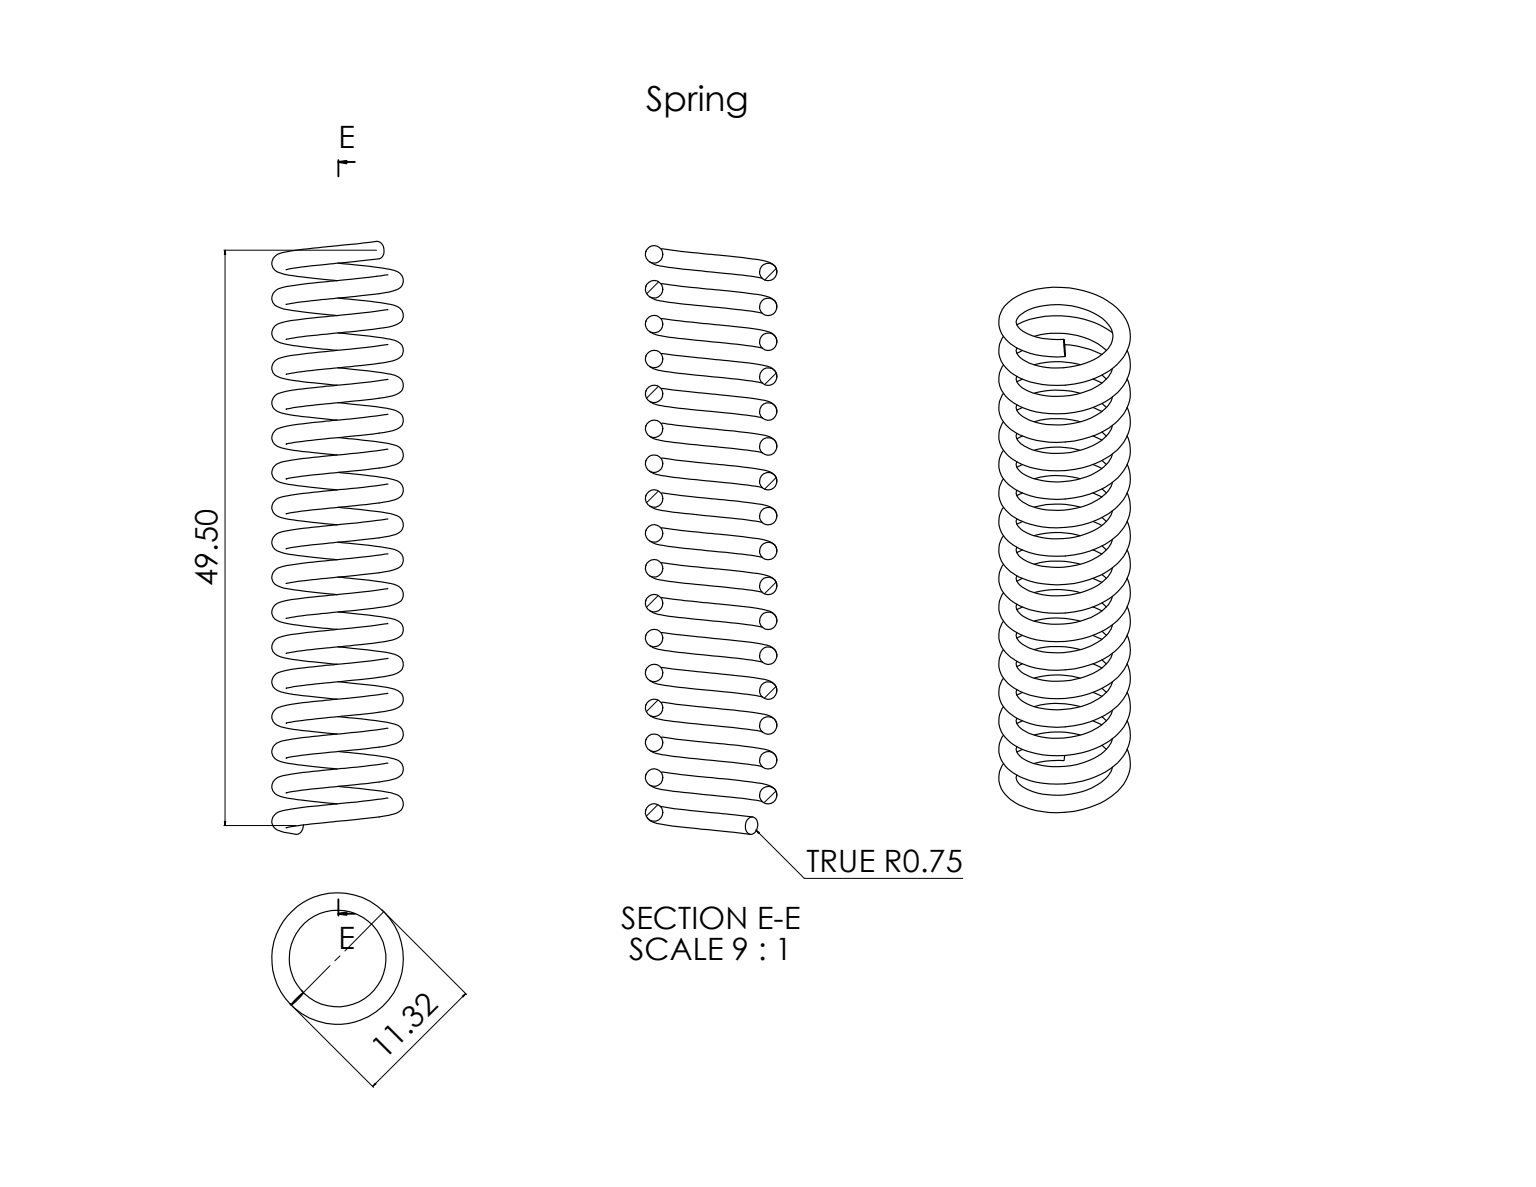
ISO-10303-21;
HEADER;
FILE_DESCRIPTION (('STEP AP214'),
    '1' );
FILE_NAME ('Spring.step',
    '2026-10-25T21:42:00',
    ( '' ),
    ( '' ),
    'SwSTEP 2.0',
    'SolidWorks 2025',
    '' );
FILE_SCHEMA (( 'AUTOMOTIVE_DESIGN' ));
ENDSEC;

DATA;
#8=CARTESIAN_POINT ( 'NONE',  ( 2.564989113914249330, 22.87042866830903876, -37.34295307432606137 ) ) ;
#27=CARTESIAN_POINT ( 'NONE',  ( -3.895814058185739448, 15.51498359085620571, -28.64999999999995950 ) ) ;
#28=CARTESIAN_POINT ( 'NONE',  ( 0.6839900399647733664, 13.18145684914961357, -55.04999999999995453 ) ) ;
#40=CARTESIAN_POINT ( 'NONE',  ( -4.099003336600151925, 21.81495595370741469, -69.75704692567386189 ) ) ;
#41=CARTESIAN_POINT ( 'NONE',  ( -0.8851648821498765418, 11.91128888458923285, -58.19999999999996732 ) ) ;
#52=CARTESIAN_POINT ( 'NONE',  ( 5.852430833189966819, 16.41846101382252243, -49.95704692567387184 ) ) ;
#56=CARTESIAN_POINT ( 'NONE',  ( 3.898383833589191383, 21.60376697729997275, -70.49295307432603863 ) ) ;
#72=CARTESIAN_POINT ( 'NONE',  ( 5.041649132594343996, 14.93115145952162415, -45.59999999999996589 ) ) ;
#75=CARTESIAN_POINT ( 'NONE',  ( 4.129897239856814117, 18.00707336630801336, -58.80704692567387326 ) ) ;
#76=CARTESIAN_POINT ( 'NONE',  ( 1.985016409143818272, 21.39581405818570659, -50.84999999999996589 ) ) ;
#85=CARTESIAN_POINT ( 'NONE',  ( 4.107178604518054499, 18.15051318458946383, -60.29999999999996163 ) ) ;
#87=CARTESIAN_POINT ( 'NONE',  ( 3.043106805520193525, 20.33772366180932067, -46.50704692567387610 ) ) ;
#91=CARTESIAN_POINT ( 'NONE',  ( -4.342430937695320736, 18.03316848959025620, -36.44295307432606279 ) ) ;
#106=CARTESIAN_POINT ( 'NONE',  ( -0.8851648821498765418, 11.91128888458923285, -49.19999999999996732 ) ) ;
#122=CARTESIAN_POINT ( 'NONE',  ( -5.876318620034919782, 18.43071743580290089, -67.94999999999994600 ) ) ;
#127=CARTESIAN_POINT ( 'NONE',  ( 4.107178604518054499, 18.15051318458946383, -42.29999999999996874 ) ) ;
#138=CARTESIAN_POINT ( 'NONE',  ( -3.826489000663265472, 15.37892550466785480, -51.14295307432606563 ) ) ;
#154=CARTESIAN_POINT ( 'NONE',  ( 4.107178604518054499, 18.15051318458946383, -33.29999999999996874 ) ) ;
#181=CARTESIAN_POINT ( 'NONE',  ( 3.965139115708213868, 19.34895832295540430, -37.65704692567386758 ) ) ;
#186=CARTESIAN_POINT ( 'NONE',  ( 4.314955953707388936, 13.40099666339979123, -38.24295307432604574 ) ) ;
#187=CARTESIAN_POINT ( 'NONE',  ( -3.705139346311794313, 19.38786279086902198, -26.09999999999996234 ) ) ;
#193=CARTESIAN_POINT ( 'NONE',  ( -1.887862790868997553, 21.20513934631180319, -44.39999999999997016 ) ) ;
#196=CARTESIAN_POINT ( 'NONE',  ( -1.028604700431329233, 11.93400751992799513, -41.70704692567387184 ) ) ;
#198=CARTESIAN_POINT ( 'NONE',  ( 3.705139346311793869, 15.61213720913094960, -63.59999999999995879 ) ) ;
#211=CARTESIAN_POINT ( 'NONE',  ( -0.7417250638684240727, 11.88857024925047057, -35.69295307432606279 ) ) ;
#233=CARTESIAN_POINT ( 'NONE',  ( 3.091735541773220852, 14.40826445822673563, -57.74999999999995737 ) ) ;
#243=CARTESIAN_POINT ( 'NONE',  ( -1.028604700431329233, 11.93400751992799513, -68.70704692567387895 ) ) ;
#244=CARTESIAN_POINT ( 'NONE',  ( 5.301103610786608300, 20.20104720010254340, -60.14999999999996305 ) ) ;
#258=CARTESIAN_POINT ( 'NONE',  ( -4.099003336600151925, 21.81495595370741469, -48.75704692567386189 ) ) ;
#264=CARTESIAN_POINT ( 'NONE',  ( -2.698247469942396837, 22.47571708489507358, -63.89295307432605853 ) ) ;
#279=CARTESIAN_POINT ( 'NONE',  ( -5.588711115410763597, 16.61483511785016987, -43.79999999999996163 ) ) ;
#282=CARTESIAN_POINT ( 'NONE',  ( -4.129897239856814117, 16.99292663369196177, -48.30704692567388037 ) ) ;
#284=CARTESIAN_POINT ( 'NONE',  ( -1.985016409143819605, 13.60418594181426855, -52.34999999999995879 ) ) ;
#294=CARTESIAN_POINT ( 'NONE',  ( 2.940415233664778416, 20.44041523366473712, -59.99999999999997158 ) ) ;
#297=CARTESIAN_POINT ( 'NONE',  ( -0.7939530028709754772, 13.41554003082070246, -47.70704692567387184 ) ) ;
#301=CARTESIAN_POINT ( 'NONE',  ( 2.017261720333081598, 13.86079270138745834, -35.39295307432605142 ) ) ;
#307=CARTESIAN_POINT ( 'NONE',  ( 3.965139115708213868, 19.34895832295540430, -28.65704692567387468 ) ) ;
#316=CARTESIAN_POINT ( 'NONE',  ( 2.701047200102605572, 22.80110361078655856, -44.84999999999996589 ) ) ;
#332=CARTESIAN_POINT ( 'NONE',  ( -2.701047200102606016, 12.19889638921340413, -70.34999999999993747 ) ) ;
#337=CARTESIAN_POINT ( 'NONE',  ( 3.895814058185739448, 19.48501640914375344, -45.14999999999994884 ) ) ;
#351=CARTESIAN_POINT ( 'NONE',  ( -0.5070733663080690956, 13.37010276014318144, -41.69295307432606279 ) ) ;
#356=CARTESIAN_POINT ( 'NONE',  ( 2.017261720333081598, 13.86079270138745834, -65.39295307432605853 ) ) ;
#368=CARTESIAN_POINT ( 'NONE',  ( -4.318543150850367773, 18.18399003996480801, -25.94999999999996732 ) ) ;
#377=CARTESIAN_POINT ( 'NONE',  ( -1.028604700431329233, 11.93400751992799513, -29.70704692567387184 ) ) ;
#395=CARTESIAN_POINT ( 'NONE',  ( 2.983759233219601459, 14.30028814967311668, -35.25704692567386900 ) ) ;
#400=CARTESIAN_POINT ( 'NONE',  ( 1.081538986177402295, 11.64756916681001186, -29.54295307432605355 ) ) ;
#401=CARTESIAN_POINT ( 'NONE',  ( -0.7939530028709754772, 13.41554003082070246, -68.70704692567387895 ) ) ;
#408=CARTESIAN_POINT ( 'NONE',  ( 0.6505131845895220088, 21.60717860451803674, -44.69999999999996021 ) ) ;
#411=CARTESIAN_POINT ( 'NONE',  ( 2.439449611014226971, 12.39241881970633230, -26.40704692567387823 ) ) ;
#413=CARTESIAN_POINT ( 'NONE',  ( 3.705139346311793869, 15.61213720913094960, -60.59999999999996589 ) ) ;
#424=CARTESIAN_POINT ( 'NONE',  ( 3.898383833589191383, 21.60376697729997275, -34.49295307432605995 ) ) ;
#445=CARTESIAN_POINT ( 'NONE',  ( 4.107178604518054499, 18.15051318458946383, -45.29999999999996874 ) ) ;
#453=CARTESIAN_POINT ( 'NONE',  ( -2.837723661809363751, 14.45689319447982335, -29.99295307432605640 ) ) ;
#455=CARTESIAN_POINT ( 'NONE',  ( -4.975717084895059372, 20.19824746994243370, -66.60704692567387042 ) ) ;
#456=CARTESIAN_POINT ( 'NONE',  ( -4.001075405444606936, 13.49892459455542060, -46.49999999999997158 ) ) ;
#469=CARTESIAN_POINT ( 'NONE',  ( -5.370428668309080500, 14.93501088608579153, -42.15704692567387468 ) ) ;
#475=CARTESIAN_POINT ( 'NONE',  ( -5.107581180293630396, 19.93944961101426827, -63.59295307432605426 ) ) ;
#491=CARTESIAN_POINT ( 'NONE',  ( -0.8851648821498765418, 11.91128888458923285, -34.19999999999996732 ) ) ;
#494=CARTESIAN_POINT ( 'NONE',  ( 3.043106805520193525, 20.33772366180932067, -49.50704692567387610 ) ) ;
#495=CARTESIAN_POINT ( 'NONE',  ( 3.091735541773220852, 14.40826445822673740, -45.74999999999995737 ) ) ;
#503=CARTESIAN_POINT ( 'NONE',  ( 4.107178604518054499, 18.15051318458946383, -57.29999999999996874 ) ) ;
#505=CARTESIAN_POINT ( 'NONE',  ( -3.639207298612509689, 19.51726172033310647, -48.60704692567386331 ) ) ;
#509=CARTESIAN_POINT ( 'NONE',  ( 0.8348115903393232839, 13.20534463599456387, -35.54295307432605711 ) ) ;
#516=CARTESIAN_POINT ( 'NONE',  ( 4.129897239856814117, 18.00707336630801336, -28.80704692567387326 ) ) ;
#523=CARTESIAN_POINT ( 'NONE',  ( 5.588711115410763597, 18.38516488214980882, -36.29999999999996163 ) ) ;
#543=CARTESIAN_POINT ( 'NONE',  ( -5.588711115410763597, 16.61483511785016987, -67.79999999999996874 ) ) ;
#548=CARTESIAN_POINT ( 'NONE',  ( -1.887862790868997553, 21.20513934631180319, -35.39999999999996305 ) ) ;
#549=CARTESIAN_POINT ( 'NONE',  ( -2.940415233664778860, 14.55958476633523802, -73.49999999999997158 ) ) ;
#560=CARTESIAN_POINT ( 'NONE',  ( 3.199711850326839357, 14.51624076678035635, -44.24295307432605995 ) ) ;
#565=CARTESIAN_POINT ( 'NONE',  ( -2.017261720333081598, 21.13920729861251857, -66.89295307432607274 ) ) ;
#575=CARTESIAN_POINT ( 'NONE',  ( -0.6839900399647736995, 21.81854315085035623, -26.54999999999996163 ) ) ;
#584=CARTESIAN_POINT ( 'NONE',  ( 5.301103610786608300, 20.20104720010253985, -63.14999999999997016 ) ) ;
#598=CARTESIAN_POINT ( 'NONE',  ( 4.314955953707388936, 13.40099666339979123, -62.24295307432607416 ) ) ;
#603=CARTESIAN_POINT ( 'NONE',  ( 4.129897239856814117, 18.00707336630801336, -31.80704692567387326 ) ) ;
#607=CARTESIAN_POINT ( 'NONE',  ( -2.837723661809363751, 14.45689319447982335, -74.99295307432603863 ) ) ;
#608=CARTESIAN_POINT ( 'NONE',  ( 4.294655364005415699, 16.66518840966061887, -64.95704692567387895 ) ) ;
#615=CARTESIAN_POINT ( 'NONE',  ( 0.6839900399647733664, 13.18145684914961357, -40.04999999999994742 ) ) ;
#618=CARTESIAN_POINT ( 'NONE',  ( -5.852430833189966819, 18.58153898617744915, -27.45704692567386829 ) ) ;
#620=CARTESIAN_POINT ( 'NONE',  ( 4.107178604518054499, 18.15051318458946383, -57.29999999999996874 ) ) ;
#633=( GEOMETRIC_REPRESENTATION_CONTEXT ( 3 ) GLOBAL_UNCERTAINTY_ASSIGNED_CONTEXT ( ( #768 ) ) GLOBAL_UNIT_ASSIGNED_CONTEXT ( ( #32119, #6174, #22541 ) ) REPRESENTATION_CONTEXT ( 'NONE', 'WORKASPACE' ) );
#635=CARTESIAN_POINT ( 'NONE',  ( -0.7417250638684240727, 11.88857024925047057, -29.69295307432606279 ) ) ;
#655=CARTESIAN_POINT ( 'NONE',  ( -4.318543150850367773, 18.18399003996480801, -43.94999999999995310 ) ) ;
#665=CARTESIAN_POINT ( 'NONE',  ( 0.6839900399647733664, 13.18145684914961357, -73.04999999999998295 ) ) ;
#667=CARTESIAN_POINT ( 'NONE',  ( -0.7798958854283041253, 23.40020640687986386, -58.05704692567386616 ) ) ;
#668=CARTESIAN_POINT ( 'NONE',  ( -5.041649132594344884, 20.06884854047834921, -44.09999999999996589 ) ) ;
#682=CARTESIAN_POINT ( 'NONE',  ( -1.028604700431329233, 11.93400751992799513, -41.70704692567387184 ) ) ;
#690=CARTESIAN_POINT ( 'NONE',  ( 5.565992480072003978, 18.52860470043125574, -58.79295307432606421 ) ) ;
#705=CARTESIAN_POINT ( 'NONE',  ( 4.206979645153767322, 13.29302035484617051, -30.74999999999995737 ) ) ;
#708=CARTESIAN_POINT ( 'NONE',  ( -3.639207298612509689, 19.51726172033310647, -54.60704692567387752 ) ) ;
#709=CARTESIAN_POINT ( 'NONE',  ( 3.705139346311793869, 15.61213720913094960, -36.59999999999996589 ) ) ;
#718=CARTESIAN_POINT ( 'NONE',  ( -1.985016409143819605, 13.60418594181426855, -52.34999999999994458 ) ) ;
#721=CARTESIAN_POINT ( 'NONE',  ( 0.5331684895902240040, 13.15756906230466328, -32.55704692567387326 ) ) ;
#725=CARTESIAN_POINT ( 'NONE',  ( -2.017261720333081598, 21.13920729861251857, -39.89295307432605853 ) ) ;
#733=CARTESIAN_POINT ( 'NONE',  ( 0.5331684895902240040, 13.15756906230466328, -26.55704692567386971 ) ) ;
#741=CARTESIAN_POINT ( 'NONE',  ( -5.301103610786608300, 14.79895279989743706, -40.64999999999994174 ) ) ;
#759=CARTESIAN_POINT ( 'NONE',  ( -5.301103610786608300, 14.79895279989743706, -58.64999999999997016 ) ) ;
#764=CARTESIAN_POINT ( 'NONE',  ( 4.318543150850367773, 16.81600996003516357, -33.44999999999994600 ) ) ;
#765=CARTESIAN_POINT ( 'NONE',  ( -1.985016409143819605, 13.60418594181426855, -64.34999999999996589 ) ) ;
#768=UNCERTAINTY_MEASURE_WITH_UNIT (LENGTH_MEASURE( 1.000000000000000082E-05 ), #32119, 'distance_accuracy_value', 'NONE');
#778=CARTESIAN_POINT ( 'NONE',  ( -0.8348115903393239501, 21.79465536400541126, -43.04295307432605711 ) ) ;
#784=CARTESIAN_POINT ( 'NONE',  ( -2.837723661809363751, 14.45689319447982335, -62.99295307432606705 ) ) ;
#796=CARTESIAN_POINT ( 'NONE',  ( 2.940415233664778416, 20.44041523366473712, -29.99999999999996447 ) ) ;
#804=CARTESIAN_POINT ( 'NONE',  ( 2.568848540478311460, 12.45835086740561692, -63.89999999999997016 ) ) ;
#821=CARTESIAN_POINT ( 'NONE',  ( -0.7417250638684240727, 11.88857024925047057, -68.69295307432605568 ) ) ;
#829=CARTESIAN_POINT ( 'NONE',  ( 1.848958322955461808, 21.46513911570817612, -76.34295307432604716 ) ) ;
#830=CARTESIAN_POINT ( 'NONE',  ( -0.7939530028709754772, 13.41554003082070246, -62.70704692567387184 ) ) ;
#842=CARTESIAN_POINT ( 'NONE',  ( -2.837105286290963146, 12.26822144673588255, -26.85704692567387397 ) ) ;
#844=CARTESIAN_POINT ( 'NONE',  ( -3.895814058185739448, 15.51498359085620571, -58.64999999999997016 ) ) ;
#857=CARTESIAN_POINT ( 'NONE',  ( -3.898383833589191827, 13.39623302270000771, -29.99295307432605640 ) ) ;
#876=CARTESIAN_POINT ( 'NONE',  ( -0.6839900399647736995, 21.81854315085035623, -44.54999999999994742 ) ) ;
#885=CARTESIAN_POINT ( 'NONE',  ( 4.107178604518054499, 18.15051318458946383, -66.29999999999996874 ) ) ;
#887=CARTESIAN_POINT ( 'NONE',  ( 1.028604700431328567, 23.06599248007198355, -61.20704692567387184 ) ) ;
#888=CARTESIAN_POINT ( 'NONE',  ( -4.206979645153769098, 21.70697964515380107, -41.24999999999995737 ) ) ;
#901=CARTESIAN_POINT ( 'NONE',  ( -0.7798958854283041253, 23.40020640687986386, -43.05704692567387326 ) ) ;
#906=CARTESIAN_POINT ( 'NONE',  ( 2.698247469942395949, 12.52428291510489977, -56.39295307432605853 ) ) ;
#924=CARTESIAN_POINT ( 'NONE',  ( 5.301103610786608300, 20.20104720010253985, -33.14999999999996305 ) ) ;
#927=CARTESIAN_POINT ( 'NONE',  ( 3.639207298612508801, 15.48273827966686866, -53.10704692567387752 ) ) ;
#938=CARTESIAN_POINT ( 'NONE',  ( 3.705139346311793869, 15.61213720913094960, -57.59999999999997300 ) ) ;
#940=CARTESIAN_POINT ( 'NONE',  ( -2.983759233219601903, 20.69971185032686023, -36.75704692567386900 ) ) ;
#941=CARTESIAN_POINT ( 'NONE',  ( -2.568848540478311904, 22.54164913259435465, -74.39999999999996305 ) ) ;
#944=CARTESIAN_POINT ( 'NONE',  ( -1.848958322955462474, 13.53486088429179546, -32.84295307432606137 ) ) ;
#952=CARTESIAN_POINT ( 'NONE',  ( 3.043106805520193525, 20.33772366180932067, -25.50704692567387610 ) ) ;
#958=CARTESIAN_POINT ( 'NONE',  ( 4.001075405444606048, 21.50107540544455276, -38.99999999999996447 ) ) ;
#976=CARTESIAN_POINT ( 'NONE',  ( -4.001075405444606936, 13.49892459455542060, -61.49999999999997158 ) ) ;
#981=CARTESIAN_POINT ( 'NONE',  ( 0.6505131845895220088, 21.60717860451803674, -35.69999999999996732 ) ) ;
#982=CARTESIAN_POINT ( 'NONE',  ( -2.940415233664778860, 14.55958476633523802, -64.49999999999997158 ) ) ;
#995=CARTESIAN_POINT ( 'NONE',  ( 3.199711850326839357, 14.51624076678035635, -41.24295307432605284 ) ) ;
#1000=CARTESIAN_POINT ( 'NONE',  ( -3.771071394011080269, 19.25846386140493394, -60.59295307432606847 ) ) ;
#1011=CARTESIAN_POINT ( 'NONE',  ( 1.887862790868997109, 13.79486065368817194, -30.89999999999996305 ) ) ;
#1020=CARTESIAN_POINT ( 'NONE',  ( 4.206979645153767322, 13.29302035484617051, -66.74999999999997158 ) ) ;
#1038=CARTESIAN_POINT ( 'NONE',  ( 4.314955953707388936, 13.40099666339979123, -59.24295307432605995 ) ) ;
#1047=CARTESIAN_POINT ( 'NONE',  ( -3.771071394011080269, 19.25846386140493394, -72.59295307432606137 ) ) ;
#1049=CARTESIAN_POINT ( 'NONE',  ( -2.983759233219601903, 20.69971185032686023, -60.75704692567388321 ) ) ;
#1059=CARTESIAN_POINT ( 'NONE',  ( -2.439449611014227859, 22.60758118029364283, -27.90704692567387823 ) ) ;
#1061=CARTESIAN_POINT ( 'NONE',  ( 3.091735541773220852, 14.40826445822673563, -54.74999999999997158 ) ) ;
#1076=CARTESIAN_POINT ( 'NONE',  ( -5.900206406879871857, 18.27989588542834554, -30.44295307432605213 ) ) ;
#1095=CARTESIAN_POINT ( 'NONE',  ( 3.091735541773220852, 14.40826445822673563, -45.74999999999995737 ) ) ;
#1103=CARTESIAN_POINT ( 'NONE',  ( 3.895814058185739448, 19.48501640914375344, -63.14999999999997016 ) ) ;
#1105=CARTESIAN_POINT ( 'NONE',  ( -1.028604700431329233, 11.93400751992799513, -53.70704692567388605 ) ) ;
#1106=CARTESIAN_POINT ( 'NONE',  ( 5.876318620034919782, 16.56928256419707068, -45.44999999999996021 ) ) ;
#1118=CARTESIAN_POINT ( 'NONE',  ( -1.028604700431329233, 11.93400751992799513, -35.70704692567387184 ) ) ;
#1122=CARTESIAN_POINT ( 'NONE',  ( 2.564989113914249330, 22.87042866830903876, -58.34295307432606137 ) ) ;
#1137=CARTESIAN_POINT ( 'NONE',  ( -4.001075405444606936, 13.49892459455542060, -28.49999999999996447 ) ) ;
#1140=CARTESIAN_POINT ( 'NONE',  ( -1.758463861404912842, 21.27107139401109137, -54.90704692567386758 ) ) ;
#1142=CARTESIAN_POINT ( 'NONE',  ( 1.887862790868997109, 13.79486065368817194, -72.89999999999996305 ) ) ;
#1150=CARTESIAN_POINT ( 'NONE',  ( -4.318543150850367773, 18.18399003996480801, -58.94999999999995310 ) ) ;
#1152=CARTESIAN_POINT ( 'NONE',  ( -4.294655364005415699, 18.33481159033935626, -39.45704692567387184 ) ) ;
#1162=CARTESIAN_POINT ( 'NONE',  ( -4.099003336600151925, 21.81495595370741469, -69.75704692567386189 ) ) ;
#1167=CARTESIAN_POINT ( 'NONE',  ( -5.588711115410763597, 16.61483511785016987, -37.79999999999996874 ) ) ;
#1182=CARTESIAN_POINT ( 'NONE',  ( -2.701047200102606016, 12.19889638921340413, -61.34999999999996589 ) ) ;
#1187=CARTESIAN_POINT ( 'NONE',  ( -0.6505131845895224529, 13.39282139548194195, -31.19999999999996376 ) ) ;
#1188=CARTESIAN_POINT ( 'NONE',  ( -3.895814058185739892, 15.51498359085620748, -67.64999999999997726 ) ) ;
#1202=CARTESIAN_POINT ( 'NONE',  ( -0.8348115903393239501, 21.79465536400541126, -46.04295307432605711 ) ) ;
#1207=CARTESIAN_POINT ( 'NONE',  ( -3.199711850326840246, 20.48375923321962233, -63.74295307432605995 ) ) ;
#1225=CARTESIAN_POINT ( 'NONE',  ( 5.876318620034919782, 16.56928256419707068, -66.44999999999997442 ) ) ;
#1245=CARTESIAN_POINT ( 'NONE',  ( 1.081538986177402295, 11.64756916681001186, -59.54295307432605711 ) ) ;
#1253=CARTESIAN_POINT ( 'NONE',  ( 2.837723661809363307, 20.54310680552015356, -70.49295307432603863 ) ) ;
#1255=CARTESIAN_POINT ( 'NONE',  ( -4.129897239856814117, 16.99292663369196177, -63.30704692567387326 ) ) ;
#1270=CARTESIAN_POINT ( 'NONE',  ( 4.975717084895059372, 14.80175253005754143, -32.10704692567387042 ) ) ;
#1271=CARTESIAN_POINT ( 'NONE',  ( 3.091735541773220852, 14.40826445822673563, -57.74999999999995737 ) ) ;
#1282=CARTESIAN_POINT ( 'NONE',  ( 0.8348115903393232839, 13.20534463599456387, -71.54295307432605000 ) ) ;
#1299=CARTESIAN_POINT ( 'NONE',  ( -0.6839900399647736995, 21.81854315085035623, -47.54999999999997584 ) ) ;
#1308=CARTESIAN_POINT ( 'NONE',  ( 1.887862790868997109, 13.79486065368817194, -69.89999999999996305 ) ) ;
#1310=CARTESIAN_POINT ( 'NONE',  ( 4.103766977300021601, 21.39838383358913987, -58.50704692567387610 ) ) ;
#1311=CARTESIAN_POINT ( 'NONE',  ( 5.041649132594343996, 14.93115145952162415, -48.59999999999996589 ) ) ;
#1326=CARTESIAN_POINT ( 'NONE',  ( -5.611429750749524992, 16.75827493613162034, -36.30704692567387326 ) ) ;
#1330=CARTESIAN_POINT ( 'NONE',  ( 4.314955953707388936, 13.40099666339979123, -47.24295307432605995 ) ) ;
#1345=CARTESIAN_POINT ( 'NONE',  ( 0.9307174358028528216, 11.62368137996505801, -31.04999999999995808 ) ) ;
#1348=CARTESIAN_POINT ( 'NONE',  ( 3.043106805520193525, 20.33772366180932067, -46.50704692567387610 ) ) ;
#1349=CARTESIAN_POINT ( 'NONE',  ( 0.6839900399647733664, 13.18145684914961357, -73.04999999999998295 ) ) ;
#1356=CARTESIAN_POINT ( 'NONE',  ( -1.887862790868997553, 21.20513934631180319, -53.39999999999997016 ) ) ;
#1358=CARTESIAN_POINT ( 'NONE',  ( -1.758463861404912842, 21.27107139401109137, -36.90704692567386758 ) ) ;
#1369=CARTESIAN_POINT ( 'NONE',  ( 4.099003336600150149, 13.18504404629255689, -68.25704692567387610 ) ) ;
#1373=CARTESIAN_POINT ( 'NONE',  ( -5.301103610786608300, 14.79895279989743706, -37.64999999999996305 ) ) ;
#1391=CARTESIAN_POINT ( 'NONE',  ( 5.301103610786608300, 20.20104720010253985, -60.14999999999995595 ) ) ;
#1396=CARTESIAN_POINT ( 'NONE',  ( -3.705139346311794313, 19.38786279086902198, -29.09999999999996589 ) ) ;
#1397=CARTESIAN_POINT ( 'NONE',  ( -1.887862790868997553, 21.20513934631180319, -71.39999999999996305 ) ) ;
#1408=CARTESIAN_POINT ( 'NONE',  ( 2.017261720333081598, 13.86079270138745834, -32.39295307432605142 ) ) ;
#1413=CARTESIAN_POINT ( 'NONE',  ( -4.342430937695320736, 18.03316848959025620, -51.44295307432605568 ) ) ;
#1430=CARTESIAN_POINT ( 'NONE',  ( 4.001075405444606048, 21.50107540544455276, -65.99999999999997158 ) ) ;
#1453=CARTESIAN_POINT ( 'NONE',  ( 5.231778553264135212, 20.33710528629089254, -58.64295307432606563 ) ) ;
#1461=CARTESIAN_POINT ( 'NONE',  ( 2.837723661809363307, 20.54310680552015356, -61.49295307432606705 ) ) ;
#1463=CARTESIAN_POINT ( 'NONE',  ( -3.043106805520194413, 14.66227633819065623, -54.00704692567387610 ) ) ;
#1475=CARTESIAN_POINT ( 'NONE',  ( 1.985016409143818272, 21.39581405818570303, -53.84999999999995879 ) ) ;
#1485=CARTESIAN_POINT ( 'NONE',  ( 0.5070733663080689846, 21.62989723985679902, -70.19295307432605568 ) ) ;
#1499=CARTESIAN_POINT ( 'NONE',  ( -1.985016409143819605, 13.60418594181426855, -40.34999999999996589 ) ) ;
#1505=CARTESIAN_POINT ( 'NONE',  ( -4.107178604518053611, 16.84948681541050775, -31.79999999999996874 ) ) ;
#1515=CARTESIAN_POINT ( 'NONE',  ( 2.940415233664778416, 20.44041523366473712, -62.99999999999997158 ) ) ;
#1518=CARTESIAN_POINT ( 'NONE',  ( -4.975717084895059372, 20.19824746994243370, -54.60704692567387752 ) ) ;
#1519=CARTESIAN_POINT ( 'NONE',  ( -4.206979645153769098, 21.70697964515380107, -35.24999999999997158 ) ) ;
#1532=CARTESIAN_POINT ( 'NONE',  ( -4.099003336600151925, 21.81495595370741469, -39.75704692567386900 ) ) ;
#1535=CARTESIAN_POINT ( 'NONE',  ( -4.314955953707389824, 21.59900333660018390, -54.74295307432605995 ) ) ;
#1553=CARTESIAN_POINT ( 'NONE',  ( 0.8851648821498760977, 23.08871111541074228, -26.69999999999996732 ) ) ;
#1557=CARTESIAN_POINT ( 'NONE',  ( 3.965139115708213868, 19.34895832295540430, -43.65704692567387468 ) ) ;
#1567=CARTESIAN_POINT ( 'NONE',  ( 0.6839900399647733664, 13.18145684914961357, -49.04999999999994742 ) ) ;
#1570=CARTESIAN_POINT ( 'NONE',  ( -4.129897239856814117, 16.99292663369196177, -36.30704692567387326 ) ) ;
#1571=CARTESIAN_POINT ( 'NONE',  ( 5.041649132594343996, 14.93115145952162415, -72.59999999999996589 ) ) ;
#1581=CARTESIAN_POINT ( 'NONE',  ( 4.099003336600150149, 13.18504404629255689, -62.25704692567386900 ) ) ;
#1585=CARTESIAN_POINT ( 'NONE',  ( -5.876318620034919782, 18.43071743580290089, -31.94999999999994955 ) ) ;
#1600=CARTESIAN_POINT ( 'NONE',  ( -5.588711115410763597, 16.61483511785016987, -58.79999999999996163 ) ) ;
#1605=CARTESIAN_POINT ( 'NONE',  ( 3.043106805520193525, 20.33772366180932067, -73.50704692567386189 ) ) ;
#1606=CARTESIAN_POINT ( 'NONE',  ( 0.6839900399647732554, 13.18145684914961357, -64.04999999999995453 ) ) ;
#1613=CARTESIAN_POINT ( 'NONE',  ( 3.705139346311793869, 15.61213720913094960, -69.59999999999996589 ) ) ;
#1617=CARTESIAN_POINT ( 'NONE',  ( -2.017261720333081598, 21.13920729861251857, -39.89295307432605853 ) ) ;
#1620=CARTESIAN_POINT ( 'NONE',  ( 0.5070733663080689846, 21.62989723985679902, -52.19295307432606279 ) ) ;
#1634=CARTESIAN_POINT ( 'NONE',  ( -4.206979645153768210, 21.70697964515380107, -53.24999999999996447 ) ) ;
#1654=CARTESIAN_POINT ( 'NONE',  ( 5.565992480072003978, 18.52860470043125574, -58.79295307432606421 ) ) ;
#1663=CARTESIAN_POINT ( 'NONE',  ( 2.837723661809363307, 20.54310680552015356, -64.49295307432606705 ) ) ;
#1666=CARTESIAN_POINT ( 'NONE',  ( 2.983759233219601459, 14.30028814967311668, -59.25704692567388321 ) ) ;
#1680=CARTESIAN_POINT ( 'NONE',  ( -0.6839900399647736995, 21.81854315085035623, -50.54999999999996163 ) ) ;
#1691=CARTESIAN_POINT ( 'NONE',  ( -1.848958322955462474, 13.53486088429179546, -74.84295307432606137 ) ) ;
#1707=CARTESIAN_POINT ( 'NONE',  ( 2.940415233664778416, 20.44041523366473712, -38.99999999999996447 ) ) ;
#1711=CARTESIAN_POINT ( 'NONE',  ( -0.6839900399647736995, 21.81854315085035623, -32.54999999999996163 ) ) ;
#1722=CARTESIAN_POINT ( 'NONE',  ( -1.985016409143819605, 13.60418594181426855, -52.34999999999994458 ) ) ;
#1724=CARTESIAN_POINT ( 'NONE',  ( -5.611429750749524992, 16.75827493613162034, -51.30704692567388037 ) ) ;
#1725=CARTESIAN_POINT ( 'NONE',  ( -5.301103610786608300, 14.79895279989743528, -34.64999999999997016 ) ) ;
#1728=CARTESIAN_POINT ( 'NONE',  ( 3.091735541773220852, 14.40826445822673563, -72.74999999999995737 ) ) ;
#1740=CARTESIAN_POINT ( 'NONE',  ( -2.837105286290963146, 12.26822144673588255, -35.85704692567387752 ) ) ;
#1743=CARTESIAN_POINT ( 'NONE',  ( 2.698247469942395949, 12.52428291510489977, -53.39295307432605853 ) ) ;
#1761=CARTESIAN_POINT ( 'NONE',  ( 3.898383833589191383, 21.60376697729997275, -76.49295307432603863 ) ) ;
#1764=CARTESIAN_POINT ( 'NONE',  ( -4.129897239856814117, 16.99292663369196177, -45.30704692567388037 ) ) ;
#1765=CARTESIAN_POINT ( 'NONE',  ( 4.318543150850367773, 16.81600996003516357, -39.44999999999994600 ) ) ;
#1766=CARTESIAN_POINT ( 'NONE',  ( 1.985016409143818272, 21.39581405818570303, -68.84999999999996589 ) ) ;
#1775=CARTESIAN_POINT ( 'NONE',  ( -4.129897239856814117, 16.99292663369196177, -30.30704692567387326 ) ) ;
#1776=CARTESIAN_POINT ( 'NONE',  ( -4.001075405444606936, 13.49892459455542060, -64.49999999999997158 ) ) ;
#1786=CARTESIAN_POINT ( 'NONE',  ( 5.370428668309080500, 20.06498911391418360, -61.65704692567387468 ) ) ;
#1790=CARTESIAN_POINT ( 'NONE',  ( -2.701047200102606016, 12.19889638921340413, -28.34999999999995524 ) ) ;
#1806=CARTESIAN_POINT ( 'NONE',  ( 5.588711115410763597, 18.38516488214980882, -54.29999999999996874 ) ) ;
#1810=CARTESIAN_POINT ( 'NONE',  ( -0.5331684895902242260, 21.84243093769531185, -73.05704692567387326 ) ) ;
#1811=CARTESIAN_POINT ( 'NONE',  ( -4.318543150850366885, 18.18399003996480801, -55.94999999999997442 ) ) ;
#1823=CARTESIAN_POINT ( 'NONE',  ( -0.8348115903393239501, 21.79465536400541126, -37.04295307432605711 ) ) ;
#1826=CARTESIAN_POINT ( 'NONE',  ( -3.771071394011080269, 19.25846386140493394, -51.59295307432605426 ) ) ;
#1840=CARTESIAN_POINT ( 'NONE',  ( -0.8851648821498765418, 11.91128888458923285, -55.19999999999997442 ) ) ;
#1860=CARTESIAN_POINT ( 'NONE',  ( 5.900206406879871857, 16.72010411457162604, -52.94295307432605568 ) ) ;
#1868=CARTESIAN_POINT ( 'NONE',  ( -4.342430937695320736, 18.03316848959025620, -63.44295307432605568 ) ) ;
#1881=CARTESIAN_POINT ( 'NONE',  ( -4.107178604518053611, 16.84948681541050775, -46.79999999999996874 ) ) ;
#1892=CARTESIAN_POINT ( 'NONE',  ( 0.5070733663080689846, 21.62989723985679902, -76.19295307432606990 ) ) ;
#1903=CARTESIAN_POINT ( 'NONE',  ( -1.887862790868997553, 21.20513934631180319, -35.39999999999996305 ) ) ;
#1908=CARTESIAN_POINT ( 'NONE',  ( -1.985016409143819605, 13.60418594181426855, -31.34999999999996945 ) ) ;
#1913=SHAPE_REPRESENTATION ( 'Spring', ( #40442 ), #33653 ) ;
#1917=CARTESIAN_POINT ( 'NONE',  ( 3.705139346311793869, 15.61213720913094960, -51.59999999999996589 ) ) ;
#1919=CARTESIAN_POINT ( 'NONE',  ( 4.975717084895059372, 14.80175253005754143, -50.10704692567387752 ) ) ;
#1920=CARTESIAN_POINT ( 'NONE',  ( 2.701047200102605128, 22.80110361078656211, -32.84999999999996589 ) ) ;
#1924=CARTESIAN_POINT ( 'NONE',  ( -3.771071394011080269, 19.25846386140493394, -27.59295307432605782 ) ) ;
#1935=CARTESIAN_POINT ( 'NONE',  ( 5.370428668309080500, 20.06498911391418360, -31.65704692567386402 ) ) ;
#1940=CARTESIAN_POINT ( 'NONE',  ( -5.231778553264134324, 14.66289471370907727, -54.14295307432606563 ) ) ;
#1957=CARTESIAN_POINT ( 'NONE',  ( -5.231778553264134324, 14.66289471370907727, -75.14295307432605853 ) ) ;
#1960=CARTESIAN_POINT ( 'NONE',  ( 0.7939530028709752552, 21.58445996917927445, -46.20704692567387184 ) ) ;
#1961=CARTESIAN_POINT ( 'NONE',  ( -3.895814058185739448, 15.51498359085620571, -31.64999999999995950 ) ) ;
#1962=CARTESIAN_POINT ( 'NONE',  ( -4.107178604518053611, 16.84948681541050775, -64.79999999999996874 ) ) ;
#1971=CARTESIAN_POINT ( 'NONE',  ( 4.294655364005415699, 16.66518840966061887, -28.95704692567387184 ) ) ;
#1972=CARTESIAN_POINT ( 'NONE',  ( -4.001075405444606936, 13.49892459455542060, -61.49999999999997158 ) ) ;
#1987=CARTESIAN_POINT ( 'NONE',  ( -1.028604700431329233, 11.93400751992799513, -68.70704692567387895 ) ) ;
#1991=CARTESIAN_POINT ( 'NONE',  ( -1.081538986177402961, 23.35243083318996327, -76.04295307432605000 ) ) ;
#2008=CARTESIAN_POINT ( 'NONE',  ( -0.9307174358028533767, 23.37631862003491889, -50.54999999999996163 ) ) ;
#2013=CARTESIAN_POINT ( 'NONE',  ( -2.940415233664778860, 14.55958476633523802, -25.49999999999996803 ) ) ;
#2014=CARTESIAN_POINT ( 'NONE',  ( -2.940415233664778860, 14.55958476633523802, -55.49999999999996447 ) ) ;
#2020=CARTESIAN_POINT ( 'NONE',  ( 2.940415233664778416, 20.44041523366473712, -74.99999999999997158 ) ) ;
#2025=CARTESIAN_POINT ( 'NONE',  ( -4.084459969179292216, 16.70604699712905372, -39.29295307432605711 ) ) ;
#2029=CARTESIAN_POINT ( 'NONE',  ( 0.5070733663080689846, 21.62989723985679902, -55.19295307432606279 ) ) ;
#2044=CARTESIAN_POINT ( 'NONE',  ( 2.568848540478311460, 12.45835086740561692, -60.89999999999997016 ) ) ;
#2065=CARTESIAN_POINT ( 'NONE',  ( 5.900206406879871857, 16.72010411457162604, -46.94295307432605568 ) ) ;
#2075=CARTESIAN_POINT ( 'NONE',  ( -1.848958322955462474, 13.53486088429179546, -68.84295307432606137 ) ) ;
#2089=CARTESIAN_POINT ( 'NONE',  ( -0.6839900399647736995, 21.81854315085035623, -44.54999999999994742 ) ) ;
#2115=CARTESIAN_POINT ( 'NONE',  ( -1.887862790868997553, 21.20513934631180319, -41.39999999999996305 ) ) ;
#2120=CARTESIAN_POINT ( 'NONE',  ( -0.6505131845895224529, 13.39282139548194195, -34.19999999999996732 ) ) ;
#2129=CARTESIAN_POINT ( 'NONE',  ( 4.318543150850367773, 16.81600996003516357, -54.44999999999996021 ) ) ;
#2131=CARTESIAN_POINT ( 'NONE',  ( 4.099003336600150149, 13.18504404629255689, -44.25704692567387610 ) ) ;
#2132=CARTESIAN_POINT ( 'NONE',  ( -5.588711115410763597, 16.61483511785016987, -34.79999999999996163 ) ) ;
#2135=CARTESIAN_POINT ( 'NONE',  ( -1.887862790868997553, 21.20513934631180319, -71.39999999999996305 ) ) ;
#2143=CARTESIAN_POINT ( 'NONE',  ( 4.099003336600150149, 13.18504404629255689, -29.25704692567387255 ) ) ;
#2147=CARTESIAN_POINT ( 'NONE',  ( -5.231778553264134324, 14.66289471370907727, -51.14295307432606563 ) ) ;
#2166=CARTESIAN_POINT ( 'NONE',  ( -2.568848540478311904, 22.54164913259435465, -26.39999999999996660 ) ) ;
#2171=CARTESIAN_POINT ( 'NONE',  ( -3.965139115708213868, 15.65104167704456906, -39.15704692567386758 ) ) ;
#2172=CARTESIAN_POINT ( 'NONE',  ( 3.895814058185739448, 19.48501640914375344, -30.14999999999997016 ) ) ;
#2174=CARTESIAN_POINT ( 'NONE',  ( 1.985016409143818272, 21.39581405818570303, -62.84999999999995879 ) ) ;
#2185=CARTESIAN_POINT ( 'NONE',  ( 0.5331684895902240040, 13.15756906230466328, -29.55704692567387681 ) ) ;
#2186=CARTESIAN_POINT ( 'NONE',  ( 0.8851648821498760977, 23.08871111541074228, -68.69999999999997442 ) ) ;
#2199=CARTESIAN_POINT ( 'NONE',  ( 0.7798958854283032371, 11.59979359312010772, -62.55704692567387326 ) ) ;
#2203=CARTESIAN_POINT ( 'NONE',  ( 4.206979645153767322, 13.29302035484617051, -27.74999999999995381 ) ) ;
#2223=CARTESIAN_POINT ( 'NONE',  ( -2.568848540478311904, 22.54164913259435465, -47.39999999999997016 ) ) ;
#2227=CARTESIAN_POINT ( 'NONE',  ( 4.107178604518054499, 18.15051318458946383, -27.29999999999996163 ) ) ;
#2228=CARTESIAN_POINT ( 'NONE',  ( 0.6839900399647732554, 13.18145684914961357, -58.04999999999996163 ) ) ;
#2239=CARTESIAN_POINT ( 'NONE',  ( -3.199711850326840246, 20.48375923321962233, -36.74295307432605995 ) ) ;
#2243=CARTESIAN_POINT ( 'NONE',  ( 4.342430937695320736, 16.96683151040971538, -58.94295307432605568 ) ) ;
#2259=CARTESIAN_POINT ( 'NONE',  ( -0.9307174358028533767, 23.37631862003491889, -56.54999999999996874 ) ) ;
#2282=CARTESIAN_POINT ( 'NONE',  ( 4.314955953707388936, 13.40099666339979123, -44.24295307432605995 ) ) ;
#2289=CARTESIAN_POINT ( 'NONE',  ( -2.837723661809363751, 14.45689319447982335, -68.99295307432605284 ) ) ;
#2303=CARTESIAN_POINT ( 'NONE',  ( 3.895814058185739448, 19.48501640914375344, -42.14999999999996305 ) ) ;
#2330=CARTESIAN_POINT ( 'NONE',  ( 3.705139346311793869, 15.61213720913094960, -30.59999999999996589 ) ) ;
#2335=CARTESIAN_POINT ( 'NONE',  ( 0.6839900399647733664, 13.18145684914961357, -37.04999999999996163 ) ) ;
#2342=EDGE_CURVE ( 'NONE', #21597, #2773, #38326, .T. ) ;
#2344=CARTESIAN_POINT ( 'NONE',  ( -3.895814058185739448, 15.51498359085620571, -55.64999999999994174 ) ) ;
#2346=CARTESIAN_POINT ( 'NONE',  ( -4.099003336600151925, 21.81495595370741469, -42.75704692567387610 ) ) ;
#2347=CARTESIAN_POINT ( 'NONE',  ( 2.568848540478311460, 12.45835086740561692, -39.89999999999996305 ) ) ;
#2349=CARTESIAN_POINT ( 'NONE',  ( 1.887862790868997109, 13.79486065368817194, -69.89999999999996305 ) ) ;
#2360=CARTESIAN_POINT ( 'NONE',  ( -2.439449611014227859, 22.60758118029364283, -27.90704692567387823 ) ) ;
#2366=CARTESIAN_POINT ( 'NONE',  ( -0.7417250638684240727, 11.88857024925047057, -38.69295307432606279 ) ) ;
#2385=CARTESIAN_POINT ( 'NONE',  ( -2.698247469942396837, 22.47571708489507358, -72.89295307432605853 ) ) ;
#2390=CARTESIAN_POINT ( 'NONE',  ( -3.091735541773221296, 20.59173554177323950, -35.24999999999997158 ) ) ;
#2391=CARTESIAN_POINT ( 'NONE',  ( -4.107178604518053611, 16.84948681541050775, -67.79999999999996874 ) ) ;
#2401=CARTESIAN_POINT ( 'NONE',  ( 3.043106805520193525, 20.33772366180932067, -28.50704692567387610 ) ) ;
#2402=CARTESIAN_POINT ( 'NONE',  ( -2.568848540478311904, 22.54164913259435465, -68.39999999999997726 ) ) ;
#2413=CARTESIAN_POINT ( 'NONE',  ( 0.7798958854283032371, 11.59979359312010772, -56.55704692567387326 ) ) ;
#2416=CARTESIAN_POINT ( 'NONE',  ( -2.698247469942396837, 22.47571708489507358, -66.89295307432607274 ) ) ;
#2435=CARTESIAN_POINT ( 'NONE',  ( -2.568848540478311904, 22.54164913259435465, -50.39999999999996305 ) ) ;
#2439=CARTESIAN_POINT ( 'NONE',  ( 3.639207298612508801, 15.48273827966686866, -71.10704692567387042 ) ) ;
#2440=CARTESIAN_POINT ( 'NONE',  ( -4.318543150850366885, 18.18399003996480801, -58.94999999999996021 ) ) ;
#2446=CARTESIAN_POINT ( 'NONE',  ( -0.6839900399647736995, 21.81854315085035623, -74.54999999999994031 ) ) ;
#2448=CARTESIAN_POINT ( 'NONE',  ( -3.965139115708213868, 15.65104167704456906, -54.15704692567387468 ) ) ;
#2451=CARTESIAN_POINT ( 'NONE',  ( -4.342430937695320736, 18.03316848959025620, -30.44295307432605213 ) ) ;
#2453=CARTESIAN_POINT ( 'NONE',  ( 3.199711850326839357, 14.51624076678035635, -44.24295307432605995 ) ) ;
#2469=CARTESIAN_POINT ( 'NONE',  ( -2.568848540478311904, 22.54164913259435465, -62.39999999999997016 ) ) ;
#2490=CARTESIAN_POINT ( 'NONE',  ( 4.314955953707388936, 13.40099666339979123, -50.24295307432605284 ) ) ;
#2498=CARTESIAN_POINT ( 'NONE',  ( -1.848958322955462474, 13.53486088429179546, -59.84295307432606137 ) ) ;
#2511=CARTESIAN_POINT ( 'NONE',  ( 3.895814058185739448, 19.48501640914375344, -45.14999999999994884 ) ) ;
#2537=CARTESIAN_POINT ( 'NONE',  ( 0.6505131845895220088, 21.60717860451803674, -26.69999999999996732 ) ) ;
#2542=CARTESIAN_POINT ( 'NONE',  ( 0.5331684895902240040, 13.15756906230466328, -71.55704692567385905 ) ) ;
#2551=CARTESIAN_POINT ( 'NONE',  ( -3.895814058185739448, 15.51498359085620571, -58.64999999999997016 ) ) ;
#2555=CARTESIAN_POINT ( 'NONE',  ( 2.837105286290961370, 22.73177855326409613, -46.35704692567385621 ) ) ;
#2557=CARTESIAN_POINT ( 'NONE',  ( -4.084459969179292216, 16.70604699712905372, -30.29295307432605355 ) ) ;
#2568=CARTESIAN_POINT ( 'NONE',  ( -0.7798958854283041253, 23.40020640687986386, -28.05704692567386971 ) ) ;
#2572=CARTESIAN_POINT ( 'NONE',  ( 5.565992480072003978, 18.52860470043125574, -43.79295307432606421 ) ) ;
#2588=CARTESIAN_POINT ( 'NONE',  ( -0.7417250638684240727, 11.88857024925047057, -59.69295307432605568 ) ) ;
#2592=CARTESIAN_POINT ( 'NONE',  ( 0.6505131845895220088, 21.60717860451803674, -38.69999999999996021 ) ) ;
#2593=CARTESIAN_POINT ( 'NONE',  ( -2.940415233664778860, 14.55958476633523802, -64.49999999999997158 ) ) ;
#2605=CARTESIAN_POINT ( 'NONE',  ( 3.639207298612508801, 15.48273827966686866, -29.10704692567387752 ) ) ;
#2606=CARTESIAN_POINT ( 'NONE',  ( 5.876318620034919782, 16.56928256419707068, -63.44999999999996732 ) ) ;
#2619=CARTESIAN_POINT ( 'NONE',  ( 4.099003336600150149, 13.18504404629255689, -53.25704692567386900 ) ) ;
#2622=CARTESIAN_POINT ( 'NONE',  ( 0.7417250638684235176, 23.11142975074950101, -73.19295307432605568 ) ) ;
#2639=CARTESIAN_POINT ( 'NONE',  ( -5.588711115410763597, 16.61483511785016987, -37.79999999999996874 ) ) ;
#2643=CARTESIAN_POINT ( 'NONE',  ( -1.758463861404912842, 21.27107139401109137, -63.90704692567388179 ) ) ;
#2644=CARTESIAN_POINT ( 'NONE',  ( -3.705139346311794313, 19.38786279086902198, -56.09999999999996589 ) ) ;
#2651=CARTESIAN_POINT ( 'NONE',  ( -0.6505131845895224529, 13.39282139548194195, -64.19999999999996021 ) ) ;
#2654=CARTESIAN_POINT ( 'NONE',  ( 3.639207298612508801, 15.48273827966686866, -59.10704692567387752 ) ) ;
#2657=CARTESIAN_POINT ( 'NONE',  ( -2.940415233664778860, 14.55958476633523802, -70.49999999999997158 ) ) ;
#2660=CARTESIAN_POINT ( 'NONE',  ( -3.199711850326840246, 20.48375923321962233, -42.74295307432605284 ) ) ;
#2677=CARTESIAN_POINT ( 'NONE',  ( -4.001075405444606936, 13.49892459455542060, -52.49999999999996447 ) ) ;
#2695=CARTESIAN_POINT ( 'NONE',  ( 0.6505131845895220088, 21.60717860451803674, -38.69999999999996021 ) ) ;
#2697=CARTESIAN_POINT ( 'NONE',  ( 2.698247469942395949, 12.52428291510489977, -47.39295307432605853 ) ) ;
#2707=CARTESIAN_POINT ( 'NONE',  ( -0.5070733663080690956, 13.37010276014318144, -56.69295307432606279 ) ) ;
#2722=CARTESIAN_POINT ( 'NONE',  ( 1.985016409143818272, 21.39581405818570303, -38.84999999999996589 ) ) ;
#2748=CARTESIAN_POINT ( 'NONE',  ( 2.940415233664778416, 20.44041523366473712, -26.99999999999996803 ) ) ;
#2751=CARTESIAN_POINT ( 'NONE',  ( -4.314955953707389824, 21.59900333660018390, -33.74295307432605995 ) ) ;
#2752=CARTESIAN_POINT ( 'NONE',  ( 3.895814058185739448, 19.48501640914375344, -30.14999999999997016 ) ) ;
#2760=CARTESIAN_POINT ( 'NONE',  ( 0.6505131845895220088, 21.60717860451803674, -50.69999999999996732 ) ) ;
#2763=CARTESIAN_POINT ( 'NONE',  ( -2.837105286290963146, 12.26822144673588255, -35.85704692567387752 ) ) ;
#2765=CARTESIAN_POINT ( 'NONE',  ( -2.940415233664778860, 14.55958476633523802, -67.49999999999995737 ) ) ;
#2773=VERTEX_POINT ( 'NONE', #34406 ) ;
#2777=CARTESIAN_POINT ( 'NONE',  ( -5.041649132594344884, 20.06884854047834921, -74.09999999999996589 ) ) ;
#2783=CARTESIAN_POINT ( 'NONE',  ( -5.565992480072003978, 16.47139529956871229, -42.29295307432605711 ) ) ;
#2803=CARTESIAN_POINT ( 'NONE',  ( 1.081538986177402295, 11.64756916681001186, -65.54295307432606421 ) ) ;
#2808=CARTESIAN_POINT ( 'NONE',  ( 3.895814058185739448, 19.48501640914375344, -27.14999999999995595 ) ) ;
#2809=CARTESIAN_POINT ( 'NONE',  ( -3.091735541773221296, 20.59173554177323950, -56.24999999999995026 ) ) ;
#2819=CARTESIAN_POINT ( 'NONE',  ( 4.975717084895059372, 14.80175253005754143, -62.10704692567388463 ) ) ;
#2820=CARTESIAN_POINT ( 'NONE',  ( 4.206979645153768210, 13.29302035484617406, -54.74999999999996447 ) ) ;
#2831=CARTESIAN_POINT ( 'NONE',  ( 4.103766977300021601, 21.39838383358913987, -58.50704692567387610 ) ) ;
#2835=CARTESIAN_POINT ( 'NONE',  ( 4.314955953707388936, 13.40099666339979123, -74.24295307432606705 ) ) ;
#2851=CARTESIAN_POINT ( 'NONE',  ( 5.301103610786608300, 20.20104720010253985, -39.14999999999997016 ) ) ;
#2855=CARTESIAN_POINT ( 'NONE',  ( 4.129897239856814117, 18.00707336630801336, -64.80704692567387326 ) ) ;
#2856=CARTESIAN_POINT ( 'NONE',  ( 3.705139346311793869, 15.61213720913094960, -51.59999999999996589 ) ) ;
#2865=CARTESIAN_POINT ( 'NONE',  ( 1.887862790868997109, 13.79486065368817194, -63.89999999999997016 ) ) ;
#2867=CARTESIAN_POINT ( 'NONE',  ( -1.758463861404912842, 21.27107139401109137, -51.90704692567388179 ) ) ;
#2870=CARTESIAN_POINT ( 'NONE',  ( 1.887862790868997109, 13.79486065368817194, -72.89999999999996305 ) ) ;
#2873=CARTESIAN_POINT ( 'NONE',  ( -2.017261720333081598, 21.13920729861251857, -48.89295307432605853 ) ) ;
#2888=CARTESIAN_POINT ( 'NONE',  ( 4.206979645153767322, 13.29302035484617051, -48.74999999999997158 ) ) ;
#2904=CARTESIAN_POINT ( 'NONE',  ( 5.041649132594343996, 14.93115145952162415, -66.59999999999996589 ) ) ;
#2910=CARTESIAN_POINT ( 'NONE',  ( -0.6839900399647736995, 21.81854315085035623, -38.54999999999996874 ) ) ;
#2911=CARTESIAN_POINT ( 'NONE',  ( -5.900206406879871857, 18.27989588542834554, -45.44295307432605568 ) ) ;
#2920=CARTESIAN_POINT ( 'NONE',  ( -4.084459969179292216, 16.70604699712905372, -57.29295307432606421 ) ) ;
#2936=CARTESIAN_POINT ( 'NONE',  ( -3.091735541773221296, 20.59173554177323950, -35.24999999999997158 ) ) ;
#2938=DIRECTION ( 'NONE',  ( -0.7037848285661852943, 0.7037848285661921777, -0.09681854243955982653 ) ) ;
#2961=CARTESIAN_POINT ( 'NONE',  ( -3.639207298612509689, 19.51726172033310647, -33.60704692567387042 ) ) ;
#2962=CARTESIAN_POINT ( 'NONE',  ( -0.6839900399647738105, 21.81854315085035623, -29.54999999999996518 ) ) ;
#2964=CARTESIAN_POINT ( 'NONE',  ( 0.7417250638684235176, 23.11142975074950101, -31.19295307432605568 ) ) ;
#2965=CARTESIAN_POINT ( 'NONE',  ( -4.107178604518053611, 16.84948681541050775, -25.79999999999996163 ) ) ;
#2973=CARTESIAN_POINT ( 'NONE',  ( -3.705139346311794313, 19.38786279086902198, -50.09999999999996589 ) ) ;
#2976=CARTESIAN_POINT ( 'NONE',  ( 0.7798958854283032371, 11.59979359312010772, -35.55704692567386616 ) ) ;
#2977=CARTESIAN_POINT ( 'NONE',  ( 4.001075405444606048, 21.50107540544455276, -29.99999999999996447 ) ) ;
#2978=CARTESIAN_POINT ( 'NONE',  ( -3.705139346311794313, 19.38786279086902198, -62.09999999999996589 ) ) ;
#2987=CARTESIAN_POINT ( 'NONE',  ( 2.837105286290961370, 22.73177855326409613, -25.35704692567387042 ) ) ;
#2993=CARTESIAN_POINT ( 'NONE',  ( 3.898383833589191383, 21.60376697729997275, -40.49295307432605995 ) ) ;
#3011=CARTESIAN_POINT ( 'NONE',  ( -4.314955953707389824, 21.59900333660018390, -63.74295307432605995 ) ) ;
#3017=CARTESIAN_POINT ( 'NONE',  ( -0.6839900399647736995, 21.81854315085035623, -53.54999999999996163 ) ) ;
#3027=CARTESIAN_POINT ( 'NONE',  ( 2.837105286290961370, 22.73177855326409613, -61.35704692567387752 ) ) ;
#3028=CARTESIAN_POINT ( 'NONE',  ( 5.876318620034919782, 16.56928256419707068, -54.44999999999996021 ) ) ;
#3041=CARTESIAN_POINT ( 'NONE',  ( -0.7798958854283041253, 23.40020640687986386, -52.05704692567388747 ) ) ;
#3046=CARTESIAN_POINT ( 'NONE',  ( 5.107581180293630396, 15.06055038898570686, -74.09295307432606137 ) ) ;
#3063=CARTESIAN_POINT ( 'NONE',  ( 0.9307174358028528216, 11.62368137996505801, -43.04999999999996163 ) ) ;
#3067=CARTESIAN_POINT ( 'NONE',  ( -3.639207298612509689, 19.51726172033310647, -63.60704692567387752 ) ) ;
#3068=CARTESIAN_POINT ( 'NONE',  ( 3.091735541773220852, 14.40826445822673740, -51.74999999999995026 ) ) ;
#3078=CARTESIAN_POINT ( 'NONE',  ( 4.107178604518054499, 18.15051318458946383, -63.29999999999996874 ) ) ;
#3081=CARTESIAN_POINT ( 'NONE',  ( 3.965139115708213868, 19.34895832295540430, -43.65704692567387468 ) ) ;
#3086=CARTESIAN_POINT ( 'NONE',  ( 3.826489000663266360, 19.62107449533211678, -43.64295307432605853 ) ) ;
#3103=CARTESIAN_POINT ( 'NONE',  ( 2.701047200102605572, 22.80110361078655856, -47.84999999999994458 ) ) ;
#3113=EDGE_LOOP ( 'NONE', ( #6953, #20798, #19476, #12977 ) ) ;
#3116=CARTESIAN_POINT ( 'NONE',  ( -5.876318620034919782, 18.43071743580290089, -73.94999999999997442 ) ) ;
#3122=CARTESIAN_POINT ( 'NONE',  ( 3.895814058185739448, 19.48501640914375344, -42.14999999999996305 ) ) ;
#3134=CARTESIAN_POINT ( 'NONE',  ( 3.199711850326839357, 14.51624076678035635, -56.24295307432605995 ) ) ;
#3151=CARTESIAN_POINT ( 'NONE',  ( 0.6839900399647733664, 13.18145684914961357, -40.04999999999994742 ) ) ;
#3175=CARTESIAN_POINT ( 'NONE',  ( 4.294655364005415699, 16.66518840966061887, -31.95704692567387184 ) ) ;
#3176=CARTESIAN_POINT ( 'NONE',  ( -1.887862790868997553, 21.20513934631180319, -32.39999999999996305 ) ) ;
#3179=CARTESIAN_POINT ( 'NONE',  ( -5.900206406879871857, 18.27989588542834554, -36.44295307432606279 ) ) ;
#3180=CARTESIAN_POINT ( 'NONE',  ( -2.940415233664778860, 14.55958476633523802, -25.49999999999996803 ) ) ;
#3188=CARTESIAN_POINT ( 'NONE',  ( -4.107178604518053611, 16.84948681541050775, -49.79999999999996874 ) ) ;
#3191=CARTESIAN_POINT ( 'NONE',  ( 0.7798958854283032371, 11.59979359312010772, -41.55704692567387326 ) ) ;
#3192=CARTESIAN_POINT ( 'NONE',  ( -2.701047200102606460, 12.19889638921340591, -31.34999999999996945 ) ) ;
#3193=CARTESIAN_POINT ( 'NONE',  ( -3.895814058185739448, 15.51498359085620571, -61.64999999999995595 ) ) ;
#3206=CARTESIAN_POINT ( 'NONE',  ( 5.231778553264135212, 20.33710528629089254, -37.64295307432604432 ) ) ;
#3223=CARTESIAN_POINT ( 'NONE',  ( -4.107178604518053611, 16.84948681541050775, -25.79999999999996163 ) ) ;
#3224=CARTESIAN_POINT ( 'NONE',  ( 1.985016409143818272, 21.39581405818570303, -50.84999999999997300 ) ) ;
#3235=CARTESIAN_POINT ( 'NONE',  ( -1.028604700431329233, 11.93400751992799513, -62.70704692567387184 ) ) ;
#3236=CARTESIAN_POINT ( 'NONE',  ( -5.588711115410763597, 16.61483511785016987, -52.79999999999996874 ) ) ;
#3247=CARTESIAN_POINT ( 'NONE',  ( 2.439449611014226971, 12.39241881970633230, -50.40704692567388179 ) ) ;
#3254=CARTESIAN_POINT ( 'NONE',  ( -2.698247469942396837, 22.47571708489507358, -69.89295307432607274 ) ) ;
#3268=CARTESIAN_POINT ( 'NONE',  ( -4.206979645153768210, 21.70697964515380107, -44.24999999999997868 ) ) ;
#3271=CARTESIAN_POINT ( 'NONE',  ( -1.758463861404912842, 21.27107139401109137, -66.90704692567388179 ) ) ;
#3272=CARTESIAN_POINT ( 'NONE',  ( -3.705139346311794313, 19.38786279086902198, -47.09999999999996589 ) ) ;
#3283=CARTESIAN_POINT ( 'NONE',  ( 3.091735541773220852, 14.40826445822673563, -60.74999999999995737 ) ) ;
#3285=CARTESIAN_POINT ( 'NONE',  ( 0.7939530028709752552, 21.58445996917927445, -46.20704692567387184 ) ) ;
#3289=CARTESIAN_POINT ( 'NONE',  ( 4.084459969179292216, 18.29395300287091430, -40.79295307432605711 ) ) ;
#3302=CARTESIAN_POINT ( 'NONE',  ( -5.876318620034919782, 18.43071743580290089, -52.94999999999994600 ) ) ;
#3319=CARTESIAN_POINT ( 'NONE',  ( 2.568848540478311460, 12.45835086740561692, -72.89999999999996305 ) ) ;
#3325=CARTESIAN_POINT ( 'NONE',  ( -3.895814058185739448, 15.51498359085620571, -43.64999999999996305 ) ) ;
#3336=CARTESIAN_POINT ( 'NONE',  ( -1.848958322955462474, 13.53486088429179546, -56.84295307432604716 ) ) ;
#3353=CARTESIAN_POINT ( 'NONE',  ( 3.091735541773220852, 14.40826445822673563, -33.74999999999996447 ) ) ;
#3381=CARTESIAN_POINT ( 'NONE',  ( -4.294655364005415699, 18.33481159033935626, -36.45704692567386473 ) ) ;
#3384=CARTESIAN_POINT ( 'NONE',  ( -0.7417250638684240727, 11.88857024925047057, -32.69295307432605568 ) ) ;
#3385=CARTESIAN_POINT ( 'NONE',  ( 3.965139115708213868, 19.34895832295540430, -70.65704692567386758 ) ) ;
#3392=CARTESIAN_POINT ( 'NONE',  ( -1.985016409143819605, 13.60418594181426855, -49.34999999999996589 ) ) ;
#3394=CARTESIAN_POINT ( 'NONE',  ( 2.439449611014226971, 12.39241881970633230, -35.40704692567386758 ) ) ;
#3395=CARTESIAN_POINT ( 'NONE',  ( -5.301103610786608300, 14.79895279989743528, -25.64999999999996305 ) ) ;
#3396=CARTESIAN_POINT ( 'NONE',  ( -0.6505131845895224529, 13.39282139548194195, -67.19999999999997442 ) ) ;
#3407=CARTESIAN_POINT ( 'NONE',  ( -5.107581180293630396, 19.93944961101426827, -27.59295307432605782 ) ) ;
#3424=CARTESIAN_POINT ( 'NONE',  ( 4.318543150850367773, 16.81600996003516357, -27.44999999999996021 ) ) ;
#3425=CARTESIAN_POINT ( 'NONE',  ( 0.6505131845895220088, 21.60717860451803674, -56.69999999999997442 ) ) ;
#3435=CARTESIAN_POINT ( 'NONE',  ( 0.7798958854283032371, 11.59979359312010772, -65.55704692567385905 ) ) ;
#3436=CARTESIAN_POINT ( 'NONE',  ( -2.568848540478311904, 22.54164913259435465, -56.39999999999996305 ) ) ;
#3449=CARTESIAN_POINT ( 'NONE',  ( -4.103766977300021601, 13.60161616641083704, -45.00704692567388321 ) ) ;
#3454=CARTESIAN_POINT ( 'NONE',  ( 5.565992480072003978, 18.52860470043125574, -61.79295307432605000 ) ) ;
#3469=CARTESIAN_POINT ( 'NONE',  ( 5.301103610786608300, 20.20104720010253985, -45.14999999999994884 ) ) ;
#3472=CARTESIAN_POINT ( 'NONE',  ( -2.983759233219601903, 20.69971185032686023, -60.75704692567388321 ) ) ;
#3473=CARTESIAN_POINT ( 'NONE',  ( 0.6505131845895220088, 21.60717860451803674, -47.69999999999996732 ) ) ;
#3484=CARTESIAN_POINT ( 'NONE',  ( 0.6505131845895220088, 21.60717860451803674, -68.69999999999997442 ) ) ;
#3486=CARTESIAN_POINT ( 'NONE',  ( 2.121074495332174958, 21.32648900066323350, -43.35704692567387752 ) ) ;
#3490=CARTESIAN_POINT ( 'NONE',  ( -3.199711850326840246, 20.48375923321962233, -39.74295307432605995 ) ) ;
#3497=CARTESIAN_POINT ( 'NONE',  ( -3.639207298612509689, 19.51726172033310647, -27.60704692567387397 ) ) ;
#3503=CARTESIAN_POINT ( 'NONE',  ( 0.9307174358028528216, 11.62368137996505801, -49.04999999999994742 ) ) ;
#3520=CARTESIAN_POINT ( 'NONE',  ( 5.588711115410763597, 18.38516488214980882, -69.29999999999996874 ) ) ;
#3525=CARTESIAN_POINT ( 'NONE',  ( 1.887862790868997109, 13.79486065368817194, -42.89999999999996305 ) ) ;
#3526=CARTESIAN_POINT ( 'NONE',  ( -0.6839900399647738105, 21.81854315085035623, -74.54999999999995453 ) ) ;
#3536=CARTESIAN_POINT ( 'NONE',  ( -2.837723661809363751, 14.45689319447982335, -47.99295307432606705 ) ) ;
#3542=CARTESIAN_POINT ( 'NONE',  ( -2.837723661809363751, 14.45689319447982335, -65.99295307432606705 ) ) ;
#3553=CARTESIAN_POINT ( 'NONE',  ( 0.6505131845895220088, 21.60717860451803674, -35.69999999999996732 ) ) ;
#3579=CARTESIAN_POINT ( 'NONE',  ( -3.043106805520194413, 14.66227633819065623, -30.00704692567387610 ) ) ;
#3584=CARTESIAN_POINT ( 'NONE',  ( 3.898383833589191383, 21.60376697729997275, -37.49295307432604574 ) ) ;
#3585=CARTESIAN_POINT ( 'NONE',  ( -0.5331684895902242260, 21.84243093769531185, -64.05704692567387326 ) ) ;
#3594=CARTESIAN_POINT ( 'NONE',  ( 3.091735541773220852, 14.40826445822673563, -48.74999999999997158 ) ) ;
#3598=CARTESIAN_POINT ( 'NONE',  ( -2.837105286290963146, 12.26822144673588255, -41.85704692567387752 ) ) ;
#3600=CARTESIAN_POINT ( 'NONE',  ( -1.985016409143819605, 13.60418594181426855, -67.34999999999996589 ) ) ;
#3614=CARTESIAN_POINT ( 'NONE',  ( 2.698247469942395949, 12.52428291510489977, -35.39295307432605142 ) ) ;
#3634=CARTESIAN_POINT ( 'NONE',  ( 3.091735541773220852, 14.40826445822673563, -54.74999999999997158 ) ) ;
#3641=CARTESIAN_POINT ( 'NONE',  ( -0.6505131845895224529, 13.39282139548194195, -73.19999999999997442 ) ) ;
#3643=CARTESIAN_POINT ( 'NONE',  ( 4.975717084895059372, 14.80175253005754143, -65.10704692567387042 ) ) ;
#3644=CARTESIAN_POINT ( 'NONE',  ( -5.301103610786608300, 14.79895279989743528, -52.64999999999997016 ) ) ;
#3659=CARTESIAN_POINT ( 'NONE',  ( -4.099003336600151925, 21.81495595370741469, -42.75704692567387610 ) ) ;
#3665=CARTESIAN_POINT ( 'NONE',  ( -1.081538986177402961, 23.35243083318996327, -61.04295307432605711 ) ) ;
#3681=CARTESIAN_POINT ( 'NONE',  ( -5.588711115410763597, 16.61483511785016987, -28.79999999999996518 ) ) ;
#3684=CARTESIAN_POINT ( 'NONE',  ( 4.129897239856814117, 18.00707336630801336, -55.80704692567388037 ) ) ;
#3685=CARTESIAN_POINT ( 'NONE',  ( -3.705139346311794313, 19.38786279086902198, -44.09999999999996589 ) ) ;
#3694=CARTESIAN_POINT ( 'NONE',  ( 1.887862790868997109, 13.79486065368817194, -57.89999999999996305 ) ) ;
#3696=CARTESIAN_POINT ( 'NONE',  ( 3.965139115708213868, 19.34895832295540430, -46.65704692567388179 ) ) ;
#3700=CARTESIAN_POINT ( 'NONE',  ( 1.848958322955461808, 21.46513911570817612, -37.34295307432606137 ) ) ;
#3706=CARTESIAN_POINT ( 'NONE',  ( -4.129897239856814117, 16.99292663369196177, -24.30704692567386971 ) ) ;
#3712=CARTESIAN_POINT ( 'NONE',  ( -4.206979645153768210, 21.70697964515380107, -38.24999999999996447 ) ) ;
#3731=CARTESIAN_POINT ( 'NONE',  ( 5.041649132594343996, 14.93115145952162415, -72.59999999999996589 ) ) ;
#3736=CARTESIAN_POINT ( 'NONE',  ( -2.940415233664778860, 14.55958476633523802, -31.49999999999996447 ) ) ;
#3749=CARTESIAN_POINT ( 'NONE',  ( -3.199711850326840246, 20.48375923321962233, -48.74295307432605284 ) ) ;
#3754=CARTESIAN_POINT ( 'NONE',  ( 2.017261720333081598, 13.86079270138745834, -59.39295307432605853 ) ) ;
#3766=CARTESIAN_POINT ( 'NONE',  ( 4.107178604518054499, 18.15051318458946383, -27.29999999999996163 ) ) ;
#3774=CARTESIAN_POINT ( 'NONE',  ( 4.206979645153767322, 13.29302035484617051, -69.74999999999997158 ) ) ;
#3792=CARTESIAN_POINT ( 'NONE',  ( 0.7417250638684235176, 23.11142975074950101, -67.19295307432605568 ) ) ;
#3796=CARTESIAN_POINT ( 'NONE',  ( -3.965139115708213868, 15.65104167704456906, -36.15704692567386758 ) ) ;
#3801=CARTESIAN_POINT ( 'NONE',  ( -0.7417250638684240727, 11.88857024925047057, -29.69295307432606279 ) ) ;
#3803=CARTESIAN_POINT ( 'NONE',  ( -0.7939530028709754772, 13.41554003082070246, -59.70704692567387184 ) ) ;
#3812=CARTESIAN_POINT ( 'NONE',  ( -1.887862790868997553, 21.20513934631180319, -41.39999999999996305 ) ) ;
#3815=CARTESIAN_POINT ( 'NONE',  ( -4.099003336600151925, 21.81495595370741469, -27.75704692567387255 ) ) ;
#3817=CARTESIAN_POINT ( 'NONE',  ( -1.887862790868997553, 21.20513934631180319, -53.39999999999997016 ) ) ;
#3830=CARTESIAN_POINT ( 'NONE',  ( 1.081538986177402295, 11.64756916681001186, -32.54295307432605711 ) ) ;
#3849=CARTESIAN_POINT ( 'NONE',  ( -4.107178604518053611, 16.84948681541050775, -46.79999999999996874 ) ) ;
#3859=CARTESIAN_POINT ( 'NONE',  ( -3.091735541773221296, 20.59173554177323950, -74.24999999999997158 ) ) ;
#3861=CARTESIAN_POINT ( 'NONE',  ( -5.370428668309080500, 14.93501088608579153, -54.15704692567387468 ) ) ;
#3862=CARTESIAN_POINT ( 'NONE',  ( -2.568848540478311904, 22.54164913259435465, -50.39999999999996305 ) ) ;
#3876=CARTESIAN_POINT ( 'NONE',  ( 2.837105286290961370, 22.73177855326409613, -49.35704692567387042 ) ) ;
#3880=CARTESIAN_POINT ( 'NONE',  ( 2.564989113914249330, 22.87042866830903876, -64.34295307432606137 ) ) ;
#3887=CARTESIAN_POINT ( 'NONE',  ( 2.940415233664778416, 20.44041523366473712, -74.99999999999997158 ) ) ;
#3892=CARTESIAN_POINT ( 'NONE',  ( 0.9307174358028528216, 11.62368137996505801, -34.04999999999995453 ) ) ;
#3896=CARTESIAN_POINT ( 'NONE',  ( 2.983759233219601459, 14.30028814967311668, -50.25704692567386900 ) ) ;
#3897=CARTESIAN_POINT ( 'NONE',  ( -3.895814058185739892, 15.51498359085620748, -34.64999999999997016 ) ) ;
#3898=CARTESIAN_POINT ( 'NONE',  ( -3.091735541773221296, 20.59173554177323950, -74.24999999999997158 ) ) ;
#3906=CARTESIAN_POINT ( 'NONE',  ( -1.887862790868997553, 21.20513934631180319, -50.39999999999996305 ) ) ;
#3908=CARTESIAN_POINT ( 'NONE',  ( 4.129897239856814117, 18.00707336630801336, -40.80704692567388037 ) ) ;
#3909=CARTESIAN_POINT ( 'NONE',  ( -5.876318620034919782, 18.43071743580290089, -70.94999999999997442 ) ) ;
#3912=CARTESIAN_POINT ( 'NONE',  ( -2.017261720333081598, 21.13920729861251857, -33.89295307432605142 ) ) ;
#3919=CARTESIAN_POINT ( 'NONE',  ( -5.852430833189966819, 18.58153898617744915, -72.45704692567387895 ) ) ;
#3925=CARTESIAN_POINT ( 'NONE',  ( 4.206979645153767322, 13.29302035484617051, -39.74999999999996447 ) ) ;
#3942=CARTESIAN_POINT ( 'NONE',  ( -5.876318620034919782, 18.43071743580290089, -64.94999999999996021 ) ) ;
#3948=CARTESIAN_POINT ( 'NONE',  ( -3.091735541773221296, 20.59173554177323950, -32.24999999999996447 ) ) ;
#3949=CARTESIAN_POINT ( 'NONE',  ( 1.887862790868997109, 13.79486065368817194, -72.89999999999996305 ) ) ;
#3960=CARTESIAN_POINT ( 'NONE',  ( 2.837723661809363307, 20.54310680552015356, -46.49295307432606705 ) ) ;
#3965=CARTESIAN_POINT ( 'NONE',  ( 3.826489000663266360, 19.62107449533211678, -64.64295307432604432 ) ) ;
#3975=CARTESIAN_POINT ( 'NONE',  ( -4.107178604518053611, 16.84948681541050775, -25.79999999999996163 ) ) ;
#3983=VERTEX_POINT ( 'NONE', #8918 ) ;
#3984=CARTESIAN_POINT ( 'NONE',  ( -2.568848540478311904, 22.54164913259435465, -71.39999999999996305 ) ) ;
#3999=CARTESIAN_POINT ( 'NONE',  ( -3.898383833589191827, 13.39623302270000771, -62.99295307432606705 ) ) ;
#4008=CARTESIAN_POINT ( 'NONE',  ( 2.837723661809363307, 20.54310680552015356, -76.49295307432603863 ) ) ;
#4010=CARTESIAN_POINT ( 'NONE',  ( 4.294655364005415699, 16.66518840966061887, -67.95704692567387895 ) ) ;
#4022=CARTESIAN_POINT ( 'NONE',  ( 5.611429750749524992, 18.24172506386835479, -25.80704692567386971 ) ) ;
#4024=CARTESIAN_POINT ( 'NONE',  ( 1.887862790868997109, 13.79486065368817194, -54.89999999999996305 ) ) ;
#4031=CARTESIAN_POINT ( 'NONE',  ( -5.565992480072003978, 16.47139529956871229, -39.29295307432605711 ) ) ;
#4038=CARTESIAN_POINT ( 'NONE',  ( 5.565992480072003978, 18.52860470043125574, -34.79295307432605711 ) ) ;
#4055=CARTESIAN_POINT ( 'NONE',  ( 0.6839900399647733664, 13.18145684914961357, -43.04999999999996163 ) ) ;
#4064=CARTESIAN_POINT ( 'NONE',  ( -0.6839900399647736995, 21.81854315085035623, -68.54999999999998295 ) ) ;
#4066=CARTESIAN_POINT ( 'NONE',  ( -4.103766977300021601, 13.60161616641083704, -54.00704692567387610 ) ) ;
#4067=CARTESIAN_POINT ( 'NONE',  ( -5.588711115410763597, 16.61483511785016987, -49.79999999999996874 ) ) ;
#4076=PRODUCT ( 'Spring', 'Spring', '', ( #9700 ) ) ;
#4082=CARTESIAN_POINT ( 'NONE',  ( 4.103766977300021601, 21.39838383358913987, -49.50704692567387610 ) ) ;
#4086=CARTESIAN_POINT ( 'NONE',  ( -3.898383833589191827, 13.39623302270000771, -59.99295307432606705 ) ) ;
#4102=CARTESIAN_POINT ( 'NONE',  ( 4.001075405444606048, 21.50107540544455276, -35.99999999999996447 ) ) ;
#4105=CARTESIAN_POINT ( 'NONE',  ( 1.758463861404912620, 13.72892860598888731, -53.40704692567386758 ) ) ;
#4115=CARTESIAN_POINT ( 'NONE',  ( -1.887862790868997553, 21.20513934631180319, -56.39999999999996305 ) ) ;
#4117=CARTESIAN_POINT ( 'NONE',  ( -3.965139115708213868, 15.65104167704456906, -36.15704692567386758 ) ) ;
#4118=CARTESIAN_POINT ( 'NONE',  ( -5.301103610786608300, 14.79895279989743528, -73.64999999999994884 ) ) ;
#4122=CARTESIAN_POINT ( 'NONE',  ( 2.837723661809363307, 20.54310680552015356, -31.49295307432605995 ) ) ;
#4129=CARTESIAN_POINT ( 'NONE',  ( 3.965139115708213868, 19.34895832295540430, -25.65704692567387823 ) ) ;
#4136=CARTESIAN_POINT ( 'NONE',  ( -4.001075405444606936, 13.49892459455542060, -37.49999999999996447 ) ) ;
#4154=CARTESIAN_POINT ( 'NONE',  ( -5.041649132594344884, 20.06884854047834921, -62.09999999999996589 ) ) ;
#4159=CARTESIAN_POINT ( 'NONE',  ( -2.940415233664778860, 14.55958476633523802, -34.49999999999997158 ) ) ;
#4160=CARTESIAN_POINT ( 'NONE',  ( -3.091735541773221296, 20.59173554177323950, -68.24999999999995737 ) ) ;
#4172=CARTESIAN_POINT ( 'NONE',  ( 2.017261720333081598, 13.86079270138745834, -47.39295307432605853 ) ) ;
#4179=CARTESIAN_POINT ( 'NONE',  ( -1.848958322955462474, 13.53486088429179546, -68.84295307432606137 ) ) ;
#4190=CARTESIAN_POINT ( 'NONE',  ( 0.6505131845895220088, 21.60717860451803674, -29.69999999999996376 ) ) ;
#4198=CARTESIAN_POINT ( 'NONE',  ( 0.9307174358028528216, 11.62368137996505801, -67.04999999999994031 ) ) ;
#4218=CARTESIAN_POINT ( 'NONE',  ( 2.698247469942395949, 12.52428291510489977, -50.39295307432605853 ) ) ;
#4226=CARTESIAN_POINT ( 'NONE',  ( -4.084459969179292216, 16.70604699712905372, -72.29295307432605000 ) ) ;
#4228=CARTESIAN_POINT ( 'NONE',  ( 3.965139115708213868, 19.34895832295540430, -67.65704692567386758 ) ) ;
#4240=CARTESIAN_POINT ( 'NONE',  ( 4.103766977300021601, 21.39838383358913987, -31.50704692567387610 ) ) ;
#4242=CARTESIAN_POINT ( 'NONE',  ( -3.705139346311794313, 19.38786279086902198, -53.09999999999996589 ) ) ;
#4254=CARTESIAN_POINT ( 'NONE',  ( 4.314955953707388936, 13.40099666339979123, -32.24295307432605284 ) ) ;
#4274=CARTESIAN_POINT ( 'NONE',  ( -1.985016409143819605, 13.60418594181426855, -40.34999999999996589 ) ) ;
#4283=CARTESIAN_POINT ( 'NONE',  ( -3.895814058185739448, 15.51498359085620571, -64.64999999999994884 ) ) ;
#4285=CARTESIAN_POINT ( 'NONE',  ( -5.852430833189966819, 18.58153898617744915, -54.45704692567387895 ) ) ;
#4286=CARTESIAN_POINT ( 'NONE',  ( -0.8851648821498765418, 11.91128888458923285, -49.19999999999996732 ) ) ;
#4299=CARTESIAN_POINT ( 'NONE',  ( -5.852430833189966819, 18.58153898617744915, -45.45704692567387184 ) ) ;
#4303=CARTESIAN_POINT ( 'NONE',  ( 1.081538986177402295, 11.64756916681001186, -65.54295307432606421 ) ) ;
#4320=CARTESIAN_POINT ( 'NONE',  ( -5.041649132594344884, 20.06884854047834921, -29.09999999999996589 ) ) ;
#4323=CARTESIAN_POINT ( 'NONE',  ( 2.121074495332174958, 21.32648900066323350, -52.35704692567387042 ) ) ;
#4324=CARTESIAN_POINT ( 'NONE',  ( 0.6505131845895220088, 21.60717860451803674, -74.69999999999997442 ) ) ;
#4331=CARTESIAN_POINT ( 'NONE',  ( -3.091735541773221296, 20.59173554177323950, -53.24999999999996447 ) ) ;
#4333=CARTESIAN_POINT ( 'NONE',  ( -0.5331684895902242260, 21.84243093769531185, -34.05704692567386616 ) ) ;
#4339=CARTESIAN_POINT ( 'NONE',  ( -2.837723661809363751, 14.45689319447982335, -38.99295307432604574 ) ) ;
#4348=CARTESIAN_POINT ( 'NONE',  ( 4.294655364005415699, 16.66518840966061887, -25.95704692567387184 ) ) ;
#4353=CARTESIAN_POINT ( 'NONE',  ( -5.041649132594344884, 20.06884854047834921, -35.09999999999996589 ) ) ;
#4372=CARTESIAN_POINT ( 'NONE',  ( 5.041649132594343996, 14.93115145952162415, -57.59999999999997300 ) ) ;
#4378=CARTESIAN_POINT ( 'NONE',  ( -0.6839900399647736995, 21.81854315085035623, -29.54999999999996518 ) ) ;
#4379=CARTESIAN_POINT ( 'NONE',  ( 3.895814058185739892, 19.48501640914376054, -69.14999999999996305 ) ) ;
#4391=CARTESIAN_POINT ( 'NONE',  ( -4.342430937695320736, 18.03316848959025620, -45.44295307432605568 ) ) ;
#4396=CARTESIAN_POINT ( 'NONE',  ( 3.826489000663266360, 19.62107449533211678, -67.64295307432605853 ) ) ;
#4415=CARTESIAN_POINT ( 'NONE',  ( 4.206979645153767322, 13.29302035484617051, -63.74999999999997868 ) ) ;
#4435=CARTESIAN_POINT ( 'NONE',  ( 2.698247469942395949, 12.52428291510489977, -56.39295307432605853 ) ) ;
#4445=CARTESIAN_POINT ( 'NONE',  ( 1.848958322955461808, 21.46513911570817612, -73.34295307432607558 ) ) ;
#4447=CARTESIAN_POINT ( 'NONE',  ( -0.7939530028709754772, 13.41554003082070246, -65.70704692567387895 ) ) ;
#4458=CARTESIAN_POINT ( 'NONE',  ( -4.975717084895059372, 20.19824746994243370, -24.60704692567387397 ) ) ;
#4460=CARTESIAN_POINT ( 'NONE',  ( 3.895814058185739448, 19.48501640914375344, -51.14999999999994884 ) ) ;
#4472=CARTESIAN_POINT ( 'NONE',  ( -3.898383833589191827, 13.39623302270000771, -26.99295307432605995 ) ) ;
#4488=CARTESIAN_POINT ( 'NONE',  ( -2.940415233664778860, 14.55958476633523802, -49.49999999999996447 ) ) ;
#4497=CARTESIAN_POINT ( 'NONE',  ( 3.091735541773220852, 14.40826445822673563, -63.74999999999997868 ) ) ;
#4499=CARTESIAN_POINT ( 'NONE',  ( -0.7798958854283041253, 23.40020640687986386, -52.05704692567388747 ) ) ;
#4500=CARTESIAN_POINT ( 'NONE',  ( -4.001075405444606936, 13.49892459455542060, -49.49999999999996447 ) ) ;
#4512=CARTESIAN_POINT ( 'NONE',  ( -0.7798958854283041253, 23.40020640687986386, -37.05704692567387326 ) ) ;
#4513=VERTEX_POINT ( 'NONE', #27124 ) ;
#4515=CARTESIAN_POINT ( 'NONE',  ( 4.314955953707388936, 13.40099666339979123, -50.24295307432605284 ) ) ;
#4530=CARTESIAN_POINT ( 'NONE',  ( -0.8851648821498765418, 11.91128888458923285, -31.19999999999996376 ) ) ;
#4533=CARTESIAN_POINT ( 'NONE',  ( -3.639207298612509689, 19.51726172033310647, -48.60704692567386331 ) ) ;
#4534=CARTESIAN_POINT ( 'NONE',  ( -3.705139346311794313, 19.38786279086902198, -74.09999999999996589 ) ) ;
#4543=CARTESIAN_POINT ( 'NONE',  ( -3.091735541773221296, 20.59173554177323950, -59.24999999999997158 ) ) ;
#4545=CARTESIAN_POINT ( 'NONE',  ( 2.983759233219601459, 14.30028814967311668, -35.25704692567386900 ) ) ;
#4546=CARTESIAN_POINT ( 'NONE',  ( -5.041649132594344884, 20.06884854047834921, -71.09999999999996589 ) ) ;
#4558=CARTESIAN_POINT ( 'NONE',  ( -4.975717084895059372, 20.19824746994243370, -63.60704692567387752 ) ) ;
#4562=CARTESIAN_POINT ( 'NONE',  ( -2.568848540478311904, 22.54164913259435465, -38.39999999999997016 ) ) ;
#4579=CARTESIAN_POINT ( 'NONE',  ( 5.588711115410763597, 18.38516488214980882, -63.29999999999996874 ) ) ;
#4584=CARTESIAN_POINT ( 'NONE',  ( 4.107178604518054499, 18.15051318458946383, -30.29999999999996518 ) ) ;
#4586=CARTESIAN_POINT ( 'NONE',  ( -4.318543150850366885, 18.18399003996480801, -70.94999999999997442 ) ) ;
#4596=CARTESIAN_POINT ( 'NONE',  ( -0.5070733663080690956, 13.37010276014318144, -32.69295307432605568 ) ) ;
#4601=CARTESIAN_POINT ( 'NONE',  ( 4.084459969179292216, 18.29395300287091430, -49.79295307432606421 ) ) ;
#4619=CARTESIAN_POINT ( 'NONE',  ( 5.041649132594343996, 14.93115145952162415, -66.59999999999996589 ) ) ;
#4641=CARTESIAN_POINT ( 'NONE',  ( 1.081538986177402295, 11.64756916681001186, -53.54295307432606421 ) ) ;
#4648=CARTESIAN_POINT ( 'NONE',  ( -0.8348115903393239501, 21.79465536400541126, -70.04295307432606421 ) ) ;
#4650=CARTESIAN_POINT ( 'NONE',  ( 2.983759233219601459, 14.30028814967311668, -50.25704692567386900 ) ) ;
#4662=CARTESIAN_POINT ( 'NONE',  ( 3.895814058185739448, 19.48501640914375344, -54.14999999999997726 ) ) ;
#4674=CARTESIAN_POINT ( 'NONE',  ( 2.837723661809363307, 20.54310680552015356, -73.49295307432603863 ) ) ;
#4688=CARTESIAN_POINT ( 'NONE',  ( -3.091735541773221296, 20.59173554177323950, -35.24999999999997158 ) ) ;
#4693=CARTESIAN_POINT ( 'NONE',  ( -1.887862790868997553, 21.20513934631180319, -32.39999999999996305 ) ) ;
#4702=CARTESIAN_POINT ( 'NONE',  ( 1.887862790868997109, 13.79486065368817194, -63.89999999999997016 ) ) ;
#4704=CARTESIAN_POINT ( 'NONE',  ( -2.439449611014227859, 22.60758118029364283, -54.90704692567386758 ) ) ;
#4705=CARTESIAN_POINT ( 'NONE',  ( -5.301103610786608300, 14.79895279989743528, -31.64999999999996660 ) ) ;
#4719=CARTESIAN_POINT ( 'NONE',  ( 0.7798958854283032371, 11.59979359312010772, -35.55704692567386616 ) ) ;
#4722=CARTESIAN_POINT ( 'NONE',  ( -1.081538986177402961, 23.35243083318996327, -55.04295307432606421 ) ) ;
#4739=CARTESIAN_POINT ( 'NONE',  ( 5.107581180293630396, 15.06055038898570686, -71.09295307432604716 ) ) ;
#4742=CARTESIAN_POINT ( 'NONE',  ( 4.294655364005415699, 16.66518840966061887, -43.95704692567387184 ) ) ;
#4743=CARTESIAN_POINT ( 'NONE',  ( 4.107178604518054499, 18.15051318458946383, -69.29999999999996874 ) ) ;
#4750=CARTESIAN_POINT ( 'NONE',  ( 3.895814058185739448, 19.48501640914375344, -48.14999999999997726 ) ) ;
#4753=CARTESIAN_POINT ( 'NONE',  ( 3.965139115708213868, 19.34895832295540430, -37.65704692567386758 ) ) ;
#4763=CARTESIAN_POINT ( 'NONE',  ( 0.7798958854283032371, 11.59979359312010772, -65.55704692567385905 ) ) ;
#4768=CARTESIAN_POINT ( 'NONE',  ( 3.898383833589191383, 21.60376697729997275, -76.49295307432603863 ) ) ;
#4787=CARTESIAN_POINT ( 'NONE',  ( -5.876318620034919782, 18.43071743580290089, -58.94999999999995310 ) ) ;
#4791=CARTESIAN_POINT ( 'NONE',  ( 3.639207298612508801, 15.48273827966686866, -68.10704692567387042 ) ) ;
#4792=CARTESIAN_POINT ( 'NONE',  ( 2.940415233664778416, 20.44041523366473712, -65.99999999999997158 ) ) ;
#4803=CARTESIAN_POINT ( 'NONE',  ( 4.084459969179292216, 18.29395300287091430, -31.79295307432605355 ) ) ;
#4807=CARTESIAN_POINT ( 'NONE',  ( -1.848958322955462474, 13.53486088429179546, -53.84295307432606137 ) ) ;
#4824=CARTESIAN_POINT ( 'NONE',  ( 2.701047200102605572, 22.80110361078655856, -56.84999999999995879 ) ) ;
#4843=CARTESIAN_POINT ( 'NONE',  ( 5.565992480072003978, 18.52860470043125574, -55.79295307432606421 ) ) ;
#4851=CARTESIAN_POINT ( 'NONE',  ( -2.017261720333081598, 21.13920729861251857, -63.89295307432605853 ) ) ;
#4853=CARTESIAN_POINT ( 'NONE',  ( 4.294655364005415699, 16.66518840966061887, -58.95704692567386473 ) ) ;
#4865=CARTESIAN_POINT ( 'NONE',  ( 1.887862790868997109, 13.79486065368817194, -45.89999999999997016 ) ) ;
#4878=CARTESIAN_POINT ( 'NONE',  ( -4.342430937695320736, 18.03316848959025620, -75.44295307432606990 ) ) ;
#4893=CARTESIAN_POINT ( 'NONE',  ( 4.107178604518054499, 18.15051318458946383, -36.29999999999996163 ) ) ;
#4898=CARTESIAN_POINT ( 'NONE',  ( 3.091735541773220852, 14.40826445822673563, -39.74999999999996447 ) ) ;
#4906=CARTESIAN_POINT ( 'NONE',  ( 4.107178604518054499, 18.15051318458946383, -69.29999999999996874 ) ) ;
#4909=CARTESIAN_POINT ( 'NONE',  ( -4.975717084895059372, 20.19824746994243370, -42.60704692567387752 ) ) ;
#4910=CARTESIAN_POINT ( 'NONE',  ( 0.9307174358028527106, 11.62368137996505801, -37.04999999999996163 ) ) ;
#4922=CARTESIAN_POINT ( 'NONE',  ( -5.852430833189966819, 18.58153898617744915, -39.45704692567387184 ) ) ;
#4925=CARTESIAN_POINT ( 'NONE',  ( -2.698247469942396837, 22.47571708489507358, -48.89295307432605853 ) ) ;
#4944=CARTESIAN_POINT ( 'NONE',  ( 3.898383833589191383, 21.60376697729997275, -73.49295307432603863 ) ) ;
#4947=CARTESIAN_POINT ( 'NONE',  ( 0.5331684895902240040, 13.15756906230466328, -41.55704692567387326 ) ) ;
#4948=CARTESIAN_POINT ( 'NONE',  ( 3.091735541773220852, 14.40826445822673563, -60.74999999999995737 ) ) ;
#4958=CARTESIAN_POINT ( 'NONE',  ( -0.5331684895902242260, 21.84243093769531185, -40.05704692567387326 ) ) ;
#4959=CARTESIAN_POINT ( 'NONE',  ( 2.568848540478311460, 12.45835086740561692, -66.89999999999997726 ) ) ;
#4971=CARTESIAN_POINT ( 'NONE',  ( 2.837105286290961370, 22.73177855326409613, -61.35704692567387752 ) ) ;
#4975=CARTESIAN_POINT ( 'NONE',  ( 5.588711115410763597, 18.38516488214980882, -27.29999999999996163 ) ) ;
#4992=CARTESIAN_POINT ( 'NONE',  ( 0.8851648821498760977, 23.08871111541074228, -47.69999999999996732 ) ) ;
#4996=CARTESIAN_POINT ( 'NONE',  ( 3.091735541773220852, 14.40826445822673563, -27.74999999999995381 ) ) ;
#4997=CARTESIAN_POINT ( 'NONE',  ( -0.6839900399647738105, 21.81854315085035623, -65.54999999999996874 ) ) ;
#5008=CARTESIAN_POINT ( 'NONE',  ( -4.342430937695320736, 18.03316848959025620, -39.44295307432604858 ) ) ;
#5011=CARTESIAN_POINT ( 'NONE',  ( 3.826489000663266360, 19.62107449533211678, -55.64295307432606563 ) ) ;
#5027=CARTESIAN_POINT ( 'NONE',  ( 5.041649132594343996, 14.93115145952162415, -54.59999999999996589 ) ) ;
#5049=CARTESIAN_POINT ( 'NONE',  ( -5.900206406879871857, 18.27989588542834554, -54.44295307432606990 ) ) ;
#5059=CARTESIAN_POINT ( 'NONE',  ( -3.199711850326840246, 20.48375923321962233, -66.74295307432606705 ) ) ;
#5061=CARTESIAN_POINT ( 'NONE',  ( 2.983759233219601459, 14.30028814967311668, -53.25704692567386900 ) ) ;
#5074=CARTESIAN_POINT ( 'NONE',  ( -3.705139346311794313, 19.38786279086902198, -41.09999999999996589 ) ) ;
#5086=CARTESIAN_POINT ( 'NONE',  ( -2.837723661809363751, 14.45689319447982335, -74.99295307432603863 ) ) ;
#5100=CARTESIAN_POINT ( 'NONE',  ( 4.107178604518054499, 18.15051318458946383, -42.29999999999996874 ) ) ;
#5105=CARTESIAN_POINT ( 'NONE',  ( -3.895814058185739448, 15.51498359085620571, -31.64999999999995950 ) ) ;
#5115=CARTESIAN_POINT ( 'NONE',  ( 4.107178604518054499, 18.15051318458946383, -60.29999999999996163 ) ) ;
#5117=CARTESIAN_POINT ( 'NONE',  ( -5.370428668309080500, 14.93501088608579153, -42.15704692567387468 ) ) ;
#5118=CARTESIAN_POINT ( 'NONE',  ( -5.041649132594344884, 20.06884854047834921, -38.09999999999996589 ) ) ;
#5119=CARTESIAN_POINT ( 'NONE',  ( 5.231778553264135212, 20.33710528629089254, -40.64295307432606563 ) ) ;
#5122=CARTESIAN_POINT ( 'NONE',  ( -2.837723661809363751, 14.45689319447982335, -26.99295307432605995 ) ) ;
#5133=CARTESIAN_POINT ( 'NONE',  ( 4.099003336600150149, 13.18504404629255689, -32.25704692567387610 ) ) ;
#5138=CARTESIAN_POINT ( 'NONE',  ( 5.565992480072003978, 18.52860470043125574, -46.79295307432605711 ) ) ;
#5159=CARTESIAN_POINT ( 'NONE',  ( 0.7417250638684235176, 23.11142975074950101, -73.19295307432605568 ) ) ;
#5162=CARTESIAN_POINT ( 'NONE',  ( 3.965139115708213868, 19.34895832295540430, -40.65704692567387468 ) ) ;
#5163=CARTESIAN_POINT ( 'NONE',  ( -1.887862790868997553, 21.20513934631180319, -38.39999999999997016 ) ) ;
#5164=CARTESIAN_POINT ( 'NONE',  ( 1.887862790868997109, 13.79486065368817194, -63.89999999999997016 ) ) ;
#5175=CARTESIAN_POINT ( 'NONE',  ( 2.837105286290961370, 22.73177855326409613, -73.35704692567385621 ) ) ;
#5176=CARTESIAN_POINT ( 'NONE',  ( -4.206979645153769098, 21.70697964515380107, -68.24999999999995737 ) ) ;
#5186=CARTESIAN_POINT ( 'NONE',  ( -1.028604700431329233, 11.93400751992799513, -59.70704692567387184 ) ) ;
#5190=CARTESIAN_POINT ( 'NONE',  ( -4.001075405444606936, 13.49892459455542060, -25.49999999999996803 ) ) ;
#5205=CARTESIAN_POINT ( 'NONE',  ( -2.568848540478311904, 22.54164913259435465, -56.39999999999996305 ) ) ;
#5209=CARTESIAN_POINT ( 'NONE',  ( 0.7939530028709752552, 21.58445996917927445, -70.20704692567387895 ) ) ;
#5210=CARTESIAN_POINT ( 'NONE',  ( -2.940415233664778860, 14.55958476633523802, -61.49999999999997158 ) ) ;
#5221=CARTESIAN_POINT ( 'NONE',  ( -4.342430937695320736, 18.03316848959025620, -33.44295307432605568 ) ) ;
#5224=CARTESIAN_POINT ( 'NONE',  ( 4.342430937695320736, 16.96683151040971538, -49.94295307432606279 ) ) ;
#5240=CARTESIAN_POINT ( 'NONE',  ( -2.568848540478311904, 22.54164913259435465, -56.39999999999996305 ) ) ;
#5260=CARTESIAN_POINT ( 'NONE',  ( 0.7417250638684235176, 23.11142975074950101, -49.19295307432605568 ) ) ;
#5269=CARTESIAN_POINT ( 'NONE',  ( -3.771071394011080269, 19.25846386140493394, -66.59295307432604716 ) ) ;
#5283=CARTESIAN_POINT ( 'NONE',  ( -4.107178604518053611, 16.84948681541050775, -49.79999999999996874 ) ) ;
#5308=CARTESIAN_POINT ( 'NONE',  ( 3.705139346311793869, 15.61213720913094960, -39.59999999999996589 ) ) ;
#5312=CARTESIAN_POINT ( 'NONE',  ( 2.940415233664778416, 20.44041523366473712, -32.99999999999996447 ) ) ;
#5320=CARTESIAN_POINT ( 'NONE',  ( 3.895814058185739448, 19.48501640914375344, -54.14999999999997726 ) ) ;
#5322=CARTESIAN_POINT ( 'NONE',  ( 5.611429750749524992, 18.24172506386835479, -46.80704692567388037 ) ) ;
#5323=CARTESIAN_POINT ( 'NONE',  ( -5.876318620034919782, 18.43071743580290089, -37.94999999999996021 ) ) ;
#5326=CARTESIAN_POINT ( 'NONE',  ( -4.318543150850367773, 18.18399003996480801, -73.94999999999997442 ) ) ;
#5335=CARTESIAN_POINT ( 'NONE',  ( -4.099003336600151925, 21.81495595370741469, -30.75704692567387610 ) ) ;
#5341=CARTESIAN_POINT ( 'NONE',  ( -5.107581180293630396, 19.93944961101426827, -48.59295307432606847 ) ) ;
#5357=CARTESIAN_POINT ( 'NONE',  ( 5.565992480072003978, 18.52860470043125574, -70.79295307432605000 ) ) ;
#5361=CARTESIAN_POINT ( 'NONE',  ( -1.758463861404912842, 21.27107139401109137, -39.90704692567386758 ) ) ;
#5362=CARTESIAN_POINT ( 'NONE',  ( 4.318543150850367773, 16.81600996003516357, -30.44999999999995310 ) ) ;
#5363=CARTESIAN_POINT ( 'NONE',  ( 3.705139346311793869, 15.61213720913094960, -63.59999999999995879 ) ) ;
#5374=CARTESIAN_POINT ( 'NONE',  ( -5.852430833189966819, 18.58153898617744915, -72.45704692567387895 ) ) ;
#5375=CARTESIAN_POINT ( 'NONE',  ( -2.568848540478311904, 22.54164913259435465, -62.39999999999997016 ) ) ;
#5388=CARTESIAN_POINT ( 'NONE',  ( -5.370428668309080500, 14.93501088608579153, -66.15704692567388179 ) ) ;
#5393=CARTESIAN_POINT ( 'NONE',  ( -0.9307174358028533767, 23.37631862003491889, -32.54999999999996163 ) ) ;
#5411=CARTESIAN_POINT ( 'NONE',  ( 5.588711115410763597, 18.38516488214980882, -48.29999999999996874 ) ) ;
#5415=CARTESIAN_POINT ( 'NONE',  ( -0.7939530028709754772, 13.41554003082070246, -71.70704692567387895 ) ) ;
#5416=CARTESIAN_POINT ( 'NONE',  ( -4.107178604518053611, 16.84948681541050775, -58.79999999999996163 ) ) ;
#5422=CARTESIAN_POINT ( 'NONE',  ( -4.318543150850367773, 18.18399003996480801, -70.94999999999997442 ) ) ;
#5427=CARTESIAN_POINT ( 'NONE',  ( -2.837723661809363751, 14.45689319447982335, -35.99295307432605995 ) ) ;
#5431=CARTESIAN_POINT ( 'NONE',  ( -3.826489000663265472, 15.37892550466785480, -51.14295307432606563 ) ) ;
#5447=CARTESIAN_POINT ( 'NONE',  ( -0.9307174358028533767, 23.37631862003491889, -62.54999999999996874 ) ) ;
#5468=CARTESIAN_POINT ( 'NONE',  ( 4.314955953707388936, 13.40099666339979123, -47.24295307432605995 ) ) ;
#5470=PRODUCT_DEFINITION_SHAPE ( 'NONE', 'NONE',  #19506 ) ;
#5479=CARTESIAN_POINT ( 'NONE',  ( 2.017261720333081598, 13.86079270138745834, -65.39295307432605853 ) ) ;
#5493=CARTESIAN_POINT ( 'NONE',  ( -2.940415233664778860, 14.55958476633523802, -49.49999999999996447 ) ) ;
#5520=CARTESIAN_POINT ( 'NONE',  ( -1.887862790868997553, 21.20513934631180319, -26.39999999999996660 ) ) ;
#5524=CARTESIAN_POINT ( 'NONE',  ( 4.318543150850367773, 16.81600996003516357, -36.44999999999996732 ) ) ;
#5534=CARTESIAN_POINT ( 'NONE',  ( -3.895814058185739448, 15.51498359085620571, -52.64999999999997016 ) ) ;
#5536=CARTESIAN_POINT ( 'NONE',  ( 5.852430833189966819, 16.41846101382252243, -43.95704692567387184 ) ) ;
#5537=CARTESIAN_POINT ( 'NONE',  ( -5.588711115410763597, 16.61483511785016987, -31.79999999999996874 ) ) ;
#5539=CARTESIAN_POINT ( 'NONE',  ( -1.985016409143819605, 13.60418594181426855, -70.34999999999993747 ) ) ;
#5551=CARTESIAN_POINT ( 'NONE',  ( -4.099003336600151925, 21.81495595370741469, -27.75704692567387255 ) ) ;
#5556=CARTESIAN_POINT ( 'NONE',  ( -3.898383833589191827, 13.39623302270000771, -44.99295307432606705 ) ) ;
#5573=CARTESIAN_POINT ( 'NONE',  ( -5.231778553264134324, 14.66289471370907727, -72.14295307432605853 ) ) ;
#5579=CARTESIAN_POINT ( 'NONE',  ( 2.940415233664778416, 20.44041523366473712, -32.99999999999996447 ) ) ;
#5581=CARTESIAN_POINT ( 'NONE',  ( 1.985016409143818272, 21.39581405818570303, -59.84999999999996589 ) ) ;
#5592=CARTESIAN_POINT ( 'NONE',  ( 2.439449611014226971, 12.39241881970633230, -71.40704692567388179 ) ) ;
#5593=CARTESIAN_POINT ( 'NONE',  ( 4.001075405444606048, 21.50107540544455276, -65.99999999999997158 ) ) ;
#5603=CARTESIAN_POINT ( 'NONE',  ( 2.837105286290961370, 22.73177855326409613, -55.35704692567387752 ) ) ;
#5610=CARTESIAN_POINT ( 'NONE',  ( -5.588711115410763597, 16.61483511785016987, -31.79999999999996874 ) ) ;
#5625=CARTESIAN_POINT ( 'NONE',  ( -4.206979645153768210, 21.70697964515380107, -56.24999999999995026 ) ) ;
#5629=CARTESIAN_POINT ( 'NONE',  ( 2.121074495332174958, 21.32648900066323350, -70.35704692567388463 ) ) ;
#5630=CARTESIAN_POINT ( 'NONE',  ( -3.091735541773221296, 20.59173554177323950, -62.24999999999996447 ) ) ;
#5638=CARTESIAN_POINT ( 'NONE',  ( -4.318543150850367773, 18.18399003996480801, -73.94999999999997442 ) ) ;
#5643=CARTESIAN_POINT ( 'NONE',  ( -0.8348115903393239501, 21.79465536400541126, -31.04295307432605355 ) ) ;
#5647=CARTESIAN_POINT ( 'NONE',  ( 0.8348115903393232839, 13.20534463599456387, -44.54295307432605711 ) ) ;
#5661=CARTESIAN_POINT ( 'NONE',  ( -5.041649132594344884, 20.06884854047834921, -59.09999999999997300 ) ) ;
#5686=CARTESIAN_POINT ( 'NONE',  ( -5.565992480072003978, 16.47139529956871229, -42.29295307432605711 ) ) ;
#5693=CARTESIAN_POINT ( 'NONE',  ( 4.084459969179292216, 18.29395300287091430, -61.79295307432605000 ) ) ;
#5708=CARTESIAN_POINT ( 'NONE',  ( -0.6839900399647736995, 21.81854315085035623, -47.54999999999997584 ) ) ;
#5734=CARTESIAN_POINT ( 'NONE',  ( 2.940415233664778416, 20.44041523366473712, -29.99999999999996447 ) ) ;
#5739=CARTESIAN_POINT ( 'NONE',  ( -1.985016409143819605, 13.60418594181426855, -28.34999999999995524 ) ) ;
#5747=CARTESIAN_POINT ( 'NONE',  ( 3.705139346311793869, 15.61213720913094960, -54.59999999999996589 ) ) ;
#5749=CARTESIAN_POINT ( 'NONE',  ( -2.837105286290963146, 12.26822144673588255, -44.85704692567387752 ) ) ;
#5750=CARTESIAN_POINT ( 'NONE',  ( 0.8851648821498760977, 23.08871111541074228, -26.69999999999996732 ) ) ;
#5751=CARTESIAN_POINT ( 'NONE',  ( 2.837723661809363307, 20.54310680552015356, -28.49295307432605995 ) ) ;
#5762=CARTESIAN_POINT ( 'NONE',  ( 2.837105286290961370, 22.73177855326409613, -28.35704692567387397 ) ) ;
#5768=CARTESIAN_POINT ( 'NONE',  ( -5.565992480072003978, 16.47139529956871229, -39.29295307432605711 ) ) ;
#5787=CARTESIAN_POINT ( 'NONE',  ( -4.314955953707389824, 21.59900333660018390, -66.74295307432606705 ) ) ;
#5792=CARTESIAN_POINT ( 'NONE',  ( -4.107178604518053611, 16.84948681541050775, -37.79999999999996874 ) ) ;
#5793=CARTESIAN_POINT ( 'NONE',  ( 1.887862790868997109, 13.79486065368817194, -66.89999999999997726 ) ) ;
#5804=CARTESIAN_POINT ( 'NONE',  ( -3.965139115708213868, 15.65104167704456906, -27.15704692567387823 ) ) ;
#5805=CARTESIAN_POINT ( 'NONE',  ( 2.701047200102605128, 22.80110361078656211, -68.84999999999996589 ) ) ;
#5816=CARTESIAN_POINT ( 'NONE',  ( -0.7798958854283041253, 23.40020640687986386, -55.05704692567387326 ) ) ;
#5819=CARTESIAN_POINT ( 'NONE',  ( 3.898383833589191383, 21.60376697729997275, -73.49295307432603863 ) ) ;
#5836=CARTESIAN_POINT ( 'NONE',  ( 5.301103610786608300, 20.20104720010253985, -54.14999999999997726 ) ) ;
#5840=CARTESIAN_POINT ( 'NONE',  ( 4.129897239856814117, 18.00707336630801336, -61.80704692567387326 ) ) ;
#5841=CARTESIAN_POINT ( 'NONE',  ( 3.705139346311793869, 15.61213720913094960, -54.59999999999996589 ) ) ;
#5849=CARTESIAN_POINT ( 'NONE',  ( 3.091735541773220852, 14.40826445822673563, -69.74999999999997158 ) ) ;
#5851=CARTESIAN_POINT ( 'NONE',  ( 0.7939530028709752552, 21.58445996917927445, -52.20704692567388605 ) ) ;
#5854=CARTESIAN_POINT ( 'NONE',  ( -3.895814058185739448, 15.51498359085620571, -70.64999999999996305 ) ) ;
#5857=CARTESIAN_POINT ( 'NONE',  ( 4.084459969179292216, 18.29395300287091430, -46.79295307432605711 ) ) ;
#5871=CARTESIAN_POINT ( 'NONE',  ( 4.001075405444606048, 21.50107540544455276, -47.99999999999996447 ) ) ;
#5890=CARTESIAN_POINT ( 'NONE',  ( -3.091735541773221296, 20.59173554177323950, -47.24999999999995026 ) ) ;
#5891=CARTESIAN_POINT ( 'NONE',  ( -3.898383833589191827, 13.39623302270000771, -44.99295307432606705 ) ) ;
#5899=CARTESIAN_POINT ( 'NONE',  ( 0.8348115903393232839, 13.20534463599456387, -59.54295307432605711 ) ) ;
#5917=CARTESIAN_POINT ( 'NONE',  ( 4.107178604518054499, 18.15051318458946383, -39.29999999999996874 ) ) ;
#5938=CARTESIAN_POINT ( 'NONE',  ( 0.6839900399647732554, 13.18145684914961357, -28.04999999999996163 ) ) ;
#5941=CARTESIAN_POINT ( 'NONE',  ( -3.898383833589191827, 13.39623302270000771, -29.99295307432605640 ) ) ;
#5942=CARTESIAN_POINT ( 'NONE',  ( 4.107178604518054499, 18.15051318458946383, -27.29999999999996163 ) ) ;
#5951=CARTESIAN_POINT ( 'NONE',  ( 1.887862790868997109, 13.79486065368817194, -54.89999999999996305 ) ) ;
#5954=CARTESIAN_POINT ( 'NONE',  ( -1.028604700431329233, 11.93400751992799513, -32.70704692567387184 ) ) ;
#5955=CARTESIAN_POINT ( 'NONE',  ( 5.588711115410763597, 18.38516488214980882, -30.29999999999996518 ) ) ;
#5956=CARTESIAN_POINT ( 'NONE',  ( 1.985016409143818272, 21.39581405818570303, -62.84999999999995879 ) ) ;
#5967=CARTESIAN_POINT ( 'NONE',  ( 2.439449611014226971, 12.39241881970633230, -26.40704692567387823 ) ) ;
#5972=CARTESIAN_POINT ( 'NONE',  ( 4.314955953707388936, 13.40099666339979123, -38.24295307432604574 ) ) ;
#5990=CARTESIAN_POINT ( 'NONE',  ( -0.7417250638684240727, 11.88857024925047057, -62.69295307432606279 ) ) ;
#5995=CARTESIAN_POINT ( 'NONE',  ( -3.705139346311794313, 19.38786279086902198, -29.09999999999996589 ) ) ;
#5996=CARTESIAN_POINT ( 'NONE',  ( -2.940415233664778860, 14.55958476633523802, -58.49999999999997158 ) ) ;
#6006=CARTESIAN_POINT ( 'NONE',  ( -5.852430833189966819, 18.58153898617744915, -63.45704692567386473 ) ) ;
#6007=CARTESIAN_POINT ( 'NONE',  ( 5.876318620034919782, 16.56928256419707068, -51.44999999999996732 ) ) ;
#6020=CARTESIAN_POINT ( 'NONE',  ( 1.028604700431328567, 23.06599248007198355, -58.20704692567387184 ) ) ;
#6023=CARTESIAN_POINT ( 'NONE',  ( 5.565992480072003978, 18.52860470043125574, -73.79295307432605000 ) ) ;
#6040=CARTESIAN_POINT ( 'NONE',  ( -2.568848540478311904, 22.54164913259435465, -41.39999999999996305 ) ) ;
#6044=CARTESIAN_POINT ( 'NONE',  ( 4.294655364005415699, 16.66518840966061887, -64.95704692567387895 ) ) ;
#6045=CARTESIAN_POINT ( 'NONE',  ( 1.985016409143818272, 21.39581405818570659, -47.84999999999995168 ) ) ;
#6052=CARTESIAN_POINT ( 'NONE',  ( -3.895814058185739448, 15.51498359085620571, -67.64999999999997726 ) ) ;
#6054=CARTESIAN_POINT ( 'NONE',  ( 3.639207298612508801, 15.48273827966686866, -53.10704692567387752 ) ) ;
#6057=CARTESIAN_POINT ( 'NONE',  ( -0.5070733663080690956, 13.37010276014318144, -29.69295307432606279 ) ) ;
#6060=CARTESIAN_POINT ( 'NONE',  ( 1.848958322955461808, 21.46513911570817612, -43.34295307432605426 ) ) ;
#6073=CARTESIAN_POINT ( 'NONE',  ( -5.301103610786608300, 14.79895279989743706, -49.64999999999995595 ) ) ;
#6089=CARTESIAN_POINT ( 'NONE',  ( 4.206979645153767322, 13.29302035484617051, -66.74999999999997158 ) ) ;
#6094=CARTESIAN_POINT ( 'NONE',  ( 4.107178604518054499, 18.15051318458946383, -39.29999999999996874 ) ) ;
#6095=CARTESIAN_POINT ( 'NONE',  ( 5.107581180293630396, 15.06055038898570686, -41.09295307432606137 ) ) ;
#6104=CARTESIAN_POINT ( 'NONE',  ( 2.017261720333081598, 13.86079270138745834, -53.39295307432605853 ) ) ;
#6121=CARTESIAN_POINT ( 'NONE',  ( -0.6505131845895224529, 13.39282139548194195, -37.19999999999996732 ) ) ;
#6131=ADVANCED_BREP_SHAPE_REPRESENTATION ( '', ( #24407, #40442 ), #33653 ) ;
#6148=CARTESIAN_POINT ( 'NONE',  ( -1.758463861404912842, 21.27107139401109137, -30.90704692567387113 ) ) ;
#6149=CARTESIAN_POINT ( 'NONE',  ( -3.705139346311794313, 19.38786279086902198, -32.09999999999996589 ) ) ;
#6153=CARTESIAN_POINT ( 'NONE',  ( 2.564989113914249330, 22.87042866830903876, -34.34295307432605426 ) ) ;
#6154=CARTESIAN_POINT ( 'NONE',  ( 2.940415233664778416, 20.44041523366473712, -26.99999999999996803 ) ) ;
#6163=CARTESIAN_POINT ( 'NONE',  ( -0.6839900399647736995, 21.81854315085035623, -50.54999999999996163 ) ) ;
#6166=CARTESIAN_POINT ( 'NONE',  ( 4.099003336600150149, 13.18504404629255689, -35.25704692567386900 ) ) ;
#6167=CARTESIAN_POINT ( 'NONE',  ( 0.9307174358028527106, 11.62368137996505801, -28.04999999999996163 ) ) ;
#6168=CARTESIAN_POINT ( 'NONE',  ( 1.887862790868997109, 13.79486065368817194, -63.89999999999997016 ) ) ;
#6174=( NAMED_UNIT ( * ) PLANE_ANGLE_UNIT ( ) SI_UNIT ( $, .RADIAN. ) );
#6179=CARTESIAN_POINT ( 'NONE',  ( -2.701047200102606016, 12.19889638921340413, -73.34999999999996589 ) ) ;
#6183=CARTESIAN_POINT ( 'NONE',  ( -0.7417250638684240727, 11.88857024925047057, -44.69295307432606279 ) ) ;
#6200=CARTESIAN_POINT ( 'NONE',  ( -3.898383833589191827, 13.39623302270000771, -59.99295307432606705 ) ) ;
#6206=CARTESIAN_POINT ( 'NONE',  ( 1.985016409143818272, 21.39581405818570303, -29.84999999999996589 ) ) ;
#6207=CARTESIAN_POINT ( 'NONE',  ( -0.6839900399647736995, 21.81854315085035623, -56.54999999999996874 ) ) ;
#6218=CARTESIAN_POINT ( 'NONE',  ( 5.370428668309080500, 20.06498911391418360, -61.65704692567387468 ) ) ;
#6219=CARTESIAN_POINT ( 'NONE',  ( -5.876318620034919782, 18.43071743580290089, -55.94999999999997442 ) ) ;
#6229=CARTESIAN_POINT ( 'NONE',  ( 4.099003336600150149, 13.18504404629255689, -59.25704692567388321 ) ) ;
#6234=CARTESIAN_POINT ( 'NONE',  ( -2.698247469942396837, 22.47571708489507358, -72.89295307432605853 ) ) ;
#6251=CARTESIAN_POINT ( 'NONE',  ( 4.206979645153767322, 13.29302035484617051, -42.74999999999996447 ) ) ;
#6256=CARTESIAN_POINT ( 'NONE',  ( -3.639207298612509689, 19.51726172033310647, -66.60704692567387042 ) ) ;
#6257=CARTESIAN_POINT ( 'NONE',  ( -3.895814058185739892, 15.51498359085620748, -46.64999999999996305 ) ) ;
#6267=CARTESIAN_POINT ( 'NONE',  ( -4.318543150850367773, 18.18399003996480801, -67.94999999999994600 ) ) ;
#6269=CARTESIAN_POINT ( 'NONE',  ( 0.5331684895902240040, 13.15756906230466328, -41.55704692567387326 ) ) ;
#6287=CARTESIAN_POINT ( 'NONE',  ( 5.588711115410763597, 18.38516488214980882, -48.29999999999996874 ) ) ;
#6301=CARTESIAN_POINT ( 'NONE',  ( 0.8851648821498760977, 23.08871111541074228, -68.69999999999997442 ) ) ;
#6306=CARTESIAN_POINT ( 'NONE',  ( -0.6505131845895224529, 13.39282139548194195, -40.19999999999996732 ) ) ;
#6318=CARTESIAN_POINT ( 'NONE',  ( -3.199711850326840246, 20.48375923321962233, -51.74295307432605995 ) ) ;
#6334=CARTESIAN_POINT ( 'NONE',  ( -4.107178604518053611, 16.84948681541050775, -40.79999999999996874 ) ) ;
#6359=CARTESIAN_POINT ( 'NONE',  ( 1.758463861404912620, 13.72892860598888731, -35.40704692567386758 ) ) ;
#6360=CARTESIAN_POINT ( 'NONE',  ( -4.318543150850366885, 18.18399003996480801, -31.94999999999995666 ) ) ;
#6363=CARTESIAN_POINT ( 'NONE',  ( 1.081538986177402295, 11.64756916681001186, -32.54295307432605711 ) ) ;
#6365=CARTESIAN_POINT ( 'NONE',  ( 4.129897239856814117, 18.00707336630801336, -70.80704692567387326 ) ) ;
#6374=CARTESIAN_POINT ( 'NONE',  ( 1.887862790868997109, 13.79486065368817194, -45.89999999999997016 ) ) ;
#6377=CARTESIAN_POINT ( 'NONE',  ( 5.852430833189966819, 16.41846101382252243, -40.95704692567387184 ) ) ;
#6378=CARTESIAN_POINT ( 'NONE',  ( 5.041649132594343996, 14.93115145952162415, -30.59999999999996589 ) ) ;
#6379=CARTESIAN_POINT ( 'NONE',  ( 1.887862790868997109, 13.79486065368817194, -66.89999999999997726 ) ) ;
#6391=CARTESIAN_POINT ( 'NONE',  ( -2.564989113914250662, 12.12957133169093282, -44.84295307432606137 ) ) ;
#6410=CARTESIAN_POINT ( 'NONE',  ( -5.900206406879871857, 18.27989588542834554, -66.44295307432605568 ) ) ;
#6416=CARTESIAN_POINT ( 'NONE',  ( 3.705139346311793869, 15.61213720913094960, -51.59999999999996589 ) ) ;
#6428=CARTESIAN_POINT ( 'NONE',  ( 5.611429750749524992, 18.24172506386835479, -70.80704692567387326 ) ) ;
#6429=CARTESIAN_POINT ( 'NONE',  ( 5.301103610786608300, 20.20104720010254340, -57.14999999999995595 ) ) ;
#6443=CARTESIAN_POINT ( 'NONE',  ( -2.837105286290963146, 12.26822144673588255, -53.85704692567387042 ) ) ;
#6446=CARTESIAN_POINT ( 'NONE',  ( -1.081538986177402961, 23.35243083318996327, -73.04295307432606421 ) ) ;
#6465=CARTESIAN_POINT ( 'NONE',  ( 2.568848540478311460, 12.45835086740561692, -39.89999999999996305 ) ) ;
#6469=CARTESIAN_POINT ( 'NONE',  ( 2.983759233219601459, 14.30028814967311668, -62.25704692567386900 ) ) ;
#6470=CARTESIAN_POINT ( 'NONE',  ( -0.6505131845895224529, 13.39282139548194195, -49.19999999999996732 ) ) ;
#6479=CARTESIAN_POINT ( 'NONE',  ( 1.887862790868997109, 13.79486065368817194, -60.89999999999997016 ) ) ;
#6481=CARTESIAN_POINT ( 'NONE',  ( -0.7939530028709754772, 13.41554003082070246, -44.70704692567387184 ) ) ;
#6486=CARTESIAN_POINT ( 'NONE',  ( -3.771071394011080269, 19.25846386140493394, -48.59295307432606847 ) ) ;
#6502=CARTESIAN_POINT ( 'NONE',  ( -4.001075405444606936, 13.49892459455542060, -43.49999999999997158 ) ) ;
#6517=CARTESIAN_POINT ( 'NONE',  ( -4.206979645153768210, 21.70697964515380107, -68.24999999999995737 ) ) ;
#6522=CARTESIAN_POINT ( 'NONE',  ( -1.887862790868997553, 21.20513934631180319, -47.39999999999997016 ) ) ;
#6523=CARTESIAN_POINT ( 'NONE',  ( -1.887862790868997553, 21.20513934631180319, -74.39999999999996305 ) ) ;
#6535=CARTESIAN_POINT ( 'NONE',  ( -2.017261720333081598, 21.13920729861251857, -54.89295307432605853 ) ) ;
#6574=CARTESIAN_POINT ( 'NONE',  ( -1.758463861404912842, 21.27107139401109137, -33.90704692567386758 ) ) ;
#6578=CARTESIAN_POINT ( 'NONE',  ( 0.7417250638684235176, 23.11142975074950101, -37.19295307432606279 ) ) ;
#6579=CARTESIAN_POINT ( 'NONE',  ( -3.091735541773221296, 20.59173554177323950, -29.24999999999996447 ) ) ;
#6586=CARTESIAN_POINT ( 'NONE',  ( 4.318543150850367773, 16.81600996003516357, -42.44999999999996732 ) ) ;
#6588=CARTESIAN_POINT ( 'NONE',  ( -4.975717084895059372, 20.19824746994243370, -36.60704692567387752 ) ) ;
#6589=CARTESIAN_POINT ( 'NONE',  ( -2.568848540478311904, 22.54164913259435465, -29.39999999999996660 ) ) ;
#6591=CARTESIAN_POINT ( 'NONE',  ( 0.6505131845895220088, 21.60717860451803674, -68.69999999999997442 ) ) ;
#6603=CARTESIAN_POINT ( 'NONE',  ( 5.231778553264135212, 20.33710528629089254, -28.64295307432606208 ) ) ;
#6622=CARTESIAN_POINT ( 'NONE',  ( -0.6839900399647736995, 21.81854315085035623, -29.54999999999996518 ) ) ;
#6623=CARTESIAN_POINT ( 'NONE',  ( 4.107178604518054499, 18.15051318458946383, -54.29999999999996874 ) ) ;
#6632=CARTESIAN_POINT ( 'NONE',  ( 1.028604700431328567, 23.06599248007198355, -64.20704692567387895 ) ) ;
#6633=CARTESIAN_POINT ( 'NONE',  ( 5.876318620034919782, 16.56928256419707068, -57.44999999999996021 ) ) ;
#6638=ORIENTED_EDGE ( 'NONE', *, *, #12300, .F. ) ;
#6646=CARTESIAN_POINT ( 'NONE',  ( 4.975717084895059372, 14.80175253005754143, -44.10704692567387752 ) ) ;
#6651=CARTESIAN_POINT ( 'NONE',  ( 3.898383833589191383, 21.60376697729997275, -67.49295307432606705 ) ) ;
#6664=CARTESIAN_POINT ( 'NONE',  ( -0.8851648821498765418, 11.91128888458923285, -43.19999999999996732 ) ) ;
#6668=CARTESIAN_POINT ( 'NONE',  ( 2.121074495332174958, 21.32648900066323350, -67.35704692567388463 ) ) ;
#6669=CARTESIAN_POINT ( 'NONE',  ( 1.985016409143818272, 21.39581405818570659, -44.84999999999996589 ) ) ;
#6678=CARTESIAN_POINT ( 'NONE',  ( -2.940415233664778860, 14.55958476633523802, -64.49999999999997158 ) ) ;
#6680=CARTESIAN_POINT ( 'NONE',  ( 0.7939530028709752552, 21.58445996917927445, -49.20704692567387184 ) ) ;
#6685=CARTESIAN_POINT ( 'NONE',  ( 3.771071394011080269, 15.74153613859503764, -32.09295307432605426 ) ) ;
#6692=CARTESIAN_POINT ( 'NONE',  ( -5.370428668309080500, 14.93501088608579153, -69.15704692567386758 ) ) ;
#6699=CARTESIAN_POINT ( 'NONE',  ( -0.8851648821498765418, 11.91128888458923285, -46.19999999999996021 ) ) ;
#6715=CARTESIAN_POINT ( 'NONE',  ( 5.041649132594343996, 14.93115145952162415, -69.59999999999996589 ) ) ;
#6720=CARTESIAN_POINT ( 'NONE',  ( 4.318543150850367773, 16.81600996003516357, -42.44999999999996732 ) ) ;
#6732=CARTESIAN_POINT ( 'NONE',  ( 3.771071394011080269, 15.74153613859503764, -47.09295307432606137 ) ) ;
#6738=CARTESIAN_POINT ( 'NONE',  ( -2.837723661809363751, 14.45689319447982335, -59.99295307432606705 ) ) ;
#6749=CARTESIAN_POINT ( 'NONE',  ( 4.107178604518054499, 18.15051318458946383, -36.29999999999996163 ) ) ;
#6776=CARTESIAN_POINT ( 'NONE',  ( 4.129897239856814117, 18.00707336630801336, -34.80704692567387326 ) ) ;
#6781=CARTESIAN_POINT ( 'NONE',  ( -1.081538986177402961, 23.35243083318996327, -34.04295307432605711 ) ) ;
#6782=CARTESIAN_POINT ( 'NONE',  ( 2.121074495332174958, 21.32648900066323350, -61.35704692567387752 ) ) ;
#6788=CARTESIAN_POINT ( 'NONE',  ( -0.6505131845895224529, 13.39282139548194195, -46.19999999999996021 ) ) ;
#6791=CARTESIAN_POINT ( 'NONE',  ( 4.975717084895059372, 14.80175253005754143, -41.10704692567387752 ) ) ;
#6793=CARTESIAN_POINT ( 'NONE',  ( 2.940415233664778416, 20.44041523366473712, -68.99999999999995737 ) ) ;
#6807=CARTESIAN_POINT ( 'NONE',  ( -4.314955953707389824, 21.59900333660018390, -36.74295307432605995 ) ) ;
#6815=ORIENTED_EDGE ( 'NONE', *, *, #19442, .F. ) ;
#6824=CARTESIAN_POINT ( 'NONE',  ( -1.887862790868997553, 21.20513934631180319, -50.39999999999996305 ) ) ;
#6833=CARTESIAN_POINT ( 'NONE',  ( -3.199711850326840246, 20.48375923321962233, -27.74295307432605995 ) ) ;
#6835=CARTESIAN_POINT ( 'NONE',  ( 1.028604700431328567, 23.06599248007198355, -67.20704692567387895 ) ) ;
#6836=CARTESIAN_POINT ( 'NONE',  ( 0.8851648821498760977, 23.08871111541074228, -53.69999999999996732 ) ) ;
#6851=CARTESIAN_POINT ( 'NONE',  ( 4.099003336600150149, 13.18504404629255689, -44.25704692567387610 ) ) ;
#6855=CARTESIAN_POINT ( 'NONE',  ( 2.698247469942395949, 12.52428291510489977, -65.39295307432605853 ) ) ;
#6872=CARTESIAN_POINT ( 'NONE',  ( 5.041649132594343996, 14.93115145952162415, -39.59999999999996589 ) ) ;
#6875=CARTESIAN_POINT ( 'NONE',  ( -0.5331684895902242260, 21.84243093769531185, -55.05704692567387326 ) ) ;
#6876=CARTESIAN_POINT ( 'NONE',  ( 4.318543150850366885, 16.81600996003516713, -48.44999999999996732 ) ) ;
#6883=CARTESIAN_POINT ( 'NONE',  ( -3.705139346311794313, 19.38786279086902198, -53.09999999999996589 ) ) ;
#6885=CARTESIAN_POINT ( 'NONE',  ( -3.043106805520194413, 14.66227633819065623, -42.00704692567387610 ) ) ;
#6890=CARTESIAN_POINT ( 'NONE',  ( 4.342430937695320736, 16.96683151040971538, -34.94295307432605568 ) ) ;
#6899=CARTESIAN_POINT ( 'NONE',  ( 4.103766977300021601, 21.39838383358913987, -73.50704692567386189 ) ) ;
#6906=CARTESIAN_POINT ( 'NONE',  ( 2.701047200102605572, 22.80110361078655856, -38.84999999999996589 ) ) ;
#6926=CARTESIAN_POINT ( 'NONE',  ( -5.301103610786608300, 14.79895279989743706, -70.64999999999996305 ) ) ;
#6931=CARTESIAN_POINT ( 'NONE',  ( 4.107178604518054499, 18.15051318458946383, -33.29999999999996874 ) ) ;
#6943=CARTESIAN_POINT ( 'NONE',  ( 1.848958322955461808, 21.46513911570817612, -46.34295307432606137 ) ) ;
#6949=CARTESIAN_POINT ( 'NONE',  ( -0.8348115903393239501, 21.79465536400541126, -67.04295307432605000 ) ) ;
#6953=ORIENTED_EDGE ( 'NONE', *, *, #28003, .T. ) ;
#6960=CARTESIAN_POINT ( 'NONE',  ( 3.705139346311793869, 15.61213720913094960, -27.59999999999996589 ) ) ;
#6970=CARTESIAN_POINT ( 'NONE',  ( -5.588711115410763597, 16.61483511785016987, -73.79999999999996874 ) ) ;
#6990=CARTESIAN_POINT ( 'NONE',  ( 3.639207298612508801, 15.48273827966686866, -35.10704692567387752 ) ) ;
#6994=CARTESIAN_POINT ( 'NONE',  ( 0.5070733663080689846, 21.62989723985679902, -76.19295307432606990 ) ) ;
#6995=CARTESIAN_POINT ( 'NONE',  ( 3.639207298612508801, 15.48273827966686866, -65.10704692567387042 ) ) ;
#7002=CARTESIAN_POINT ( 'NONE',  ( 0.6839900399647733664, 13.18145684914961357, -49.04999999999994742 ) ) ;
#7006=CARTESIAN_POINT ( 'NONE',  ( -4.103766977300021601, 13.60161616641083704, -30.00704692567387610 ) ) ;
#7009=CARTESIAN_POINT ( 'NONE',  ( -4.318543150850367773, 18.18399003996480801, -58.94999999999995310 ) ) ;
#7020=CARTESIAN_POINT ( 'NONE',  ( 5.900206406879871857, 16.72010411457162604, -34.94295307432605568 ) ) ;
#7039=CARTESIAN_POINT ( 'NONE',  ( 3.705139346311793869, 15.61213720913094960, -45.59999999999996589 ) ) ;
#7047=CARTESIAN_POINT ( 'NONE',  ( -0.6839900399647736995, 21.81854315085035623, -74.54999999999994031 ) ) ;
#7049=CARTESIAN_POINT ( 'NONE',  ( -1.028604700431329233, 11.93400751992799513, -59.70704692567387184 ) ) ;
#7050=CARTESIAN_POINT ( 'NONE',  ( -5.588711115410763597, 16.61483511785016987, -46.79999999999996874 ) ) ;
#7065=CARTESIAN_POINT ( 'NONE',  ( -4.975717084895059372, 20.19824746994243370, -48.60704692567386331 ) ) ;
#7070=CARTESIAN_POINT ( 'NONE',  ( 5.107581180293630396, 15.06055038898570686, -62.09295307432606847 ) ) ;
#7087=CARTESIAN_POINT ( 'NONE',  ( -5.041649132594344884, 20.06884854047834921, -32.09999999999996589 ) ) ;
#7090=CARTESIAN_POINT ( 'NONE',  ( -3.639207298612509689, 19.51726172033310647, -51.60704692567387752 ) ) ;
#7091=CARTESIAN_POINT ( 'NONE',  ( 3.895814058185739892, 19.48501640914376054, -36.14999999999996305 ) ) ;
#7093=CARTESIAN_POINT ( 'NONE',  ( -4.318543150850367773, 18.18399003996480801, -73.94999999999997442 ) ) ;
#7102=CARTESIAN_POINT ( 'NONE',  ( -1.985016409143819605, 13.60418594181426855, -55.34999999999997300 ) ) ;
#7104=CARTESIAN_POINT ( 'NONE',  ( 3.639207298612508801, 15.48273827966686866, -47.10704692567387042 ) ) ;
#7108=CARTESIAN_POINT ( 'NONE',  ( -2.837723661809363751, 14.45689319447982335, -32.99295307432605995 ) ) ;
#7115=CARTESIAN_POINT ( 'NONE',  ( 0.7939530028709752552, 21.58445996917927445, -25.20704692567387539 ) ) ;
#7123=CARTESIAN_POINT ( 'NONE',  ( 2.568848540478311460, 12.45835086740561692, -33.89999999999996305 ) ) ;
#7144=CARTESIAN_POINT ( 'NONE',  ( -0.8851648821498765418, 11.91128888458923285, -61.19999999999996732 ) ) ;
#7149=CARTESIAN_POINT ( 'NONE',  ( 2.940415233664778416, 20.44041523366473712, -32.99999999999996447 ) ) ;
#7150=CARTESIAN_POINT ( 'NONE',  ( 2.940415233664778416, 20.44041523366473712, -74.99999999999997158 ) ) ;
#7162=CARTESIAN_POINT ( 'NONE',  ( 2.837723661809363307, 20.54310680552015356, -43.49295307432606705 ) ) ;
#7167=CARTESIAN_POINT ( 'NONE',  ( 1.848958322955461808, 21.46513911570817612, -61.34295307432606137 ) ) ;
#7178=CARTESIAN_POINT ( 'NONE',  ( 1.985016409143818272, 21.39581405818570303, -29.84999999999996589 ) ) ;
#7187=CARTESIAN_POINT ( 'NONE',  ( 2.701047200102605572, 22.80110361078655856, -65.84999999999992326 ) ) ;
#7203=CARTESIAN_POINT ( 'NONE',  ( -5.107581180293630396, 19.93944961101426827, -66.59295307432604716 ) ) ;
#7213=CARTESIAN_POINT ( 'NONE',  ( 4.342430937695320736, 16.96683151040971538, -73.94295307432606990 ) ) ;
#7214=CARTESIAN_POINT ( 'NONE',  ( -0.5331684895902242260, 21.84243093769531185, -61.05704692567386616 ) ) ;
#7225=CARTESIAN_POINT ( 'NONE',  ( 4.099003336600150149, 13.18504404629255689, -26.25704692567387255 ) ) ;
#7227=CARTESIAN_POINT ( 'NONE',  ( 1.887862790868997109, 13.79486065368817194, -57.89999999999996305 ) ) ;
#7240=CARTESIAN_POINT ( 'NONE',  ( 5.565992480072003978, 18.52860470043125574, -28.79295307432605355 ) ) ;
#7257=CARTESIAN_POINT ( 'NONE',  ( -3.091735541773221296, 20.59173554177323950, -47.24999999999995026 ) ) ;
#7266=CARTESIAN_POINT ( 'NONE',  ( -3.705139346311794313, 19.38786279086902198, -65.09999999999996589 ) ) ;
#7269=CARTESIAN_POINT ( 'NONE',  ( 5.370428668309080500, 20.06498911391418360, -58.65704692567388179 ) ) ;
#7270=CARTESIAN_POINT ( 'NONE',  ( -2.568848540478311904, 22.54164913259435465, -47.39999999999997016 ) ) ;
#7283=CARTESIAN_POINT ( 'NONE',  ( -4.099003336600151925, 21.81495595370741469, -45.75704692567386900 ) ) ;
#7287=CARTESIAN_POINT ( 'NONE',  ( -4.314955953707389824, 21.59900333660018390, -57.74295307432607416 ) ) ;
#7300=CARTESIAN_POINT ( 'NONE',  ( -0.9307174358028533767, 23.37631862003491889, -32.54999999999996163 ) ) ;
#7303=CARTESIAN_POINT ( 'NONE',  ( -0.7939530028709754772, 13.41554003082070246, -53.70704692567388605 ) ) ;
#7304=CARTESIAN_POINT ( 'NONE',  ( -0.6839900399647738105, 21.81854315085035623, -38.54999999999996874 ) ) ;
#7305=CARTESIAN_POINT ( 'NONE',  ( 2.940415233664778416, 20.44041523366473712, -71.99999999999997158 ) ) ;
#7313=CARTESIAN_POINT ( 'NONE',  ( -4.318543150850367773, 18.18399003996480801, -52.94999999999994600 ) ) ;
#7316=CARTESIAN_POINT ( 'NONE',  ( 0.7939530028709752552, 21.58445996917927445, -34.20704692567387184 ) ) ;
#7317=CARTESIAN_POINT ( 'NONE',  ( -2.568848540478311904, 22.54164913259435465, -71.39999999999996305 ) ) ;
#7320=CARTESIAN_POINT ( 'NONE',  ( -3.826489000663265472, 15.37892550466785480, -33.14295307432605853 ) ) ;
#7327=CARTESIAN_POINT ( 'NONE',  ( 5.852430833189966819, 16.41846101382252243, -70.95704692567389316 ) ) ;
#7333=CARTESIAN_POINT ( 'NONE',  ( -5.041649132594344884, 20.06884854047834921, -41.09999999999996589 ) ) ;
#7349=CARTESIAN_POINT ( 'NONE',  ( 2.701047200102605572, 22.80110361078655856, -56.84999999999995879 ) ) ;
#7354=CARTESIAN_POINT ( 'NONE',  ( -1.887862790868997553, 21.20513934631180319, -32.39999999999996305 ) ) ;
#7355=CARTESIAN_POINT ( 'NONE',  ( 1.985016409143818272, 21.39581405818570659, -62.84999999999995879 ) ) ;
#7366=CARTESIAN_POINT ( 'NONE',  ( 1.848958322955461808, 21.46513911570817612, -43.34295307432605426 ) ) ;
#7371=CARTESIAN_POINT ( 'NONE',  ( 0.5070733663080689846, 21.62989723985679902, -64.19295307432605568 ) ) ;
#7381=CARTESIAN_POINT ( 'NONE',  ( -1.887862790868997553, 21.20513934631180319, -26.39999999999996660 ) ) ;
#7392=CARTESIAN_POINT ( 'NONE',  ( -0.9307174358028533767, 23.37631862003491889, -71.54999999999994031 ) ) ;
#7410=CARTESIAN_POINT ( 'NONE',  ( -3.898383833589191827, 13.39623302270000771, -50.99295307432605995 ) ) ;
#7420=CARTESIAN_POINT ( 'NONE',  ( -4.084459969179292216, 16.70604699712905372, -75.29295307432605000 ) ) ;
#7421=CARTESIAN_POINT ( 'NONE',  ( 1.758463861404912620, 13.72892860598888731, -62.40704692567388179 ) ) ;
#7433=CARTESIAN_POINT ( 'NONE',  ( 2.439449611014226971, 12.39241881970633230, -32.40704692567386758 ) ) ;
#7435=CARTESIAN_POINT ( 'NONE',  ( 3.705139346311793869, 15.61213720913094960, -57.59999999999997300 ) ) ;
#7448=CARTESIAN_POINT ( 'NONE',  ( 3.898383833589191383, 21.60376697729997275, -31.49295307432605995 ) ) ;
#7468=CARTESIAN_POINT ( 'NONE',  ( 3.705139346311793869, 15.61213720913094960, -48.59999999999996589 ) ) ;
#7478=CARTESIAN_POINT ( 'NONE',  ( -0.6505131845895224529, 13.39282139548194195, -67.19999999999997442 ) ) ;
#7480=CARTESIAN_POINT ( 'NONE',  ( 2.837105286290961370, 22.73177855326409613, -58.35704692567387752 ) ) ;
#7481=CARTESIAN_POINT ( 'NONE',  ( -5.041649132594344884, 20.06884854047834921, -41.09999999999996589 ) ) ;
#7493=CARTESIAN_POINT ( 'NONE',  ( -2.439449611014227859, 22.60758118029364283, -42.90704692567387468 ) ) ;
#7498=CARTESIAN_POINT ( 'NONE',  ( 2.698247469942395949, 12.52428291510489977, -62.39295307432605853 ) ) ;
#7515=CARTESIAN_POINT ( 'NONE',  ( -2.568848540478311904, 22.54164913259435465, -29.39999999999996660 ) ) ;
#7518=CARTESIAN_POINT ( 'NONE',  ( -0.7939530028709754772, 13.41554003082070246, -50.70704692567387184 ) ) ;
#7519=DIRECTION ( 'NONE',  ( -0.7037848285661852943, 0.7037848285661921777, 0.09681854243955874406 ) ) ;
#7528=CARTESIAN_POINT ( 'NONE',  ( 3.091735541773220852, 14.40826445822673563, -54.74999999999997158 ) ) ;
#7530=CARTESIAN_POINT ( 'NONE',  ( -1.758463861404912842, 21.27107139401109137, -39.90704692567386758 ) ) ;
#7531=CARTESIAN_POINT ( 'NONE',  ( -5.588711115410763597, 16.61483511785016987, -73.79999999999996874 ) ) ;
#7534=CARTESIAN_POINT ( 'NONE',  ( -4.084459969179292216, 16.70604699712905372, -33.29295307432605711 ) ) ;
#7539=CARTESIAN_POINT ( 'NONE',  ( 1.028604700431328567, 23.06599248007198355, -70.20704692567387895 ) ) ;
#7545=CARTESIAN_POINT ( 'NONE',  ( 0.8851648821498760977, 23.08871111541074228, -41.69999999999996732 ) ) ;
#7561=CARTESIAN_POINT ( 'NONE',  ( 2.701047200102605572, 22.80110361078655856, -59.84999999999996589 ) ) ;
#7566=CARTESIAN_POINT ( 'NONE',  ( -4.318543150850367773, 18.18399003996480801, -31.94999999999994955 ) ) ;
#7567=CARTESIAN_POINT ( 'NONE',  ( 0.6505131845895220088, 21.60717860451803674, -71.69999999999997442 ) ) ;
#7579=CARTESIAN_POINT ( 'NONE',  ( 4.084459969179292216, 18.29395300287091430, -43.79295307432606421 ) ) ;
#7584=CARTESIAN_POINT ( 'NONE',  ( 3.199711850326839357, 14.51624076678035635, -65.24295307432606705 ) ) ;
#7601=CARTESIAN_POINT ( 'NONE',  ( 0.9307174358028528216, 11.62368137996505801, -64.04999999999994031 ) ) ;
#7623=CARTESIAN_POINT ( 'NONE',  ( -4.314955953707389824, 21.59900333660018390, -57.74295307432607416 ) ) ;
#7631=CARTESIAN_POINT ( 'NONE',  ( 3.199711850326839357, 14.51624076678035635, -71.24295307432605284 ) ) ;
#7633=CARTESIAN_POINT ( 'NONE',  ( 4.129897239856814117, 18.00707336630801336, -67.80704692567387326 ) ) ;
#7645=CARTESIAN_POINT ( 'NONE',  ( -2.439449611014227859, 22.60758118029364283, -30.90704692567387113 ) ) ;
#7647=CARTESIAN_POINT ( 'NONE',  ( 3.895814058185739448, 19.48501640914375344, -57.14999999999995595 ) ) ;
#7663=CARTESIAN_POINT ( 'NONE',  ( -3.826489000663265472, 15.37892550466785480, -72.14295307432605853 ) ) ;
#7683=CARTESIAN_POINT ( 'NONE',  ( -4.318543150850367773, 18.18399003996480801, -46.94999999999996021 ) ) ;
#7691=CARTESIAN_POINT ( 'NONE',  ( -0.6839900399647736995, 21.81854315085035623, -65.54999999999996874 ) ) ;
#7693=CARTESIAN_POINT ( 'NONE',  ( -2.439449611014227859, 22.60758118029364283, -57.90704692567388179 ) ) ;
#7694=CARTESIAN_POINT ( 'NONE',  ( -0.9307174358028534877, 23.37631862003491889, -44.54999999999995453 ) ) ;
#7706=CARTESIAN_POINT ( 'NONE',  ( 2.837105286290961370, 22.73177855326409613, -37.35704692567387752 ) ) ;
#7712=CARTESIAN_POINT ( 'NONE',  ( -0.7417250638684240727, 11.88857024925047057, -59.69295307432605568 ) ) ;
#7729=CARTESIAN_POINT ( 'NONE',  ( -5.588711115410763597, 16.61483511785016987, -31.79999999999996874 ) ) ;
#7732=CARTESIAN_POINT ( 'NONE',  ( -2.121074495332175847, 13.67351099933674341, -53.85704692567387042 ) ) ;
#7733=CARTESIAN_POINT ( 'NONE',  ( -0.6839900399647736995, 21.81854315085035623, -74.54999999999994031 ) ) ;
#7741=CARTESIAN_POINT ( 'NONE',  ( 0.6839900399647733664, 13.18145684914961357, -55.04999999999995453 ) ) ;
#7744=CARTESIAN_POINT ( 'NONE',  ( -1.758463861404912842, 21.27107139401109137, -33.90704692567386758 ) ) ;
#7745=CARTESIAN_POINT ( 'NONE',  ( 4.206979645153768210, 13.29302035484617406, -72.74999999999995737 ) ) ;
#7757=CARTESIAN_POINT ( 'NONE',  ( -1.028604700431329233, 11.93400751992799513, -65.70704692567387895 ) ) ;
#7763=CARTESIAN_POINT ( 'NONE',  ( 4.206979645153767322, 13.29302035484617051, -42.74999999999996447 ) ) ;
#7780=CARTESIAN_POINT ( 'NONE',  ( -5.588711115410763597, 16.61483511785016987, -64.79999999999996874 ) ) ;
#7785=CARTESIAN_POINT ( 'NONE',  ( -4.107178604518053611, 16.84948681541050775, -37.79999999999996874 ) ) ;
#7786=CARTESIAN_POINT ( 'NONE',  ( -3.091735541773221296, 20.59173554177323950, -65.24999999999995737 ) ) ;
#7797=CARTESIAN_POINT ( 'NONE',  ( -3.771071394011080269, 19.25846386140493394, -33.59295307432606137 ) ) ;
#7802=CARTESIAN_POINT ( 'NONE',  ( -3.826489000663265472, 15.37892550466785480, -54.14295307432606563 ) ) ;
#7812=CARTESIAN_POINT ( 'NONE',  ( -3.895814058185739448, 15.51498359085620571, -31.64999999999995950 ) ) ;
#7822=CARTESIAN_POINT ( 'NONE',  ( -0.9307174358028533767, 23.37631862003491889, -68.54999999999998295 ) ) ;
#7841=CARTESIAN_POINT ( 'NONE',  ( 5.900206406879871857, 16.72010411457162604, -55.94295307432605568 ) ) ;
#7851=CARTESIAN_POINT ( 'NONE',  ( -5.231778553264134324, 14.66289471370907727, -27.14295307432605853 ) ) ;
#7853=CARTESIAN_POINT ( 'NONE',  ( 2.983759233219601459, 14.30028814967311668, -56.25704692567388321 ) ) ;
#7867=CARTESIAN_POINT ( 'NONE',  ( 1.985016409143818272, 21.39581405818570303, -59.84999999999996589 ) ) ;
#7877=CARTESIAN_POINT ( 'NONE',  ( 4.084459969179292216, 18.29395300287091430, -70.79295307432605000 ) ) ;
#7893=CARTESIAN_POINT ( 'NONE',  ( 1.985016409143818272, 21.39581405818570303, -44.84999999999996589 ) ) ;
#7903=CARTESIAN_POINT ( 'NONE',  ( 4.318543150850367773, 16.81600996003516357, -63.44999999999996732 ) ) ;
#7905=CARTESIAN_POINT ( 'NONE',  ( -4.975717084895059372, 20.19824746994243370, -60.60704692567387752 ) ) ;
#7906=CARTESIAN_POINT ( 'NONE',  ( -4.206979645153769098, 21.70697964515380107, -47.24999999999995737 ) ) ;
#7919=CARTESIAN_POINT ( 'NONE',  ( -4.975717084895059372, 20.19824746994243370, -39.60704692567387042 ) ) ;
#7924=CARTESIAN_POINT ( 'NONE',  ( 2.564989113914249330, 22.87042866830903876, -55.34295307432606137 ) ) ;
#7938=CARTESIAN_POINT ( 'NONE',  ( 5.041649132594343996, 14.93115145952162415, -36.59999999999996589 ) ) ;
#7942=CARTESIAN_POINT ( 'NONE',  ( -4.294655364005415699, 18.33481159033935626, -45.45704692567387184 ) ) ;
#7951=CARTESIAN_POINT ( 'NONE',  ( -2.940415233664778860, 14.55958476633523802, -49.49999999999996447 ) ) ;
#7954=CARTESIAN_POINT ( 'NONE',  ( 2.983759233219601459, 14.30028814967311668, -32.25704692567387610 ) ) ;
#7955=CARTESIAN_POINT ( 'NONE',  ( 2.701047200102605128, 22.80110361078656211, -74.84999999999995168 ) ) ;
#7964=CARTESIAN_POINT ( 'NONE',  ( -2.837105286290963146, 12.26822144673588255, -68.85704692567387042 ) ) ;
#7968=CARTESIAN_POINT ( 'NONE',  ( -0.9307174358028533767, 23.37631862003491889, -26.54999999999996163 ) ) ;
#7984=CARTESIAN_POINT ( 'NONE',  ( 2.701047200102605572, 22.80110361078655856, -62.84999999999995879 ) ) ;
#7987=CARTESIAN_POINT ( 'NONE',  ( 0.6839900399647733664, 13.18145684914961357, -28.04999999999995453 ) ) ;
#7988=CARTESIAN_POINT ( 'NONE',  ( 1.985016409143818272, 21.39581405818570659, -68.84999999999996589 ) ) ;
#8000=CARTESIAN_POINT ( 'NONE',  ( 3.199711850326839357, 14.51624076678035635, -35.24295307432605995 ) ) ;
#8005=CARTESIAN_POINT ( 'NONE',  ( 1.848958322955461808, 21.46513911570817612, -58.34295307432606137 ) ) ;
#8019=CARTESIAN_POINT ( 'NONE',  ( 4.001075405444606048, 21.50107540544455276, -53.99999999999996447 ) ) ;
#8039=CARTESIAN_POINT ( 'NONE',  ( -1.081538986177402961, 23.35243083318996327, -52.04295307432606421 ) ) ;
#8047=CARTESIAN_POINT ( 'NONE',  ( -1.848958322955462474, 13.53486088429179546, -65.84295307432604716 ) ) ;
#8049=CARTESIAN_POINT ( 'NONE',  ( 2.121074495332174958, 21.32648900066323350, -52.35704692567387042 ) ) ;
#8062=CARTESIAN_POINT ( 'NONE',  ( 0.6505131845895220088, 21.60717860451803674, -41.69999999999996732 ) ) ;
#8066=ORIENTED_EDGE ( 'NONE', *, *, #8142, .T. ) ;
#8072=CARTESIAN_POINT ( 'NONE',  ( 3.199711850326839357, 14.51624076678035635, -74.24295307432606705 ) ) ;
#8085=CARTESIAN_POINT ( 'NONE',  ( 0.6839900399647732554, 13.18145684914961357, -40.04999999999996163 ) ) ;
#8090=CARTESIAN_POINT ( 'NONE',  ( 0.6839900399647733664, 13.18145684914961357, -40.04999999999994742 ) ) ;
#8099=CARTESIAN_POINT ( 'NONE',  ( -0.6505131845895224529, 13.39282139548194195, -61.19999999999996732 ) ) ;
#8101=CARTESIAN_POINT ( 'NONE',  ( 4.099003336600150149, 13.18504404629255689, -47.25704692567386900 ) ) ;
#8102=CARTESIAN_POINT ( 'NONE',  ( -2.701047200102606460, 12.19889638921340591, -37.34999999999995879 ) ) ;
#8116=CARTESIAN_POINT ( 'NONE',  ( -2.439449611014227859, 22.60758118029364283, -33.90704692567386758 ) ) ;
#8120=CARTESIAN_POINT ( 'NONE',  ( 5.231778553264135212, 20.33710528629089254, -52.64295307432606563 ) ) ;
#8137=CARTESIAN_POINT ( 'NONE',  ( 5.301103610786608300, 20.20104720010253985, -27.14999999999995595 ) ) ;
#8141=CARTESIAN_POINT ( 'NONE',  ( -0.7939530028709754772, 13.41554003082070246, -41.70704692567387184 ) ) ;
#8142=EDGE_CURVE ( 'NONE', #2773, #4513, #30107, .T. ) ;
#8143=CARTESIAN_POINT ( 'NONE',  ( -4.318543150850367773, 18.18399003996480801, -67.94999999999994600 ) ) ;
#8151=APPLICATION_CONTEXT ( 'automotive_design' ) ;
#8153=CARTESIAN_POINT ( 'NONE',  ( -4.294655364005415699, 18.33481159033935626, -36.45704692567386473 ) ) ;
#8154=CARTESIAN_POINT ( 'NONE',  ( 5.588711115410763597, 18.38516488214980882, -66.29999999999996874 ) ) ;
#8164=CARTESIAN_POINT ( 'NONE',  ( 0.7798958854283032371, 11.59979359312010772, -68.55704692567387326 ) ) ;
#8167=CARTESIAN_POINT ( 'NONE',  ( 4.206979645153767322, 13.29302035484617051, -33.74999999999996447 ) ) ;
#8185=CARTESIAN_POINT ( 'NONE',  ( 4.001075405444606048, 21.50107540544455276, -47.99999999999996447 ) ) ;
#8188=CARTESIAN_POINT ( 'NONE',  ( 4.129897239856814117, 18.00707336630801336, -67.80704692567387326 ) ) ;
#8189=CARTESIAN_POINT ( 'NONE',  ( -3.705139346311794313, 19.38786279086902198, -68.09999999999996589 ) ) ;
#8201=CARTESIAN_POINT ( 'NONE',  ( -3.199711850326840246, 20.48375923321962233, -33.74295307432605995 ) ) ;
#8204=CARTESIAN_POINT ( 'NONE',  ( 3.771071394011080269, 15.74153613859503764, -56.09295307432605426 ) ) ;
#8220=CARTESIAN_POINT ( 'NONE',  ( 5.301103610786608300, 20.20104720010253985, -57.14999999999995595 ) ) ;
#8244=CARTESIAN_POINT ( 'NONE',  ( -1.081538986177402961, 23.35243083318996327, -58.04295307432605711 ) ) ;
#8252=CARTESIAN_POINT ( 'NONE',  ( 1.848958322955461808, 21.46513911570817612, -67.34295307432606137 ) ) ;
#8254=CARTESIAN_POINT ( 'NONE',  ( 0.5331684895902240040, 13.15756906230466328, -56.55704692567387326 ) ) ;
#8268=CARTESIAN_POINT ( 'NONE',  ( -4.318543150850367773, 18.18399003996480801, -46.94999999999996021 ) ) ;
#8281=CARTESIAN_POINT ( 'NONE',  ( -2.017261720333081598, 21.13920729861251857, -69.89295307432607274 ) ) ;
#8292=CARTESIAN_POINT ( 'NONE',  ( -3.705139346311794313, 19.38786279086902198, -35.09999999999996589 ) ) ;
#8297=CARTESIAN_POINT ( 'NONE',  ( 4.107178604518054499, 18.15051318458946383, -36.29999999999996163 ) ) ;
#8306=CARTESIAN_POINT ( 'NONE',  ( 4.318543150850367773, 16.81600996003516357, -51.44999999999997442 ) ) ;
#8308=CARTESIAN_POINT ( 'NONE',  ( 5.611429750749524992, 18.24172506386835479, -49.80704692567388037 ) ) ;
#8309=CARTESIAN_POINT ( 'NONE',  ( -5.301103610786608300, 14.79895279989743528, -37.64999999999997016 ) ) ;
#8312=CARTESIAN_POINT ( 'NONE',  ( 3.895814058185739448, 19.48501640914375344, -72.14999999999996305 ) ) ;
#8323=CARTESIAN_POINT ( 'NONE',  ( 0.7798958854283032371, 11.59979359312010772, -32.55704692567387326 ) ) ;
#8327=CARTESIAN_POINT ( 'NONE',  ( -5.900206406879871857, 18.27989588542834554, -48.44295307432605568 ) ) ;
#8343=CARTESIAN_POINT ( 'NONE',  ( 2.698247469942395949, 12.52428291510489977, -74.39295307432605853 ) ) ;
#8346=CARTESIAN_POINT ( 'NONE',  ( 0.5331684895902240040, 13.15756906230466328, -44.55704692567387326 ) ) ;
#8347=CARTESIAN_POINT ( 'NONE',  ( 4.107178604518054499, 18.15051318458946383, -33.29999999999996874 ) ) ;
#8348=CARTESIAN_POINT ( 'NONE',  ( -2.940415233664778860, 14.55958476633523802, -67.49999999999995737 ) ) ;
#8357=CARTESIAN_POINT ( 'NONE',  ( -3.965139115708213868, 15.65104167704456906, -24.15704692567387468 ) ) ;
#8358=CARTESIAN_POINT ( 'NONE',  ( -5.588711115410763597, 16.61483511785016987, -64.79999999999996874 ) ) ;
#8371=CARTESIAN_POINT ( 'NONE',  ( 4.975717084895059372, 14.80175253005754143, -68.10704692567387042 ) ) ;
#8375=CARTESIAN_POINT ( 'NONE',  ( -4.001075405444606936, 13.49892459455542060, -28.49999999999996447 ) ) ;
#8388=CLOSED_SHELL ( 'NONE', ( #21007, #13941, #21979, #19450 ) ) ;
#8389=CARTESIAN_POINT ( 'NONE',  ( -5.041649132594344884, 20.06884854047834921, -56.09999999999996589 ) ) ;
#8393=CARTESIAN_POINT ( 'NONE',  ( 1.887862790868997109, 13.79486065368817194, -27.89999999999996660 ) ) ;
#8394=CARTESIAN_POINT ( 'NONE',  ( -0.6839900399647738105, 21.81854315085035623, -53.54999999999996163 ) ) ;
#8400=CARTESIAN_POINT ( 'NONE',  ( -3.705139346311794313, 19.38786279086902198, -74.09999999999996589 ) ) ;
#8406=CARTESIAN_POINT ( 'NONE',  ( -3.771071394011080269, 19.25846386140493394, -39.59295307432606137 ) ) ;
#8409=CARTESIAN_POINT ( 'NONE',  ( -2.837723661809363751, 14.45689319447982335, -56.99295307432605995 ) ) ;
#8424=CARTESIAN_POINT ( 'NONE',  ( -2.568848540478311904, 22.54164913259435465, -59.39999999999997016 ) ) ;
#8447=CARTESIAN_POINT ( 'NONE',  ( -3.898383833589191827, 13.39623302270000771, -41.99295307432605995 ) ) ;
#8458=CARTESIAN_POINT ( 'NONE',  ( 0.8348115903393232839, 13.20534463599456387, -62.54295307432605711 ) ) ;
#8472=CARTESIAN_POINT ( 'NONE',  ( 3.705139346311793869, 15.61213720913094960, -42.59999999999996589 ) ) ;
#8497=CARTESIAN_POINT ( 'NONE',  ( -2.940415233664778860, 14.55958476633523802, -40.49999999999996447 ) ) ;
#8502=CARTESIAN_POINT ( 'NONE',  ( 4.318543150850367773, 16.81600996003516357, -39.44999999999994600 ) ) ;
#8512=CARTESIAN_POINT ( 'NONE',  ( 2.940415233664778416, 20.44041523366473712, -59.99999999999997158 ) ) ;
#8514=CARTESIAN_POINT ( 'NONE',  ( 2.439449611014226971, 12.39241881970633230, -50.40704692567388179 ) ) ;
#8515=CARTESIAN_POINT ( 'NONE',  ( 4.206979645153768210, 13.29302035484617406, -36.74999999999995737 ) ) ;
#8518=CARTESIAN_POINT ( 'NONE',  ( -2.837723661809363751, 14.45689319447982335, -29.99295307432605640 ) ) ;
#8527=CARTESIAN_POINT ( 'NONE',  ( -5.107581180293630396, 19.93944961101426827, -39.59295307432606137 ) ) ;
#8531=CARTESIAN_POINT ( 'NONE',  ( 5.852430833189966819, 16.41846101382252243, -31.95704692567387184 ) ) ;
#8535=CARTESIAN_POINT ( 'NONE',  ( -0.7417250638684240727, 11.88857024925047057, -47.69295307432606279 ) ) ;
#8553=CARTESIAN_POINT ( 'NONE',  ( -5.565992480072003978, 16.47139529956871229, -72.29295307432605000 ) ) ;
#8558=CARTESIAN_POINT ( 'NONE',  ( -0.7939530028709754772, 13.41554003082070246, -44.70704692567387184 ) ) ;
#8559=CARTESIAN_POINT ( 'NONE',  ( 0.6839900399647733664, 13.18145684914961357, -31.04999999999995808 ) ) ;
#8560=CARTESIAN_POINT ( 'NONE',  ( -3.091735541773221296, 20.59173554177323950, -65.24999999999995737 ) ) ;
#8570=CARTESIAN_POINT ( 'NONE',  ( -0.5331684895902242260, 21.84243093769531185, -28.05704692567386971 ) ) ;
#8571=CARTESIAN_POINT ( 'NONE',  ( 5.301103610786608300, 20.20104720010254340, -63.14999999999997016 ) ) ;
#8583=CARTESIAN_POINT ( 'NONE',  ( 4.103766977300021601, 21.39838383358913987, -67.50704692567386189 ) ) ;
#8587=CARTESIAN_POINT ( 'NONE',  ( -5.107581180293630396, 19.93944961101426827, -75.59295307432606137 ) ) ;
#8603=CARTESIAN_POINT ( 'NONE',  ( 0.9307174358028528216, 11.62368137996505801, -49.04999999999994742 ) ) ;
#8608=CARTESIAN_POINT ( 'NONE',  ( -4.294655364005415699, 18.33481159033935626, -69.45704692567387895 ) ) ;
#8609=CARTESIAN_POINT ( 'NONE',  ( -1.985016409143819605, 13.60418594181426855, -61.34999999999995879 ) ) ;
#8614=CARTESIAN_POINT ( 'NONE',  ( -3.091735541773221296, 20.59173554177323950, -71.24999999999994316 ) ) ;
#8618=CARTESIAN_POINT ( 'NONE',  ( 4.342430937695320736, 16.96683151040971538, -40.94295307432605568 ) ) ;
#8621=CARTESIAN_POINT ( 'NONE',  ( -0.8348115903393239501, 21.79465536400541126, -55.04295307432606421 ) ) ;
#8637=CARTESIAN_POINT ( 'NONE',  ( -5.301103610786608300, 14.79895279989743706, -58.64999999999997016 ) ) ;
#8643=DIRECTION ( 'NONE',  ( 0.7037848285661854053, -0.7037848285661920666, -0.09681854243955982653 ) ) ;
#8656=CARTESIAN_POINT ( 'NONE',  ( -2.564989113914250662, 12.12957133169093282, -41.84295307432606137 ) ) ;
#8664=CARTESIAN_POINT ( 'NONE',  ( -0.5070733663080690956, 13.37010276014318144, -62.69295307432606279 ) ) ;
#8678=CARTESIAN_POINT ( 'NONE',  ( -3.705139346311794313, 19.38786279086902198, -44.09999999999996589 ) ) ;
#8705=CARTESIAN_POINT ( 'NONE',  ( -0.6505131845895224529, 13.39282139548194195, -31.19999999999996376 ) ) ;
#8710=CARTESIAN_POINT ( 'NONE',  ( 3.705139346311793869, 15.61213720913094960, -39.59999999999996589 ) ) ;
#8719=CARTESIAN_POINT ( 'NONE',  ( 3.895814058185739448, 19.48501640914375344, -57.14999999999995595 ) ) ;
#8721=CARTESIAN_POINT ( 'NONE',  ( 2.837105286290961370, 22.73177855326409613, -49.35704692567387042 ) ) ;
#8722=CARTESIAN_POINT ( 'NONE',  ( 2.568848540478311460, 12.45835086740561692, -36.89999999999997016 ) ) ;
#8724=CARTESIAN_POINT ( 'NONE',  ( -3.199711850326840246, 20.48375923321962233, -27.74295307432605995 ) ) ;
#8736=CARTESIAN_POINT ( 'NONE',  ( -4.206979645153768210, 21.70697964515380107, -74.24999999999997158 ) ) ;
#8741=CARTESIAN_POINT ( 'NONE',  ( 2.564989113914249330, 22.87042866830903876, -40.34295307432606137 ) ) ;
#8760=CARTESIAN_POINT ( 'NONE',  ( -1.081538986177402961, 23.35243083318996327, -70.04295307432606421 ) ) ;
#8764=CARTESIAN_POINT ( 'NONE',  ( 2.940415233664778416, 20.44041523366473712, -35.99999999999996447 ) ) ;
#8766=CARTESIAN_POINT ( 'NONE',  ( 2.940415233664778416, 20.44041523366473712, -59.99999999999997158 ) ) ;
#8778=CARTESIAN_POINT ( 'NONE',  ( -4.129897239856814117, 16.99292663369196177, -24.30704692567386971 ) ) ;
#8779=CARTESIAN_POINT ( 'NONE',  ( 0.9307174358028527106, 11.62368137996505801, -67.04999999999995453 ) ) ;
#8795=CARTESIAN_POINT ( 'NONE',  ( 5.370428668309080500, 20.06498911391418360, -55.65704692567387468 ) ) ;
#8797=CARTESIAN_POINT ( 'NONE',  ( -5.900206406879871857, 18.27989588542834554, -75.44295307432606990 ) ) ;
#8815=CARTESIAN_POINT ( 'NONE',  ( -5.876318620034919782, 18.43071743580290089, -46.94999999999996021 ) ) ;
#8819=CARTESIAN_POINT ( 'NONE',  ( 0.5331684895902240040, 13.15756906230466328, -71.55704692567385905 ) ) ;
#8820=CARTESIAN_POINT ( 'NONE',  ( 1.887862790868997109, 13.79486065368817194, -60.89999999999997016 ) ) ;
#8826=CARTESIAN_POINT ( 'NONE',  ( -2.940415233664778860, 14.55958476633523802, -70.49999999999997158 ) ) ;
#8830=CARTESIAN_POINT ( 'NONE',  ( 3.895814058185739448, 19.48501640914375344, -72.14999999999996305 ) ) ;
#8832=CARTESIAN_POINT ( 'NONE',  ( -4.342430937695320736, 18.03316848959025620, -42.44295307432605568 ) ) ;
#8848=CARTESIAN_POINT ( 'NONE',  ( -5.041649132594344884, 20.06884854047834921, -62.09999999999996589 ) ) ;
#8870=CARTESIAN_POINT ( 'NONE',  ( -5.565992480072003978, 16.47139529956871229, -48.29295307432606421 ) ) ;
#8879=CARTESIAN_POINT ( 'NONE',  ( 0.5070733663080689846, 21.62989723985679902, -64.19295307432605568 ) ) ;
#8894=CARTESIAN_POINT ( 'NONE',  ( -3.895814058185739448, 15.51498359085620571, -49.64999999999995595 ) ) ;
#8896=CARTESIAN_POINT ( 'NONE',  ( -3.470745319554693342, 14.02925468044533019, -25.49999999999996803 ) ) ;
#8918=CARTESIAN_POINT ( 'NONE',  ( 4.001075405444606048, 21.50107540544455276, -74.99999999999997158 ) ) ;
#8920=CARTESIAN_POINT ( 'NONE',  ( 3.091735541773220852, 14.40826445822673563, -33.74999999999996447 ) ) ;
#8929=CARTESIAN_POINT ( 'NONE',  ( 2.940415233664778416, 20.44041523366473712, -53.99999999999996447 ) ) ;
#8931=CARTESIAN_POINT ( 'NONE',  ( 5.852430833189966819, 16.41846101382252243, -49.95704692567387184 ) ) ;
#8932=CARTESIAN_POINT ( 'NONE',  ( -5.876318620034919782, 18.43071743580290089, -31.94999999999995666 ) ) ;
#8934=CARTESIAN_POINT ( 'NONE',  ( -0.5070733663080690956, 13.37010276014318144, -29.69295307432606279 ) ) ;
#8944=CARTESIAN_POINT ( 'NONE',  ( -5.370428668309080500, 14.93501088608579153, -24.15704692567387468 ) ) ;
#8949=CARTESIAN_POINT ( 'NONE',  ( 5.900206406879871857, 16.72010411457162604, -40.94295307432605568 ) ) ;
#8969=CARTESIAN_POINT ( 'NONE',  ( 5.107581180293630396, 15.06055038898570686, -62.09295307432606847 ) ) ;
#8975=CARTESIAN_POINT ( 'NONE',  ( -4.318543150850367773, 18.18399003996480801, -31.94999999999994955 ) ) ;
#8977=CARTESIAN_POINT ( 'NONE',  ( -3.705139346311794313, 19.38786279086902198, -68.09999999999996589 ) ) ;
#8986=CARTESIAN_POINT ( 'NONE',  ( 3.639207298612508801, 15.48273827966686866, -26.10704692567387397 ) ) ;
#8987=CARTESIAN_POINT ( 'NONE',  ( -2.701047200102606460, 12.19889638921340591, -61.34999999999995879 ) ) ;
#8998=CARTESIAN_POINT ( 'NONE',  ( 2.837105286290961370, 22.73177855326409613, -52.35704692567387042 ) ) ;
#9002=CARTESIAN_POINT ( 'NONE',  ( -5.231778553264134324, 14.66289471370907727, -66.14295307432605853 ) ) ;
#9020=CARTESIAN_POINT ( 'NONE',  ( 2.701047200102605572, 22.80110361078655856, -50.84999999999997300 ) ) ;
#9025=CARTESIAN_POINT ( 'NONE',  ( 0.5331684895902240040, 13.15756906230466328, -65.55704692567385905 ) ) ;
#9026=CARTESIAN_POINT ( 'NONE',  ( -3.895814058185739892, 15.51498359085620748, -55.64999999999995595 ) ) ;
#9032=CARTESIAN_POINT ( 'NONE',  ( -1.985016409143819605, 13.60418594181426855, -70.34999999999993747 ) ) ;
#9036=CARTESIAN_POINT ( 'NONE',  ( -3.639207298612509689, 19.51726172033310647, -51.60704692567387752 ) ) ;
#9039=CARTESIAN_POINT ( 'NONE',  ( -1.887862790868997553, 21.20513934631180319, -71.39999999999996305 ) ) ;
#9043=CARTESIAN_POINT ( 'NONE',  ( 0.5070733663080689846, 21.62989723985679902, -46.19295307432605568 ) ) ;
#9058=CARTESIAN_POINT ( 'NONE',  ( 5.041649132594343996, 14.93115145952162415, -48.59999999999996589 ) ) ;
#9079=CARTESIAN_POINT ( 'NONE',  ( 5.565992480072003978, 18.52860470043125574, -40.79295307432605711 ) ) ;
#9088=CARTESIAN_POINT ( 'NONE',  ( -2.017261720333081598, 21.13920729861251857, -51.89295307432605853 ) ) ;
#9103=CARTESIAN_POINT ( 'NONE',  ( -4.318543150850367773, 18.18399003996480801, -34.94999999999996732 ) ) ;
#9128=CARTESIAN_POINT ( 'NONE',  ( -3.091735541773221296, 20.59173554177323950, -32.24999999999995737 ) ) ;
#9132=CARTESIAN_POINT ( 'NONE',  ( 1.081538986177402295, 11.64756916681001186, -35.54295307432605711 ) ) ;
#9133=CARTESIAN_POINT ( 'NONE',  ( 3.091735541773220852, 14.40826445822673563, -27.74999999999995381 ) ) ;
#9142=CARTESIAN_POINT ( 'NONE',  ( 1.985016409143818272, 21.39581405818570303, -56.84999999999995879 ) ) ;
#9145=CARTESIAN_POINT ( 'NONE',  ( -5.611429750749524992, 16.75827493613162034, -36.30704692567387326 ) ) ;
#9146=CARTESIAN_POINT ( 'NONE',  ( -5.588711115410763597, 16.61483511785016987, -25.79999999999996163 ) ) ;
#9147=CARTESIAN_POINT ( 'NONE',  ( -0.8348115903393239501, 21.79465536400541126, -28.04295307432605355 ) ) ;
#9157=CARTESIAN_POINT ( 'NONE',  ( -5.611429750749524992, 16.75827493613162034, -24.30704692567386971 ) ) ;
#9164=CARTESIAN_POINT ( 'NONE',  ( 2.698247469942395949, 12.52428291510489977, -44.39295307432605853 ) ) ;
#9180=CARTESIAN_POINT ( 'NONE',  ( -5.565992480072003978, 16.47139529956871229, -63.29295307432605000 ) ) ;
#9185=CARTESIAN_POINT ( 'NONE',  ( 0.6839900399647733664, 13.18145684914961357, -37.04999999999996163 ) ) ;
#9186=CARTESIAN_POINT ( 'NONE',  ( 4.107178604518054499, 18.15051318458946383, -51.29999999999996874 ) ) ;
#9198=CARTESIAN_POINT ( 'NONE',  ( -2.121074495332175847, 13.67351099933674341, -29.85704692567387397 ) ) ;
#9199=CARTESIAN_POINT ( 'NONE',  ( 5.301103610786608300, 20.20104720010254340, -51.14999999999996305 ) ) ;
#9213=CARTESIAN_POINT ( 'NONE',  ( 5.611429750749524992, 18.24172506386835479, -55.80704692567388037 ) ) ;
#9217=CARTESIAN_POINT ( 'NONE',  ( 4.314955953707388936, 13.40099666339979123, -71.24295307432605284 ) ) ;
#9237=CARTESIAN_POINT ( 'NONE',  ( -5.041649132594344884, 20.06884854047834921, -38.09999999999996589 ) ) ;
#9240=CARTESIAN_POINT ( 'NONE',  ( 2.983759233219601459, 14.30028814967311668, -65.25704692567387610 ) ) ;
#9241=CARTESIAN_POINT ( 'NONE',  ( -0.6505131845895224529, 13.39282139548194195, -55.19999999999997442 ) ) ;
#9248=CARTESIAN_POINT ( 'NONE',  ( 0.6505131845895220088, 21.60717860451803674, -62.69999999999996732 ) ) ;
#9250=CARTESIAN_POINT ( 'NONE',  ( -4.294655364005415699, 18.33481159033935626, -54.45704692567387895 ) ) ;
#9253=CARTESIAN_POINT ( 'NONE',  ( -4.342430937695320736, 18.03316848959025620, -27.44295307432605568 ) ) ;
#9256=CARTESIAN_POINT ( 'NONE',  ( -4.084459969179292216, 16.70604699712905372, -48.29295307432606421 ) ) ;
#9273=CARTESIAN_POINT ( 'NONE',  ( -5.041649132594344884, 20.06884854047834921, -50.09999999999996589 ) ) ;
#9289=CARTESIAN_POINT ( 'NONE',  ( 0.9307174358028528216, 11.62368137996505801, -67.04999999999994031 ) ) ;
#9294=CARTESIAN_POINT ( 'NONE',  ( 3.091735541773220852, 14.40826445822673563, -45.74999999999995737 ) ) ;
#9295=CARTESIAN_POINT ( 'NONE',  ( -5.231778553264134324, 14.66289471370907727, -42.14295307432605142 ) ) ;
#9304=CARTESIAN_POINT ( 'NONE',  ( 4.342430937695320736, 16.96683151040971538, -55.94295307432605568 ) ) ;
#9319=CARTESIAN_POINT ( 'NONE',  ( -0.6839900399647736995, 21.81854315085035623, -38.54999999999996874 ) ) ;
#9345=CARTESIAN_POINT ( 'NONE',  ( -2.121074495332175847, 13.67351099933674341, -38.85704692567387752 ) ) ;
#9348=CARTESIAN_POINT ( 'NONE',  ( 5.900206406879871857, 16.72010411457162604, -31.94295307432605568 ) ) ;
#9349=CARTESIAN_POINT ( 'NONE',  ( -2.983759233219601903, 20.69971185032686023, -72.75704692567386189 ) ) ;
#9357=CARTESIAN_POINT ( 'NONE',  ( -0.6505131845895224529, 13.39282139548194195, -49.19999999999996732 ) ) ;
#9360=CARTESIAN_POINT ( 'NONE',  ( -5.852430833189966819, 18.58153898617744915, -33.45704692567387895 ) ) ;
#9362=CARTESIAN_POINT ( 'NONE',  ( -0.6505131845895224529, 13.39282139548194195, -64.19999999999996021 ) ) ;
#9373=CARTESIAN_POINT ( 'NONE',  ( -4.103766977300021601, 13.60161616641083704, -24.00704692567387610 ) ) ;
#9377=CARTESIAN_POINT ( 'NONE',  ( 0.7417250638684235176, 23.11142975074950101, -46.19295307432605568 ) ) ;
#9395=CARTESIAN_POINT ( 'NONE',  ( -5.231778553264134324, 14.66289471370907727, -66.14295307432605853 ) ) ;
#9400=CARTESIAN_POINT ( 'NONE',  ( -3.091735541773221296, 20.59173554177323950, -29.24999999999996447 ) ) ;
#9401=CARTESIAN_POINT ( 'NONE',  ( 3.895814058185739448, 19.48501640914375344, -51.14999999999994884 ) ) ;
#9412=CARTESIAN_POINT ( 'NONE',  ( -2.837105286290963146, 12.26822144673588255, -68.85704692567387042 ) ) ;
#9413=CARTESIAN_POINT ( 'NONE',  ( 5.041649132594343996, 14.93115145952162415, -51.59999999999996589 ) ) ;
#9424=CARTESIAN_POINT ( 'NONE',  ( -4.099003336600151925, 21.81495595370741469, -57.75704692567386900 ) ) ;
#9427=CARTESIAN_POINT ( 'NONE',  ( -0.7417250638684240727, 11.88857024925047057, -74.69295307432606990 ) ) ;
#9442=CARTESIAN_POINT ( 'NONE',  ( -4.206979645153768210, 21.70697964515380107, -41.24999999999995026 ) ) ;
#9446=CARTESIAN_POINT ( 'NONE',  ( -4.294655364005415699, 18.33481159033935626, -60.45704692567387895 ) ) ;
#9448=CARTESIAN_POINT ( 'NONE',  ( 3.705139346311793869, 15.61213720913094960, -48.59999999999996589 ) ) ;
#9453=AXIS2_PLACEMENT_3D ( 'NONE', #36540, #31922, #26554 ) ;
#9458=CARTESIAN_POINT ( 'NONE',  ( -2.940415233664778860, 14.55958476633523802, -67.49999999999995737 ) ) ;
#9460=CARTESIAN_POINT ( 'NONE',  ( 4.294655364005415699, 16.66518840966061887, -40.95704692567387184 ) ) ;
#9463=CARTESIAN_POINT ( 'NONE',  ( -3.771071394011080269, 19.25846386140493394, -27.59295307432605782 ) ) ;
#9466=CARTESIAN_POINT ( 'NONE',  ( 3.826489000663266360, 19.62107449533211678, -49.64295307432606563 ) ) ;
#9482=CARTESIAN_POINT ( 'NONE',  ( -5.588711115410763597, 16.61483511785016987, -52.79999999999996874 ) ) ;
#9498=CARTESIAN_POINT ( 'NONE',  ( -5.041649132594344884, 20.06884854047834921, -71.09999999999996589 ) ) ;
#9503=CARTESIAN_POINT ( 'NONE',  ( -1.985016409143819605, 13.60418594181426855, -43.34999999999994458 ) ) ;
#9514=CARTESIAN_POINT ( 'NONE',  ( 2.837723661809363307, 20.54310680552015356, -52.49295307432605995 ) ) ;
#9532=CARTESIAN_POINT ( 'NONE',  ( -4.318543150850367773, 18.18399003996480801, -37.94999999999996021 ) ) ;
#9559=CARTESIAN_POINT ( 'NONE',  ( -3.043106805520194413, 14.66227633819065623, -36.00704692567386189 ) ) ;
#9564=CARTESIAN_POINT ( 'NONE',  ( 2.698247469942395949, 12.52428291510489977, -38.39295307432605142 ) ) ;
#9565=CARTESIAN_POINT ( 'NONE',  ( -1.887862790868997553, 21.20513934631180319, -26.39999999999996660 ) ) ;
#9573=CARTESIAN_POINT ( 'NONE',  ( 1.985016409143818272, 21.39581405818570303, -47.84999999999994458 ) ) ;
#9576=CARTESIAN_POINT ( 'NONE',  ( -5.852430833189966819, 18.58153898617744915, -36.45704692567386473 ) ) ;
#9577=CARTESIAN_POINT ( 'NONE',  ( -4.001075405444606936, 13.49892459455542060, -25.49999999999996803 ) ) ;
#9578=CARTESIAN_POINT ( 'NONE',  ( 0.6505131845895220088, 21.60717860451803674, -62.69999999999996732 ) ) ;
#9593=CARTESIAN_POINT ( 'NONE',  ( 3.898383833589191383, 21.60376697729997275, -46.49295307432606705 ) ) ;
#9609=CARTESIAN_POINT ( 'NONE',  ( 5.900206406879871857, 16.72010411457162604, -67.94295307432605568 ) ) ;
#9614=CARTESIAN_POINT ( 'NONE',  ( -1.887862790868997553, 21.20513934631180319, -26.39999999999996660 ) ) ;
#9615=CARTESIAN_POINT ( 'NONE',  ( 3.705139346311793869, 15.61213720913094960, -57.59999999999997300 ) ) ;
#9627=CARTESIAN_POINT ( 'NONE',  ( 5.370428668309080500, 20.06498911391418360, -67.65704692567386758 ) ) ;
#9628=CARTESIAN_POINT ( 'NONE',  ( 0.8851648821498760977, 23.08871111541074228, -59.69999999999996732 ) ) ;
#9639=CARTESIAN_POINT ( 'NONE',  ( -1.028604700431329233, 11.93400751992799513, -50.70704692567387184 ) ) ;
#9644=CARTESIAN_POINT ( 'NONE',  ( -1.081538986177402961, 23.35243083318996327, -70.04295307432606421 ) ) ;
#9662=CARTESIAN_POINT ( 'NONE',  ( 0.8851648821498760977, 23.08871111541074228, -41.69999999999996732 ) ) ;
#9666=CARTESIAN_POINT ( 'NONE',  ( -0.5331684895902242260, 21.84243093769531185, -58.05704692567386616 ) ) ;
#9668=CARTESIAN_POINT ( 'NONE',  ( 0.6839900399647732554, 13.18145684914961357, -52.04999999999996874 ) ) ;
#9677=CARTESIAN_POINT ( 'NONE',  ( -0.6505131845895224529, 13.39282139548194195, -61.19999999999996732 ) ) ;
#9680=CARTESIAN_POINT ( 'NONE',  ( -3.043106805520194413, 14.66227633819065623, -45.00704692567388321 ) ) ;
#9685=CARTESIAN_POINT ( 'NONE',  ( 2.017261720333081598, 13.86079270138745834, -47.39295307432605853 ) ) ;
#9700=PRODUCT_CONTEXT ( 'NONE', #8151, 'mechanical' ) ;
#9701=CARTESIAN_POINT ( 'NONE',  ( -2.701047200102606016, 12.19889638921340413, -52.34999999999994458 ) ) ;
#9715=CARTESIAN_POINT ( 'NONE',  ( 0.9307174358028528216, 11.62368137996505801, -70.04999999999996874 ) ) ;
#9721=CARTESIAN_POINT ( 'NONE',  ( -3.705139346311794313, 19.38786279086902198, -41.09999999999996589 ) ) ;
#9734=CARTESIAN_POINT ( 'NONE',  ( -3.826489000663265472, 15.37892550466785480, -60.14295307432605142 ) ) ;
#9749=CARTESIAN_POINT ( 'NONE',  ( 1.887862790868997109, 13.79486065368817194, -39.89999999999996305 ) ) ;
#9778=CARTESIAN_POINT ( 'NONE',  ( 0.7939530028709752552, 21.58445996917927445, -31.20704692567387539 ) ) ;
#9782=CARTESIAN_POINT ( 'NONE',  ( 4.314955953707388936, 13.40099666339979123, -35.24295307432605995 ) ) ;
#9783=CARTESIAN_POINT ( 'NONE',  ( -0.6505131845895224529, 13.39282139548194195, -28.19999999999996732 ) ) ;
#9791=CARTESIAN_POINT ( 'NONE',  ( 1.887862790868997109, 13.79486065368817194, -42.89999999999996305 ) ) ;
#9794=CARTESIAN_POINT ( 'NONE',  ( -0.7798958854283041253, 23.40020640687986386, -40.05704692567387326 ) ) ;
#9796=CARTESIAN_POINT ( 'NONE',  ( 1.985016409143818272, 21.39581405818570303, -68.84999999999996589 ) ) ;
#9809=CARTESIAN_POINT ( 'NONE',  ( -1.081538986177402961, 23.35243083318996327, -28.04295307432605355 ) ) ;
#9831=CARTESIAN_POINT ( 'NONE',  ( -4.318543150850367773, 18.18399003996480801, -49.94999999999994600 ) ) ;
#9841=CARTESIAN_POINT ( 'NONE',  ( 4.103766977300021601, 21.39838383358913987, -64.50704692567389031 ) ) ;
#9842=CARTESIAN_POINT ( 'NONE',  ( -2.568848540478311904, 22.54164913259435465, -59.39999999999997016 ) ) ;
#9858=CARTESIAN_POINT ( 'NONE',  ( 5.370428668309080500, 20.06498911391418360, -49.65704692567388179 ) ) ;
#9862=CARTESIAN_POINT ( 'NONE',  ( 5.900206406879871857, 16.72010411457162604, -73.94295307432606990 ) ) ;
#9879=CARTESIAN_POINT ( 'NONE',  ( -0.9307174358028533767, 23.37631862003491889, -38.54999999999996874 ) ) ;
#9882=CARTESIAN_POINT ( 'NONE',  ( -3.043106805520194413, 14.66227633819065623, -60.00704692567389031 ) ) ;
#9883=CARTESIAN_POINT ( 'NONE',  ( -1.887862790868997553, 21.20513934631180319, -50.39999999999996305 ) ) ;
#9891=CARTESIAN_POINT ( 'NONE',  ( 1.985016409143818272, 21.39581405818570303, -65.84999999999992326 ) ) ;
#9893=CARTESIAN_POINT ( 'NONE',  ( 3.043106805520193525, 20.33772366180932067, -43.50704692567387610 ) ) ;
#9897=CARTESIAN_POINT ( 'NONE',  ( -3.771071394011080269, 19.25846386140493394, -33.59295307432606137 ) ) ;
#9912=CARTESIAN_POINT ( 'NONE',  ( 4.206979645153767322, 13.29302035484617051, -51.74999999999994316 ) ) ;
#9928=CARTESIAN_POINT ( 'NONE',  ( -5.852430833189966819, 18.58153898617744915, -24.45704692567386829 ) ) ;
#9933=CARTESIAN_POINT ( 'NONE',  ( 3.705139346311793869, 15.61213720913094960, -39.59999999999996589 ) ) ;
#9945=CARTESIAN_POINT ( 'NONE',  ( 2.017261720333081598, 13.86079270138745834, -59.39295307432605853 ) ) ;
#9960=CARTESIAN_POINT ( 'NONE',  ( -0.6505131845895224529, 13.39282139548194195, -40.19999999999996732 ) ) ;
#9980=CARTESIAN_POINT ( 'NONE',  ( 4.294655364005415699, 16.66518840966061887, -34.95704692567387895 ) ) ;
#9984=CARTESIAN_POINT ( 'NONE',  ( 5.565992480072003978, 18.52860470043125574, -37.79295307432605711 ) ) ;
#9985=CARTESIAN_POINT ( 'NONE',  ( -1.758463861404912842, 21.27107139401109137, -69.90704692567388179 ) ) ;
#9992=CARTESIAN_POINT ( 'NONE',  ( 3.705139346311793869, 15.61213720913094960, -48.59999999999996589 ) ) ;
#9995=CARTESIAN_POINT ( 'NONE',  ( 5.852430833189966819, 16.41846101382252243, -37.95704692567387184 ) ) ;
#9996=CARTESIAN_POINT ( 'NONE',  ( 0.8851648821498760977, 23.08871111541074228, -29.69999999999996376 ) ) ;
#9997=CARTESIAN_POINT ( 'NONE',  ( -1.985016409143819605, 13.60418594181426855, -61.34999999999996589 ) ) ;
#10011=CARTESIAN_POINT ( 'NONE',  ( -4.314955953707389824, 21.59900333660018390, -30.74295307432605640 ) ) ;
#10031=CARTESIAN_POINT ( 'NONE',  ( 4.318543150850367773, 16.81600996003516357, -51.44999999999997442 ) ) ;
#10039=CARTESIAN_POINT ( 'NONE',  ( -5.370428668309080500, 14.93501088608579153, -63.15704692567388179 ) ) ;
#10040=CARTESIAN_POINT ( 'NONE',  ( 2.701047200102605128, 22.80110361078656211, -56.84999999999996589 ) ) ;
#10053=CARTESIAN_POINT ( 'NONE',  ( 4.975717084895059372, 14.80175253005754143, -47.10704692567387042 ) ) ;
#10060=CARTESIAN_POINT ( 'NONE',  ( -5.900206406879871857, 18.27989588542834554, -63.44295307432605568 ) ) ;
#10071=CARTESIAN_POINT ( 'NONE',  ( -5.301103610786608300, 14.79895279989743706, -43.64999999999996305 ) ) ;
#10074=CARTESIAN_POINT ( 'NONE',  ( -2.121074495332175847, 13.67351099933674341, -50.85704692567387752 ) ) ;
#10075=CARTESIAN_POINT ( 'NONE',  ( -1.985016409143819605, 13.60418594181426855, -49.34999999999996589 ) ) ;
#10087=CARTESIAN_POINT ( 'NONE',  ( 3.091735541773220852, 14.40826445822673563, -63.74999999999997868 ) ) ;
#10090=CARTESIAN_POINT ( 'NONE',  ( -2.121074495332175847, 13.67351099933674341, -41.85704692567387752 ) ) ;
#10094=CARTESIAN_POINT ( 'NONE',  ( 3.771071394011080269, 15.74153613859503764, -38.09295307432605426 ) ) ;
#10101=CARTESIAN_POINT ( 'NONE',  ( -3.639207298612509689, 19.51726172033310647, -24.60704692567387397 ) ) ;
#10108=CARTESIAN_POINT ( 'NONE',  ( 5.876318620034919782, 16.56928256419707068, -36.44999999999996732 ) ) ;
#10123=CARTESIAN_POINT ( 'NONE',  ( 5.588711115410763597, 18.38516488214980882, -72.29999999999996874 ) ) ;
#10128=CARTESIAN_POINT ( 'NONE',  ( 2.940415233664778416, 20.44041523366473712, -44.99999999999997158 ) ) ;
#10139=CARTESIAN_POINT ( 'NONE',  ( -0.5070733663080690956, 13.37010276014318144, -50.69295307432606279 ) ) ;
#10145=CARTESIAN_POINT ( 'NONE',  ( -4.342430937695320736, 18.03316848959025620, -66.44295307432605568 ) ) ;
#10156=CARTESIAN_POINT ( 'NONE',  ( -2.940415233664778860, 14.55958476633523802, -25.49999999999996803 ) ) ;
#10163=CARTESIAN_POINT ( 'NONE',  ( -0.7798958854283041253, 23.40020640687986386, -25.05704692567386971 ) ) ;
#10183=CARTESIAN_POINT ( 'NONE',  ( 1.758463861404912620, 13.72892860598888731, -29.40704692567386758 ) ) ;
#10186=CARTESIAN_POINT ( 'NONE',  ( -3.771071394011080269, 19.25846386140493394, -75.59295307432606137 ) ) ;
#10187=CARTESIAN_POINT ( 'NONE',  ( 3.043106805520193525, 20.33772366180932067, -64.50704692567389031 ) ) ;
#10195=CARTESIAN_POINT ( 'NONE',  ( 0.6505131845895220088, 21.60717860451803674, -41.69999999999996732 ) ) ;
#10199=CARTESIAN_POINT ( 'NONE',  ( 5.611429750749524992, 18.24172506386835479, -28.80704692567387326 ) ) ;
#10201=CARTESIAN_POINT ( 'NONE',  ( 4.107178604518054499, 18.15051318458946383, -60.29999999999996163 ) ) ;
#10214=CARTESIAN_POINT ( 'NONE',  ( -2.698247469942396837, 22.47571708489507358, -36.89295307432605142 ) ) ;
#10231=CARTESIAN_POINT ( 'NONE',  ( -2.940415233664778860, 14.55958476633523802, -40.49999999999996447 ) ) ;
#10240=CARTESIAN_POINT ( 'NONE',  ( 4.342430937695320736, 16.96683151040971538, -28.94295307432605568 ) ) ;
#10242=CARTESIAN_POINT ( 'NONE',  ( -4.099003336600151925, 21.81495595370741469, -63.75704692567388321 ) ) ;
#10243=CARTESIAN_POINT ( 'NONE',  ( 2.568848540478311460, 12.45835086740561692, -45.89999999999997016 ) ) ;
#10258=CARTESIAN_POINT ( 'NONE',  ( 1.028604700431328567, 23.06599248007198355, -43.20704692567387184 ) ) ;
#10264=CARTESIAN_POINT ( 'NONE',  ( 3.898383833589191383, 21.60376697729997275, -61.49295307432606705 ) ) ;
#10277=CARTESIAN_POINT ( 'NONE',  ( -2.701047200102606016, 12.19889638921340413, -31.34999999999996945 ) ) ;
#10280=CARTESIAN_POINT ( 'NONE',  ( -4.294655364005415699, 18.33481159033935626, -51.45704692567387895 ) ) ;
#10281=CARTESIAN_POINT ( 'NONE',  ( -4.107178604518053611, 16.84948681541050775, -43.79999999999996163 ) ) ;
#10283=CARTESIAN_POINT ( 'NONE',  ( 3.895814058185739448, 19.48501640914375344, -69.14999999999994884 ) ) ;
#10292=CARTESIAN_POINT ( 'NONE',  ( -4.318543150850367773, 18.18399003996480801, -55.94999999999997442 ) ) ;
#10294=CARTESIAN_POINT ( 'NONE',  ( 4.129897239856814117, 18.00707336630801336, -43.80704692567387326 ) ) ;
#10298=CARTESIAN_POINT ( 'NONE',  ( -3.199711850326840246, 20.48375923321962233, -36.74295307432605995 ) ) ;
#10305=CARTESIAN_POINT ( 'NONE',  ( -2.121074495332175847, 13.67351099933674341, -26.85704692567387397 ) ) ;
#10311=SHAPE_DEFINITION_REPRESENTATION ( #5470, #1913 ) ;
#10312=CARTESIAN_POINT ( 'NONE',  ( 2.568848540478311460, 12.45835086740561692, -39.89999999999996305 ) ) ;
#10333=CARTESIAN_POINT ( 'NONE',  ( 5.876318620034919782, 16.56928256419707068, -57.44999999999996732 ) ) ;
#10338=CARTESIAN_POINT ( 'NONE',  ( 3.091735541773220852, 14.40826445822673563, -36.74999999999994316 ) ) ;
#10339=CARTESIAN_POINT ( 'NONE',  ( 0.6839900399647732554, 13.18145684914961357, -73.04999999999998295 ) ) ;
#10351=CARTESIAN_POINT ( 'NONE',  ( 0.8348115903393232839, 13.20534463599456387, -50.54295307432606421 ) ) ;
#10356=CARTESIAN_POINT ( 'NONE',  ( 3.771071394011080269, 15.74153613859503764, -65.09295307432604716 ) ) ;
#10367=CARTESIAN_POINT ( 'NONE',  ( -3.091735541773221296, 20.59173554177323950, -29.24999999999996447 ) ) ;
#10375=CARTESIAN_POINT ( 'NONE',  ( 0.8851648821498760977, 23.08871111541074228, -62.69999999999996732 ) ) ;
#10394=CARTESIAN_POINT ( 'NONE',  ( 4.314955953707388936, 13.40099666339979123, -68.24295307432605284 ) ) ;
#10398=CARTESIAN_POINT ( 'NONE',  ( 2.983759233219601459, 14.30028814967311668, -29.25704692567387255 ) ) ;
#10402=CARTESIAN_POINT ( 'NONE',  ( 3.199711850326839357, 14.51624076678035635, -74.24295307432606705 ) ) ;
#10403=CARTESIAN_POINT ( 'NONE',  ( -3.965139115708213868, 15.65104167704456906, -63.15704692567388179 ) ) ;
#10412=CARTESIAN_POINT ( 'NONE',  ( 3.091735541773220852, 14.40826445822673563, -39.74999999999996447 ) ) ;
#10416=CARTESIAN_POINT ( 'NONE',  ( 4.103766977300021601, 21.39838383358913987, -28.50704692567387610 ) ) ;
#10417=CARTESIAN_POINT ( 'NONE',  ( -1.985016409143819605, 13.60418594181426855, -58.34999999999995879 ) ) ;
#10428=CARTESIAN_POINT ( 'NONE',  ( 5.107581180293630396, 15.06055038898570686, -35.09295307432605426 ) ) ;
#10448=CARTESIAN_POINT ( 'NONE',  ( -3.705139346311794313, 19.38786279086902198, -47.09999999999996589 ) ) ;
#10456=CARTESIAN_POINT ( 'NONE',  ( -4.107178604518053611, 16.84948681541050775, -64.79999999999996874 ) ) ;
#10458=CARTESIAN_POINT ( 'NONE',  ( 4.975717084895059372, 14.80175253005754143, -59.10704692567387752 ) ) ;
#10459=CARTESIAN_POINT ( 'NONE',  ( 5.301103610786608300, 20.20104720010254340, -42.14999999999996305 ) ) ;
#10472=CARTESIAN_POINT ( 'NONE',  ( -1.028604700431329233, 11.93400751992799513, -47.70704692567387184 ) ) ;
#10476=CARTESIAN_POINT ( 'NONE',  ( -4.314955953707389824, 21.59900333660018390, -63.74295307432605995 ) ) ;
#10489=CARTESIAN_POINT ( 'NONE',  ( 5.876318620034919782, 16.56928256419707068, -36.44999999999996732 ) ) ;
#10492=CARTESIAN_POINT ( 'NONE',  ( -4.129897239856814117, 16.99292663369196177, -54.30704692567388037 ) ) ;
#10493=CARTESIAN_POINT ( 'NONE',  ( -3.895814058185739892, 15.51498359085620748, -40.64999999999995595 ) ) ;
#10495=CARTESIAN_POINT ( 'NONE',  ( 4.107178604518054499, 18.15051318458946383, -72.29999999999996874 ) ) ;
#10506=CARTESIAN_POINT ( 'NONE',  ( -3.091735541773221296, 20.59173554177323950, -50.24999999999997158 ) ) ;
#10508=CARTESIAN_POINT ( 'NONE',  ( 2.121074495332174958, 21.32648900066323350, -31.35704692567387042 ) ) ;
#10509=CARTESIAN_POINT ( 'NONE',  ( 2.701047200102605128, 22.80110361078656211, -71.84999999999996589 ) ) ;
#10512=CARTESIAN_POINT ( 'NONE',  ( 2.837723661809363307, 20.54310680552015356, -40.49295307432605995 ) ) ;
#10519=CARTESIAN_POINT ( 'NONE',  ( 4.129897239856814117, 18.00707336630801336, -25.80704692567386971 ) ) ;
#10525=CARTESIAN_POINT ( 'NONE',  ( -0.9307174358028533767, 23.37631862003491889, -35.54999999999994742 ) ) ;
#10545=CARTESIAN_POINT ( 'NONE',  ( -4.206979645153768210, 21.70697964515380107, -62.24999999999995737 ) ) ;
#10550=CARTESIAN_POINT ( 'NONE',  ( 0.6839900399647733664, 13.18145684914961357, -37.04999999999996163 ) ) ;
#10551=CARTESIAN_POINT ( 'NONE',  ( 3.705139346311793869, 15.61213720913094960, -63.59999999999995879 ) ) ;
#10553=UNCERTAINTY_MEASURE_WITH_UNIT (LENGTH_MEASURE( 1.000000000000000082E-05 ), #31515, 'distance_accuracy_value', 'NONE');
#10565=CARTESIAN_POINT ( 'NONE',  ( 2.017261720333081598, 13.86079270138745834, -50.39295307432605853 ) ) ;
#10570=CARTESIAN_POINT ( 'NONE',  ( 2.837723661809363307, 20.54310680552015356, -64.49295307432606705 ) ) ;
#10582=CARTESIAN_POINT ( 'NONE',  ( -1.985016409143819605, 13.60418594181426855, -31.34999999999996945 ) ) ;
#10590=CARTESIAN_POINT ( 'NONE',  ( 5.588711115410763597, 18.38516488214980882, -66.29999999999996874 ) ) ;
#10615=CARTESIAN_POINT ( 'NONE',  ( 0.5070733663080689846, 21.62989723985679902, -73.19295307432605568 ) ) ;
#10616=CARTESIAN_POINT ( 'NONE',  ( 0.7939530028709752552, 21.58445996917927445, -64.20704692567387895 ) ) ;
#10629=CARTESIAN_POINT ( 'NONE',  ( -5.370428668309080500, 14.93501088608579153, -30.15704692567386758 ) ) ;
#10631=CARTESIAN_POINT ( 'NONE',  ( -4.318543150850367773, 18.18399003996480801, -52.94999999999994600 ) ) ;
#10644=CARTESIAN_POINT ( 'NONE',  ( -5.900206406879871857, 18.27989588542834554, -36.44295307432606279 ) ) ;
#10661=CARTESIAN_POINT ( 'NONE',  ( -0.6839900399647736995, 21.81854315085035623, -41.54999999999996874 ) ) ;
#10670=CARTESIAN_POINT ( 'NONE',  ( 3.895814058185739448, 19.48501640914375344, -66.14999999999997726 ) ) ;
#10672=CARTESIAN_POINT ( 'NONE',  ( 2.439449611014226971, 12.39241881970633230, -56.40704692567388179 ) ) ;
#10673=CARTESIAN_POINT ( 'NONE',  ( -0.8851648821498765418, 11.91128888458923285, -46.19999999999996021 ) ) ;
#10685=CARTESIAN_POINT ( 'NONE',  ( -4.103766977300021601, 13.60161616641083704, -48.00704692567387610 ) ) ;
#10689=CARTESIAN_POINT ( 'NONE',  ( 4.314955953707388936, 13.40099666339979123, -59.24295307432605995 ) ) ;
#10703=CARTESIAN_POINT ( 'NONE',  ( 4.001075405444606048, 21.50107540544455276, -29.99999999999996447 ) ) ;
#10706=CARTESIAN_POINT ( 'NONE',  ( -3.043106805520194413, 14.66227633819065623, -54.00704692567387610 ) ) ;
#10707=CARTESIAN_POINT ( 'NONE',  ( -4.318543150850367773, 18.18399003996480801, -70.94999999999997442 ) ) ;
#10712=CARTESIAN_POINT ( 'NONE',  ( 1.887862790868997109, 13.79486065368817194, -54.89999999999996305 ) ) ;
#10714=CARTESIAN_POINT ( 'NONE',  ( 3.043106805520193525, 20.33772366180932067, -31.50704692567387610 ) ) ;
#10715=CARTESIAN_POINT ( 'NONE',  ( 2.568848540478311460, 12.45835086740561692, -72.89999999999996305 ) ) ;
#10719=CARTESIAN_POINT ( 'NONE',  ( 2.837723661809363307, 20.54310680552015356, -34.49295307432605995 ) ) ;
#10725=CARTESIAN_POINT ( 'NONE',  ( 2.837105286290961370, 22.73177855326409613, -73.35704692567385621 ) ) ;
#10732=CARTESIAN_POINT ( 'NONE',  ( 0.9307174358028528216, 11.62368137996505801, -37.04999999999996163 ) ) ;
#10748=CARTESIAN_POINT ( 'NONE',  ( -0.8851648821498765418, 11.91128888458923285, -58.19999999999996732 ) ) ;
#10753=CARTESIAN_POINT ( 'NONE',  ( -1.887862790868997553, 21.20513934631180319, -38.39999999999997016 ) ) ;
#10754=CARTESIAN_POINT ( 'NONE',  ( -2.940415233664778860, 14.55958476633523802, -70.49999999999997158 ) ) ;
#10766=CARTESIAN_POINT ( 'NONE',  ( -3.771071394011080269, 19.25846386140493394, -45.59295307432606137 ) ) ;
#10771=CARTESIAN_POINT ( 'NONE',  ( 4.342430937695320736, 16.96683151040971538, -67.94295307432605568 ) ) ;
#10781=CARTESIAN_POINT ( 'NONE',  ( 0.6839900399647733664, 13.18145684914961357, -31.04999999999995808 ) ) ;
#10790=CARTESIAN_POINT ( 'NONE',  ( -5.301103610786608300, 14.79895279989743706, -67.64999999999997726 ) ) ;
#10809=CARTESIAN_POINT ( 'NONE',  ( -5.231778553264134324, 14.66289471370907727, -54.14295307432606563 ) ) ;
#10818=CARTESIAN_POINT ( 'NONE',  ( -0.5070733663080690956, 13.37010276014318144, -71.69295307432605568 ) ) ;
#10821=CARTESIAN_POINT ( 'NONE',  ( -3.043106805520194413, 14.66227633819065623, -66.00704692567386189 ) ) ;
#10834=CARTESIAN_POINT ( 'NONE',  ( -2.439449611014227859, 22.60758118029364283, -24.90704692567387823 ) ) ;
#10836=CARTESIAN_POINT ( 'NONE',  ( 3.091735541773220852, 14.40826445822673563, -51.74999999999994316 ) ) ;
#10848=CARTESIAN_POINT ( 'NONE',  ( -3.826489000663265472, 15.37892550466785480, -75.14295307432605853 ) ) ;
#10869=CARTESIAN_POINT ( 'NONE',  ( -3.895814058185739448, 15.51498359085620571, -46.64999999999994884 ) ) ;
#10881=CARTESIAN_POINT ( 'NONE',  ( -2.940415233664778860, 14.55958476633523802, -64.49999999999997158 ) ) ;
#10883=CARTESIAN_POINT ( 'NONE',  ( 5.852430833189966819, 16.41846101382252243, -52.95704692567387895 ) ) ;
#10884=CARTESIAN_POINT ( 'NONE',  ( -4.001075405444606936, 13.49892459455542060, -43.49999999999997158 ) ) ;
#10898=CARTESIAN_POINT ( 'NONE',  ( 4.099003336600150149, 13.18504404629255689, -35.25704692567386900 ) ) ;
#10901=CARTESIAN_POINT ( 'NONE',  ( -0.7417250638684240727, 11.88857024925047057, -56.69295307432606279 ) ) ;
#10917=CARTESIAN_POINT ( 'NONE',  ( -5.041649132594344884, 20.06884854047834921, -35.09999999999996589 ) ) ;
#10921=CARTESIAN_POINT ( 'NONE',  ( 1.758463861404912620, 13.72892860598888731, -50.40704692567388179 ) ) ;
#10928=CARTESIAN_POINT ( 'NONE',  ( -1.887862790868997553, 21.20513934631180319, -59.39999999999997016 ) ) ;
#10930=CARTESIAN_POINT ( 'NONE',  ( 2.121074495332174958, 21.32648900066323350, -37.35704692567387752 ) ) ;
#10941=CARTESIAN_POINT ( 'NONE',  ( -5.611429750749524992, 16.75827493613162034, -69.30704692567387326 ) ) ;
#10946=CARTESIAN_POINT ( 'NONE',  ( -5.588711115410763597, 16.61483511785016987, -40.79999999999996874 ) ) ;
#10963=CARTESIAN_POINT ( 'NONE',  ( 5.041649132594343996, 14.93115145952162415, -63.59999999999995879 ) ) ;
#10969=CARTESIAN_POINT ( 'NONE',  ( 3.705139346311793869, 15.61213720913094960, -33.59999999999996589 ) ) ;
#10970=CARTESIAN_POINT ( 'NONE',  ( -2.940415233664778860, 14.55958476633523802, -67.49999999999995737 ) ) ;
#10981=CARTESIAN_POINT ( 'NONE',  ( 0.8348115903393232839, 13.20534463599456387, -47.54295307432606421 ) ) ;
#10986=CARTESIAN_POINT ( 'NONE',  ( -0.5070733663080690956, 13.37010276014318144, -56.69295307432606279 ) ) ;
#10996=CARTESIAN_POINT ( 'NONE',  ( -0.6505131845895224529, 13.39282139548194195, -28.19999999999996732 ) ) ;
#11004=CARTESIAN_POINT ( 'NONE',  ( 5.876318620034919782, 16.56928256419707068, -69.44999999999997442 ) ) ;
#11026=CARTESIAN_POINT ( 'NONE',  ( -2.698247469942396837, 22.47571708489507358, -57.89295307432605853 ) ) ;
#11034=CARTESIAN_POINT ( 'NONE',  ( -0.8348115903393239501, 21.79465536400541126, -76.04295307432605000 ) ) ;
#11037=CARTESIAN_POINT ( 'NONE',  ( -2.121074495332175847, 13.67351099933674341, -50.85704692567387752 ) ) ;
#11051=CARTESIAN_POINT ( 'NONE',  ( 4.107178604518054499, 18.15051318458946383, -54.29999999999996874 ) ) ;
#11064=CARTESIAN_POINT ( 'NONE',  ( -3.771071394011080269, 19.25846386140493394, -72.59295307432606137 ) ) ;
#11082=DIRECTION ( 'NONE',  ( -0.7037848285661852943, 0.7037848285661921777, -0.09681854243955982653 ) ) ;
#11084=CARTESIAN_POINT ( 'NONE',  ( -3.705139346311794313, 19.38786279086902198, -44.09999999999996589 ) ) ;
#11093=CARTESIAN_POINT ( 'NONE',  ( 1.985016409143818272, 21.39581405818570303, -65.84999999999992326 ) ) ;
#11095=CARTESIAN_POINT ( 'NONE',  ( 0.7798958854283032371, 11.59979359312010772, -59.55704692567387326 ) ) ;
#11096=CARTESIAN_POINT ( 'NONE',  ( -2.701047200102606460, 12.19889638921340591, -43.34999999999995879 ) ) ;
#11110=CARTESIAN_POINT ( 'NONE',  ( -4.103766977300021601, 13.60161616641083704, -39.00704692567386900 ) ) ;
#11113=CARTESIAN_POINT ( 'NONE',  ( 4.314955953707388936, 13.40099666339979123, -53.24295307432605995 ) ) ;
#11131=CARTESIAN_POINT ( 'NONE',  ( 0.000000000000000000, 0.000000000000000000, 0.000000000000000000 ) ) ;
#11132=CARTESIAN_POINT ( 'NONE',  ( 0.8851648821498760977, 23.08871111541074228, -32.69999999999996732 ) ) ;
#11135=CARTESIAN_POINT ( 'NONE',  ( -1.758463861404912842, 21.27107139401109137, -45.90704692567387468 ) ) ;
#11136=CARTESIAN_POINT ( 'NONE',  ( 4.318543150850367773, 16.81600996003516357, -69.44999999999997442 ) ) ;
#11143=CARTESIAN_POINT ( 'NONE',  ( -2.940415233664778860, 14.55958476633523802, -55.49999999999996447 ) ) ;
#11146=CARTESIAN_POINT ( 'NONE',  ( 1.758463861404912620, 13.72892860598888731, -35.40704692567386758 ) ) ;
#11147=CARTESIAN_POINT ( 'NONE',  ( 5.588711115410763597, 18.38516488214980882, -72.29999999999996874 ) ) ;
#11158=CARTESIAN_POINT ( 'NONE',  ( 4.103766977300021601, 21.39838383358913987, -64.50704692567389031 ) ) ;
#11162=CARTESIAN_POINT ( 'NONE',  ( 5.876318620034919782, 16.56928256419707068, -30.44999999999995310 ) ) ;
#11179=CARTESIAN_POINT ( 'NONE',  ( 5.876318620034919782, 16.56928256419707068, -60.44999999999997442 ) ) ;
#11183=CARTESIAN_POINT ( 'NONE',  ( 0.5331684895902240040, 13.15756906230466328, -68.55704692567387326 ) ) ;
#11184=CARTESIAN_POINT ( 'NONE',  ( 1.887862790868997109, 13.79486065368817194, -69.89999999999996305 ) ) ;
#11194=CARTESIAN_POINT ( 'NONE',  ( 3.826489000663266360, 19.62107449533211678, -34.64295307432605142 ) ) ;
#11199=CARTESIAN_POINT ( 'NONE',  ( 4.342430937695320736, 16.96683151040971538, -55.94295307432605568 ) ) ;
#11216=CARTESIAN_POINT ( 'NONE',  ( -5.588711115410763597, 16.61483511785016987, -64.79999999999996874 ) ) ;
#11232=CARTESIAN_POINT ( 'NONE',  ( 5.107581180293630396, 15.06055038898570686, -56.09295307432605426 ) ) ;
#11241=CARTESIAN_POINT ( 'NONE',  ( -4.342430937695320736, 18.03316848959025620, -66.44295307432605568 ) ) ;
#11243=CARTESIAN_POINT ( 'NONE',  ( -2.983759233219601903, 20.69971185032686023, -54.75704692567386900 ) ) ;
#11255=CARTESIAN_POINT ( 'NONE',  ( 1.985016409143818272, 21.39581405818570303, -56.84999999999995879 ) ) ;
#11265=CARTESIAN_POINT ( 'NONE',  ( -4.342430937695320736, 18.03316848959025620, -72.44295307432605568 ) ) ;
#11277=CARTESIAN_POINT ( 'NONE',  ( -3.705139346311794313, 19.38786279086902198, -41.09999999999996589 ) ) ;
#11282=CARTESIAN_POINT ( 'NONE',  ( 3.091735541773220852, 14.40826445822673563, -30.74999999999995737 ) ) ;
#11290=CARTESIAN_POINT ( 'NONE',  ( 3.705139346311793869, 15.61213720913094960, -69.59999999999996589 ) ) ;
#11292=CARTESIAN_POINT ( 'NONE',  ( -4.975717084895059372, 20.19824746994243370, -57.60704692567387752 ) ) ;
#11293=CARTESIAN_POINT ( 'NONE',  ( -5.301103610786608300, 14.79895279989743528, -40.64999999999995595 ) ) ;
#11307=CARTESIAN_POINT ( 'NONE',  ( -5.370428668309080500, 14.93501088608579153, -33.15704692567386047 ) ) ;
#11310=CARTESIAN_POINT ( 'NONE',  ( 5.231778553264135212, 20.33710528629089254, -49.64295307432606563 ) ) ;
#11328=CARTESIAN_POINT ( 'NONE',  ( -3.898383833589191827, 13.39623302270000771, -74.99295307432603863 ) ) ;
#11331=CARTESIAN_POINT ( 'NONE',  ( -0.5331684895902242260, 21.84243093769531185, -46.05704692567387326 ) ) ;
#11332=CARTESIAN_POINT ( 'NONE',  ( -4.107178604518053611, 16.84948681541050775, -61.79999999999996874 ) ) ;
#11339=CARTESIAN_POINT ( 'NONE',  ( 4.107178604518054499, 18.15051318458946383, -48.29999999999996874 ) ) ;
#11342=CARTESIAN_POINT ( 'NONE',  ( -3.043106805520194413, 14.66227633819065623, -36.00704692567386189 ) ) ;
#11343=CARTESIAN_POINT ( 'NONE',  ( -0.9307174358028534877, 23.37631862003491889, -68.54999999999996874 ) ) ;
#11356=CARTESIAN_POINT ( 'NONE',  ( 4.103766977300021601, 21.39838383358913987, -61.50704692567389031 ) ) ;
#11361=CARTESIAN_POINT ( 'NONE',  ( -0.8851648821498765418, 11.91128888458923285, -31.19999999999996376 ) ) ;
#11378=CARTESIAN_POINT ( 'NONE',  ( -5.588711115410763597, 16.61483511785016987, -52.79999999999996874 ) ) ;
#11383=CARTESIAN_POINT ( 'NONE',  ( -4.318543150850367773, 18.18399003996480801, -25.94999999999996732 ) ) ;
#11384=CARTESIAN_POINT ( 'NONE',  ( -3.091735541773221296, 20.59173554177323950, -71.24999999999995737 ) ) ;
#11388=CARTESIAN_POINT ( 'NONE',  ( -4.107178604518053611, 16.84948681541050775, -70.79999999999996874 ) ) ;
#11393=CARTESIAN_POINT ( 'NONE',  ( 2.837723661809363307, 20.54310680552015356, -37.49295307432604574 ) ) ;
#11396=CARTESIAN_POINT ( 'NONE',  ( 3.771071394011080269, 15.74153613859503764, -53.09295307432605426 ) ) ;
#11410=CARTESIAN_POINT ( 'NONE',  ( -5.588711115410763597, 16.61483511785016987, -55.79999999999996874 ) ) ;
#11428=CARTESIAN_POINT ( 'NONE',  ( 0.7417250638684235176, 23.11142975074950101, -58.19295307432606279 ) ) ;
#11437=CARTESIAN_POINT ( 'NONE',  ( -4.342430937695320736, 18.03316848959025620, -60.44295307432605568 ) ) ;
#11439=CARTESIAN_POINT ( 'NONE',  ( 3.965139115708213868, 19.34895832295540430, -55.65704692567387468 ) ) ;
#11452=CARTESIAN_POINT ( 'NONE',  ( -1.985016409143819605, 13.60418594181426855, -46.34999999999997300 ) ) ;
#11462=CARTESIAN_POINT ( 'NONE',  ( -5.231778553264134324, 14.66289471370907727, -27.14295307432605853 ) ) ;
#11475=CARTESIAN_POINT ( 'NONE',  ( -0.6505131845895224529, 13.39282139548194195, -43.19999999999996732 ) ) ;
#11481=CARTESIAN_POINT ( 'NONE',  ( -0.6505131845895224529, 13.39282139548194195, -37.19999999999996732 ) ) ;
#11491=CARTESIAN_POINT ( 'NONE',  ( 1.887862790868997109, 13.79486065368817194, -51.89999999999997016 ) ) ;
#11492=CARTESIAN_POINT ( 'NONE',  ( 2.837105286290961370, 22.73177855326409613, -43.35704692567387752 ) ) ;
#11493=CARTESIAN_POINT ( 'NONE',  ( 0.8851648821498760977, 23.08871111541074228, -35.69999999999996732 ) ) ;
#11495=CARTESIAN_POINT ( 'NONE',  ( -3.091735541773221296, 20.59173554177323950, -71.24999999999994316 ) ) ;
#11506=CARTESIAN_POINT ( 'NONE',  ( -4.099003336600151925, 21.81495595370741469, -33.75704692567387610 ) ) ;
#11511=CARTESIAN_POINT ( 'NONE',  ( 5.900206406879871857, 16.72010411457162604, -55.94295307432605568 ) ) ;
#11528=CARTESIAN_POINT ( 'NONE',  ( -4.206979645153768210, 21.70697964515380107, -26.24999999999996803 ) ) ;
#11531=CARTESIAN_POINT ( 'NONE',  ( 2.121074495332174958, 21.32648900066323350, -46.35704692567385621 ) ) ;
#11532=CARTESIAN_POINT ( 'NONE',  ( 1.985016409143818272, 21.39581405818570303, -38.84999999999996589 ) ) ;
#11533=CARTESIAN_POINT ( 'NONE',  ( -1.887862790868997553, 21.20513934631180319, -68.39999999999997726 ) ) ;
#11543=CARTESIAN_POINT ( 'NONE',  ( 0.7798958854283032371, 11.59979359312010772, -71.55704692567385905 ) ) ;
#11544=CARTESIAN_POINT ( 'NONE',  ( -2.701047200102606460, 12.19889638921340591, -64.34999999999996589 ) ) ;
#11555=CARTESIAN_POINT ( 'NONE',  ( -5.370428668309080500, 14.93501088608579153, -63.15704692567388179 ) ) ;
#11559=CARTESIAN_POINT ( 'NONE',  ( -5.876318620034919782, 18.43071743580290089, -28.94999999999996021 ) ) ;
#11576=CARTESIAN_POINT ( 'NONE',  ( -0.9307174358028533767, 23.37631862003491889, -53.54999999999996163 ) ) ;
#11580=CARTESIAN_POINT ( 'NONE',  ( 2.940415233664778416, 20.44041523366473712, -26.99999999999996803 ) ) ;
#11581=CARTESIAN_POINT ( 'NONE',  ( 1.985016409143818272, 21.39581405818570659, -53.84999999999995879 ) ) ;
#11593=CARTESIAN_POINT ( 'NONE',  ( 1.848958322955461808, 21.46513911570817612, -37.34295307432606137 ) ) ;
#11596=CARTESIAN_POINT ( 'NONE',  ( 4.342430937695320736, 16.96683151040971538, -52.94295307432605568 ) ) ;
#11614=CARTESIAN_POINT ( 'NONE',  ( -4.001075405444606936, 13.49892459455542060, -55.49999999999996447 ) ) ;
#11634=CARTESIAN_POINT ( 'NONE',  ( 5.107581180293630396, 15.06055038898570686, -47.09295307432606137 ) ) ;
#11643=CARTESIAN_POINT ( 'NONE',  ( 3.771071394011080269, 15.74153613859503764, -65.09295307432604716 ) ) ;
#11656=CARTESIAN_POINT ( 'NONE',  ( 2.940415233664778416, 20.44041523366473712, -44.99999999999997158 ) ) ;
#11682=CARTESIAN_POINT ( 'NONE',  ( 1.887862790868997109, 13.79486065368817194, -42.89999999999996305 ) ) ;
#11686=CARTESIAN_POINT ( 'NONE',  ( -1.985016409143819605, 13.60418594181426855, -34.34999999999995879 ) ) ;
#11694=CARTESIAN_POINT ( 'NONE',  ( -4.318543150850367773, 18.18399003996480801, -52.94999999999994600 ) ) ;
#11697=CARTESIAN_POINT ( 'NONE',  ( 5.611429750749524992, 18.24172506386835479, -43.80704692567387326 ) ) ;
#11698=CARTESIAN_POINT ( 'NONE',  ( -0.9307174358028534877, 23.37631862003491889, -38.54999999999996874 ) ) ;
#11701=CARTESIAN_POINT ( 'NONE',  ( -1.848958322955462474, 13.53486088429179546, -29.84295307432605782 ) ) ;
#11713=CARTESIAN_POINT ( 'NONE',  ( 5.852430833189966819, 16.41846101382252243, -37.95704692567387184 ) ) ;
#11717=CARTESIAN_POINT ( 'NONE',  ( 5.107581180293630396, 15.06055038898570686, -56.09295307432605426 ) ) ;
#11737=CARTESIAN_POINT ( 'NONE',  ( 0.7417250638684235176, 23.11142975074950101, -76.19295307432606990 ) ) ;
#11741=CARTESIAN_POINT ( 'NONE',  ( -2.983759233219601903, 20.69971185032686023, -42.75704692567387610 ) ) ;
#11742=CARTESIAN_POINT ( 'NONE',  ( 1.887862790868997109, 13.79486065368817194, -33.89999999999996305 ) ) ;
#11743=CARTESIAN_POINT ( 'NONE',  ( 4.318543150850367773, 16.81600996003516357, -60.44999999999997442 ) ) ;
#11752=CARTESIAN_POINT ( 'NONE',  ( 0.5331684895902240040, 13.15756906230466328, -26.55704692567386971 ) ) ;
#11753=CARTESIAN_POINT ( 'NONE',  ( -5.876318620034919782, 18.43071743580290089, -61.94999999999996732 ) ) ;
#11766=CARTESIAN_POINT ( 'NONE',  ( -4.975717084895059372, 20.19824746994243370, -60.60704692567387752 ) ) ;
#11771=CARTESIAN_POINT ( 'NONE',  ( 2.701047200102605572, 22.80110361078655856, -29.84999999999996589 ) ) ;
#11789=CARTESIAN_POINT ( 'NONE',  ( 5.588711115410763597, 18.38516488214980882, -51.29999999999996874 ) ) ;
#11793=CARTESIAN_POINT ( 'NONE',  ( 1.985016409143818272, 21.39581405818570303, -26.84999999999995524 ) ) ;
#11794=CARTESIAN_POINT ( 'NONE',  ( -0.6839900399647738105, 21.81854315085035623, -62.54999999999996874 ) ) ;
#11805=CARTESIAN_POINT ( 'NONE',  ( -3.826489000663265472, 15.37892550466785480, -36.14295307432605142 ) ) ;
#11808=CARTESIAN_POINT ( 'NONE',  ( 2.837723661809363307, 20.54310680552015356, -52.49295307432605995 ) ) ;
#11824=CARTESIAN_POINT ( 'NONE',  ( -5.041649132594344884, 20.06884854047834921, -56.09999999999996589 ) ) ;
#11844=CARTESIAN_POINT ( 'NONE',  ( 5.900206406879871857, 16.72010411457162604, -43.94295307432605568 ) ) ;
#11853=CARTESIAN_POINT ( 'NONE',  ( -4.084459969179292216, 16.70604699712905372, -69.29295307432606421 ) ) ;
#11869=CARTESIAN_POINT ( 'NONE',  ( -1.887862790868997553, 21.20513934631180319, -44.39999999999997016 ) ) ;
#11896=CARTESIAN_POINT ( 'NONE',  ( 4.318543150850366885, 16.81600996003516713, -36.44999999999996732 ) ) ;
#11899=CARTESIAN_POINT ( 'NONE',  ( 3.705139346311793869, 15.61213720913094960, -36.59999999999996589 ) ) ;
#11907=CARTESIAN_POINT ( 'NONE',  ( -0.6839900399647736995, 21.81854315085035623, -59.54999999999994742 ) ) ;
#11910=CARTESIAN_POINT ( 'NONE',  ( -5.370428668309080500, 14.93501088608579153, -45.15704692567388179 ) ) ;
#11911=CARTESIAN_POINT ( 'NONE',  ( -4.206979645153769098, 21.70697964515380107, -32.24999999999995737 ) ) ;
#11913=CARTESIAN_POINT ( 'NONE',  ( -3.826489000663265472, 15.37892550466785480, -27.14295307432605853 ) ) ;
#11925=CARTESIAN_POINT ( 'NONE',  ( -5.301103610786608300, 14.79895279989743706, -73.64999999999993463 ) ) ;
#11930=CARTESIAN_POINT ( 'NONE',  ( 5.107581180293630396, 15.06055038898570686, -50.09295307432605426 ) ) ;
#11949=CARTESIAN_POINT ( 'NONE',  ( -5.876318620034919782, 18.43071743580290089, -25.94999999999996732 ) ) ;
#11953=CARTESIAN_POINT ( 'NONE',  ( -4.129897239856814117, 16.99292663369196177, -39.30704692567388037 ) ) ;
#11954=CARTESIAN_POINT ( 'NONE',  ( 3.895814058185739448, 19.48501640914375344, -39.14999999999997016 ) ) ;
#11955=CARTESIAN_POINT ( 'NONE',  ( -0.6505131845895224529, 13.39282139548194195, -61.19999999999996732 ) ) ;
#11967=CARTESIAN_POINT ( 'NONE',  ( -5.370428668309080500, 14.93501088608579153, -72.15704692567386758 ) ) ;
#11968=CARTESIAN_POINT ( 'NONE',  ( 5.041649132594343996, 14.93115145952162415, -69.59999999999996589 ) ) ;
#11978=CARTESIAN_POINT ( 'NONE',  ( 5.611429750749524992, 18.24172506386835479, -67.80704692567387326 ) ) ;
#11982=CARTESIAN_POINT ( 'NONE',  ( -4.206979645153768210, 21.70697964515380107, -29.24999999999996447 ) ) ;
#12000=CARTESIAN_POINT ( 'NONE',  ( -0.8851648821498765418, 11.91128888458923285, -52.19999999999996732 ) ) ;
#12004=CARTESIAN_POINT ( 'NONE',  ( -4.107178604518053611, 16.84948681541050775, -25.79999999999996163 ) ) ;
#12005=CARTESIAN_POINT ( 'NONE',  ( 2.940415233664778416, 20.44041523366473712, -56.99999999999996447 ) ) ;
#12011=CARTESIAN_POINT ( 'NONE',  ( -1.887862790868997553, 21.20513934631180319, -74.39999999999996305 ) ) ;
#12015=CARTESIAN_POINT ( 'NONE',  ( 4.084459969179292216, 18.29395300287091430, -34.79295307432605711 ) ) ;
#12018=CARTESIAN_POINT ( 'NONE',  ( 0.8348115903393232839, 13.20534463599456387, -41.54295307432605000 ) ) ;
#12033=CARTESIAN_POINT ( 'NONE',  ( 5.041649132594343996, 14.93115145952162415, -57.59999999999997300 ) ) ;
#12054=CARTESIAN_POINT ( 'NONE',  ( 0.7417250638684235176, 23.11142975074950101, -46.19295307432605568 ) ) ;
#12061=CARTESIAN_POINT ( 'NONE',  ( 3.771071394011080269, 15.74153613859503764, -68.09295307432604716 ) ) ;
#12074=CARTESIAN_POINT ( 'NONE',  ( 1.985016409143818272, 21.39581405818570303, -47.84999999999994458 ) ) ;
#12100=CARTESIAN_POINT ( 'NONE',  ( -3.091735541773221296, 20.59173554177323950, -29.24999999999996447 ) ) ;
#12105=CARTESIAN_POINT ( 'NONE',  ( -3.091735541773221296, 20.59173554177323950, -35.24999999999997158 ) ) ;
#12113=CARTESIAN_POINT ( 'NONE',  ( 1.985016409143818272, 21.39581405818570303, -53.84999999999995879 ) ) ;
#12115=CARTESIAN_POINT ( 'NONE',  ( -4.103766977300021601, 13.60161616641083704, -48.00704692567387610 ) ) ;
#12116=CARTESIAN_POINT ( 'NONE',  ( -5.588711115410763597, 16.61483511785016987, -37.79999999999996874 ) ) ;
#12118=CARTESIAN_POINT ( 'NONE',  ( 2.017261720333081598, 13.86079270138745834, -29.39295307432606208 ) ) ;
#12128=CARTESIAN_POINT ( 'NONE',  ( -5.611429750749524992, 16.75827493613162034, -27.30704692567386971 ) ) ;
#12135=CARTESIAN_POINT ( 'NONE',  ( -0.7417250638684240727, 11.88857024925047057, -41.69295307432606279 ) ) ;
#12156=CARTESIAN_POINT ( 'NONE',  ( -2.564989113914250662, 12.12957133169093282, -71.84295307432606137 ) ) ;
#12161=CARTESIAN_POINT ( 'NONE',  ( -0.6839900399647736995, 21.81854315085035623, -35.54999999999994742 ) ) ;
#12162=CARTESIAN_POINT ( 'NONE',  ( 4.318543150850367773, 16.81600996003516357, -66.44999999999997442 ) ) ;
#12173=CARTESIAN_POINT ( 'NONE',  ( 4.975717084895059372, 14.80175253005754143, -71.10704692567387042 ) ) ;
#12174=CARTESIAN_POINT ( 'NONE',  ( 5.301103610786608300, 20.20104720010254340, -66.14999999999997726 ) ) ;
#12188=CARTESIAN_POINT ( 'NONE',  ( 2.439449611014226971, 12.39241881970633230, -59.40704692567388179 ) ) ;
#12191=CARTESIAN_POINT ( 'NONE',  ( -5.900206406879871857, 18.27989588542834554, -66.44295307432605568 ) ) ;
#12209=CARTESIAN_POINT ( 'NONE',  ( 5.041649132594343996, 14.93115145952162415, -51.59999999999996589 ) ) ;
#12213=CARTESIAN_POINT ( 'NONE',  ( -4.294655364005415699, 18.33481159033935626, -63.45704692567386473 ) ) ;
#12214=CARTESIAN_POINT ( 'NONE',  ( 3.091735541773220852, 14.40826445822673740, -57.74999999999996447 ) ) ;
#12220=CARTESIAN_POINT ( 'NONE',  ( 4.318543150850367773, 16.81600996003516357, -72.44999999999994600 ) ) ;
#12222=CARTESIAN_POINT ( 'NONE',  ( 3.043106805520193525, 20.33772366180932067, -55.50704692567387610 ) ) ;
#12225=CARTESIAN_POINT ( 'NONE',  ( 2.837723661809363307, 20.54310680552015356, -31.49295307432605995 ) ) ;
#12229=CARTESIAN_POINT ( 'NONE',  ( 2.837723661809363307, 20.54310680552015356, -43.49295307432606705 ) ) ;
#12245=CARTESIAN_POINT ( 'NONE',  ( 0.9307174358028528216, 11.62368137996505801, -55.04999999999995453 ) ) ;
#12259=CIRCLE ( 'NONE', #23846, 0.7500000000000009992 ) ;
#12266=CARTESIAN_POINT ( 'NONE',  ( 3.898383833589191383, 21.60376697729997275, -43.49295307432606705 ) ) ;
#12275=CARTESIAN_POINT ( 'NONE',  ( 1.848958322955461808, 21.46513911570817612, -52.34295307432604716 ) ) ;
#12290=CARTESIAN_POINT ( 'NONE',  ( -0.6839900399647736995, 21.81854315085035623, -32.54999999999996163 ) ) ;
#12300=EDGE_CURVE ( 'NONE', #3983, #4513, #39825, .T. ) ;
#12317=CARTESIAN_POINT ( 'NONE',  ( 0.6839900399647732554, 13.18145684914961357, -31.04999999999996163 ) ) ;
#12321=CARTESIAN_POINT ( 'NONE',  ( 5.231778553264135212, 20.33710528629089254, -31.64295307432605853 ) ) ;
#12322=CARTESIAN_POINT ( 'NONE',  ( 2.940415233664778416, 20.44041523366473712, -29.99999999999996447 ) ) ;
#12330=CARTESIAN_POINT ( 'NONE',  ( -0.6505131845895224529, 13.39282139548194195, -55.19999999999997442 ) ) ;
#12333=CARTESIAN_POINT ( 'NONE',  ( -5.611429750749524992, 16.75827493613162034, -33.30704692567387326 ) ) ;
#12334=CARTESIAN_POINT ( 'NONE',  ( 2.701047200102605128, 22.80110361078656211, -29.84999999999996589 ) ) ;
#12335=CARTESIAN_POINT ( 'NONE',  ( -4.084459969179292216, 16.70604699712905372, -27.29295307432605355 ) ) ;
#12347=CARTESIAN_POINT ( 'NONE',  ( 0.7798958854283032371, 11.59979359312010772, -29.55704692567387681 ) ) ;
#12354=CARTESIAN_POINT ( 'NONE',  ( 0.7417250638684235176, 23.11142975074950101, -40.19295307432605568 ) ) ;
#12371=CARTESIAN_POINT ( 'NONE',  ( -5.231778553264134324, 14.66289471370907727, -69.14295307432605853 ) ) ;
#12377=CARTESIAN_POINT ( 'NONE',  ( -3.895814058185739448, 15.51498359085620571, -34.64999999999997016 ) ) ;
#12379=CARTESIAN_POINT ( 'NONE',  ( -1.887862790868997553, 21.20513934631180319, -56.39999999999996305 ) ) ;
#12391=CARTESIAN_POINT ( 'NONE',  ( 2.121074495332174958, 21.32648900066323350, -28.35704692567387397 ) ) ;
#12392=CARTESIAN_POINT ( 'NONE',  ( 4.206979645153768210, 13.29302035484617406, -51.74999999999995026 ) ) ;
#12402=CARTESIAN_POINT ( 'NONE',  ( -2.439449611014227859, 22.60758118029364283, -51.90704692567388179 ) ) ;
#12407=CARTESIAN_POINT ( 'NONE',  ( -3.898383833589191827, 13.39623302270000771, -71.99295307432603863 ) ) ;
#12424=CARTESIAN_POINT ( 'NONE',  ( -5.301103610786608300, 14.79895279989743706, -37.64999999999996305 ) ) ;
#12428=CARTESIAN_POINT ( 'NONE',  ( -0.7939530028709754772, 13.41554003082070246, -62.70704692567387184 ) ) ;
#12429=CARTESIAN_POINT ( 'NONE',  ( 1.985016409143818272, 21.39581405818570659, -59.84999999999996589 ) ) ;
#12437=CARTESIAN_POINT ( 'NONE',  ( -3.895814058185739448, 15.51498359085620571, -61.64999999999995595 ) ) ;
#12441=CARTESIAN_POINT ( 'NONE',  ( 4.294655364005415699, 16.66518840966061887, -55.95704692567386473 ) ) ;
#12444=CARTESIAN_POINT ( 'NONE',  ( -3.826489000663265472, 15.37892550466785480, -30.14295307432606208 ) ) ;
#12448=CARTESIAN_POINT ( 'NONE',  ( -2.017261720333081598, 21.13920729861251857, -45.89295307432605853 ) ) ;
#12463=CARTESIAN_POINT ( 'NONE',  ( -4.001075405444606936, 13.49892459455542060, -46.49999999999997158 ) ) ;
#12482=CARTESIAN_POINT ( 'NONE',  ( 0.6839900399647733664, 13.18145684914961357, -43.04999999999996163 ) ) ;
#12483=CARTESIAN_POINT ( 'NONE',  ( -5.231778553264134324, 14.66289471370907727, -45.14295307432605853 ) ) ;
#12492=CARTESIAN_POINT ( 'NONE',  ( -4.084459969179292216, 16.70604699712905372, -54.29295307432607132 ) ) ;
#12510=CARTESIAN_POINT ( 'NONE',  ( -3.895814058185739448, 15.51498359085620571, -37.64999999999996305 ) ) ;
#12536=CARTESIAN_POINT ( 'NONE',  ( 2.564989113914249330, 22.87042866830903876, -37.34295307432606137 ) ) ;
#12537=CARTESIAN_POINT ( 'NONE',  ( 0.6839900399647733664, 13.18145684914961357, -28.04999999999995453 ) ) ;
#12544=CARTESIAN_POINT ( 'NONE',  ( -0.6839900399647736995, 21.81854315085035623, -41.54999999999996874 ) ) ;
#12547=CARTESIAN_POINT ( 'NONE',  ( -4.975717084895059372, 20.19824746994243370, -33.60704692567387042 ) ) ;
#12548=CARTESIAN_POINT ( 'NONE',  ( -4.001075405444606936, 13.49892459455542060, -28.49999999999996447 ) ) ;
#12549=CARTESIAN_POINT ( 'NONE',  ( -2.940415233664778860, 14.55958476633523802, -64.49999999999997158 ) ) ;
#12560=CARTESIAN_POINT ( 'NONE',  ( -5.611429750749524992, 16.75827493613162034, -30.30704692567387326 ) ) ;
#12566=CARTESIAN_POINT ( 'NONE',  ( 2.564989113914249330, 22.87042866830903876, -46.34295307432606137 ) ) ;
#12583=CARTESIAN_POINT ( 'NONE',  ( 5.565992480072003978, 18.52860470043125574, -61.79295307432605000 ) ) ;
#12589=CARTESIAN_POINT ( 'NONE',  ( -1.887862790868997553, 21.20513934631180319, -29.39999999999996660 ) ) ;
#12590=CARTESIAN_POINT ( 'NONE',  ( -3.091735541773221296, 20.59173554177323950, -53.24999999999996447 ) ) ;
#12603=CARTESIAN_POINT ( 'NONE',  ( 5.611429750749524992, 18.24172506386835479, -61.80704692567387326 ) ) ;
#12604=CARTESIAN_POINT ( 'NONE',  ( 4.001075405444606048, 21.50107540544455276, -53.99999999999996447 ) ) ;
#12615=CARTESIAN_POINT ( 'NONE',  ( 4.103766977300021601, 21.39838383358913987, -55.50704692567387610 ) ) ;
#12621=CARTESIAN_POINT ( 'NONE',  ( 2.698247469942395949, 12.52428291510489977, -74.39295307432605853 ) ) ;
#12636=CARTESIAN_POINT ( 'NONE',  ( 0.9307174358028528216, 11.62368137996505801, -46.04999999999996163 ) ) ;
#12640=CARTESIAN_POINT ( 'NONE',  ( -3.043106805520194413, 14.66227633819065623, -66.00704692567386189 ) ) ;
#12641=CARTESIAN_POINT ( 'NONE',  ( -3.895814058185739892, 15.51498359085620748, -49.64999999999995595 ) ) ;
#12653=CARTESIAN_POINT ( 'NONE',  ( 0.6505131845895220088, 21.60717860451803674, -65.69999999999996021 ) ) ;
#12655=CARTESIAN_POINT ( 'NONE',  ( 0.7939530028709752552, 21.58445996917927445, -43.20704692567387184 ) ) ;
#12658=CARTESIAN_POINT ( 'NONE',  ( 0.8348115903393232839, 13.20534463599456387, -29.54295307432605355 ) ) ;
#12661=CARTESIAN_POINT ( 'NONE',  ( -1.848958322955462474, 13.53486088429179546, -47.84295307432606137 ) ) ;
#12675=CARTESIAN_POINT ( 'NONE',  ( -0.9307174358028533767, 23.37631862003491889, -44.54999999999994742 ) ) ;
#12690=CARTESIAN_POINT ( 'NONE',  ( -4.001075405444606936, 13.49892459455542060, -70.49999999999997158 ) ) ;
#12696=CARTESIAN_POINT ( 'NONE',  ( 3.705139346311793869, 15.61213720913094960, -42.59999999999996589 ) ) ;
#12697=CARTESIAN_POINT ( 'NONE',  ( 3.705139346311793869, 15.61213720913094960, -72.59999999999996589 ) ) ;
#12707=CARTESIAN_POINT ( 'NONE',  ( 3.199711850326839357, 14.51624076678035635, -53.24295307432605995 ) ) ;
#12722=CARTESIAN_POINT ( 'NONE',  ( 4.318543150850367773, 16.81600996003516357, -39.44999999999994600 ) ) ;
#12745=CARTESIAN_POINT ( 'NONE',  ( 0.5331684895902240040, 13.15756906230466328, -32.55704692567387326 ) ) ;
#12746=CARTESIAN_POINT ( 'NONE',  ( -3.091735541773221296, 20.59173554177323950, -26.24999999999996803 ) ) ;
#12749=CARTESIAN_POINT ( 'NONE',  ( 5.900206406879871857, 16.72010411457162604, -34.94295307432605568 ) ) ;
#12750=CARTESIAN_POINT ( 'NONE',  ( -4.318543150850367773, 18.18399003996480801, -25.94999999999996732 ) ) ;
#12757=CARTESIAN_POINT ( 'NONE',  ( 3.895814058185739448, 19.48501640914375344, -45.14999999999994884 ) ) ;
#12760=CARTESIAN_POINT ( 'NONE',  ( 4.103766977300021601, 21.39838383358913987, -37.50704692567386189 ) ) ;
#12761=CARTESIAN_POINT ( 'NONE',  ( 5.301103610786608300, 20.20104720010254340, -30.14999999999997016 ) ) ;
#12762=CARTESIAN_POINT ( 'NONE',  ( 3.091735541773220852, 14.40826445822673563, -66.74999999999997158 ) ) ;
#12775=CARTESIAN_POINT ( 'NONE',  ( 2.698247469942395949, 12.52428291510489977, -38.39295307432605142 ) ) ;
#12789=CARTESIAN_POINT ( 'NONE',  ( 5.107581180293630396, 15.06055038898570686, -68.09295307432604716 ) ) ;
#12795=CARTESIAN_POINT ( 'NONE',  ( -2.940415233664778860, 14.55958476633523802, -55.49999999999996447 ) ) ;
#12806=CARTESIAN_POINT ( 'NONE',  ( 0.7798958854283032371, 11.59979359312010772, -68.55704692567387326 ) ) ;
#12807=CARTESIAN_POINT ( 'NONE',  ( -5.041649132594344884, 20.06884854047834921, -53.09999999999996589 ) ) ;
#12821=CARTESIAN_POINT ( 'NONE',  ( -4.103766977300021601, 13.60161616641083704, -51.00704692567387610 ) ) ;
#12824=CARTESIAN_POINT ( 'NONE',  ( -1.081538986177402961, 23.35243083318996327, -67.04295307432605000 ) ) ;
#12842=CARTESIAN_POINT ( 'NONE',  ( 4.001075405444606048, 21.50107540544455276, -41.99999999999996447 ) ) ;
#12846=CARTESIAN_POINT ( 'NONE',  ( 3.965139115708213868, 19.34895832295540430, -61.65704692567387468 ) ) ;
#12847=CARTESIAN_POINT ( 'NONE',  ( 1.887862790868997109, 13.79486065368817194, -48.89999999999997016 ) ) ;
#12859=CARTESIAN_POINT ( 'NONE',  ( -1.985016409143819605, 13.60418594181426855, -61.34999999999996589 ) ) ;
#12861=CARTESIAN_POINT ( 'NONE',  ( 1.758463861404912620, 13.72892860598888731, -47.40704692567387468 ) ) ;
#12866=CARTESIAN_POINT ( 'NONE',  ( -2.837723661809363751, 14.45689319447982335, -41.99295307432605995 ) ) ;
#12882=CARTESIAN_POINT ( 'NONE',  ( 4.001075405444606048, 21.50107540544455276, -44.99999999999997158 ) ) ;
#12898=CARTESIAN_POINT ( 'NONE',  ( -2.701047200102606016, 12.19889638921340413, -73.34999999999996589 ) ) ;
#12903=CARTESIAN_POINT ( 'NONE',  ( -2.940415233664778860, 14.55958476633523802, -40.49999999999996447 ) ) ;
#12904=CARTESIAN_POINT ( 'NONE',  ( 1.985016409143818272, 21.39581405818570659, -74.84999999999995168 ) ) ;
#12914=CARTESIAN_POINT ( 'NONE',  ( 3.826489000663266360, 19.62107449533211678, -52.64295307432606563 ) ) ;
#12931=CARTESIAN_POINT ( 'NONE',  ( -1.887862790868997553, 21.20513934631180319, -32.39999999999996305 ) ) ;
#12955=CARTESIAN_POINT ( 'NONE',  ( -3.043106805520194413, 14.66227633819065623, -33.00704692567387610 ) ) ;
#12959=CARTESIAN_POINT ( 'NONE',  ( -4.314955953707389824, 21.59900333660018390, -36.74295307432605995 ) ) ;
#12960=CARTESIAN_POINT ( 'NONE',  ( -4.294655364005415699, 18.33481159033935626, -72.45704692567387895 ) ) ;
#12969=CARTESIAN_POINT ( 'NONE',  ( -2.940415233664778860, 14.55958476633523802, -43.49999999999997158 ) ) ;
#12972=CARTESIAN_POINT ( 'NONE',  ( -1.028604700431329233, 11.93400751992799513, -38.70704692567387184 ) ) ;
#12973=CARTESIAN_POINT ( 'NONE',  ( 5.301103610786608300, 20.20104720010254340, -27.14999999999996305 ) ) ;
#12974=CARTESIAN_POINT ( 'NONE',  ( 4.107178604518054499, 18.15051318458946383, -63.29999999999996874 ) ) ;
#12977=ORIENTED_EDGE ( 'NONE', *, *, #2342, .F. ) ;
#12989=CARTESIAN_POINT ( 'NONE',  ( 0.7417250638684235176, 23.11142975074950101, -37.19295307432606279 ) ) ;
#13010=CARTESIAN_POINT ( 'NONE',  ( -4.107178604518053611, 16.84948681541050775, -52.79999999999996874 ) ) ;
#13020=CARTESIAN_POINT ( 'NONE',  ( -5.852430833189966819, 18.58153898617744915, -66.45704692567387895 ) ) ;
#13021=CARTESIAN_POINT ( 'NONE',  ( 0.9307174358028527106, 11.62368137996505801, -52.04999999999996874 ) ) ;
#13034=CARTESIAN_POINT ( 'NONE',  ( -4.975717084895059372, 20.19824746994243370, -42.60704692567387752 ) ) ;
#13038=CARTESIAN_POINT ( 'NONE',  ( -5.565992480072003978, 16.47139529956871229, -72.29295307432605000 ) ) ;
#13051=CARTESIAN_POINT ( 'NONE',  ( -4.206979645153768210, 21.70697964515380107, -38.24999999999996447 ) ) ;
#13054=CARTESIAN_POINT ( 'NONE',  ( 0.7939530028709752552, 21.58445996917927445, -67.20704692567387895 ) ) ;
#13055=CARTESIAN_POINT ( 'NONE',  ( -2.940415233664778860, 14.55958476633523802, -46.49999999999997158 ) ) ;
#13065=CARTESIAN_POINT ( 'NONE',  ( 0.6839900399647733664, 13.18145684914961357, -67.04999999999994031 ) ) ;
#13067=CARTESIAN_POINT ( 'NONE',  ( 2.121074495332174958, 21.32648900066323350, -46.35704692567385621 ) ) ;
#13071=CARTESIAN_POINT ( 'NONE',  ( 1.848958322955461808, 21.46513911570817612, -40.34295307432606137 ) ) ;
#13086=CARTESIAN_POINT ( 'NONE',  ( 2.568848540478311460, 12.45835086740561692, -48.89999999999997016 ) ) ;
#13100=CARTESIAN_POINT ( 'NONE',  ( -0.8851648821498765418, 11.91128888458923285, -73.19999999999997442 ) ) ;
#13106=CARTESIAN_POINT ( 'NONE',  ( 2.940415233664778416, 20.44041523366473712, -41.99999999999996447 ) ) ;
#13121=CARTESIAN_POINT ( 'NONE',  ( 3.771071394011080269, 15.74153613859503764, -56.09295307432605426 ) ) ;
#13136=CARTESIAN_POINT ( 'NONE',  ( -3.091735541773221296, 20.59173554177323950, -32.24999999999996447 ) ) ;
#13161=CARTESIAN_POINT ( 'NONE',  ( -2.121074495332175847, 13.67351099933674341, -32.85704692567387752 ) ) ;
#13166=CARTESIAN_POINT ( 'NONE',  ( -1.081538986177402961, 23.35243083318996327, -37.04295307432605711 ) ) ;
#13167=CARTESIAN_POINT ( 'NONE',  ( -3.043106805520194413, 14.66227633819065623, -72.00704692567386189 ) ) ;
#13175=CARTESIAN_POINT ( 'NONE',  ( -3.091735541773221296, 20.59173554177323950, -44.24999999999997868 ) ) ;
#13178=CARTESIAN_POINT ( 'NONE',  ( -4.975717084895059372, 20.19824746994243370, -39.60704692567387042 ) ) ;
#13180=CARTESIAN_POINT ( 'NONE',  ( 2.940415233664778416, 20.44041523366473712, -62.99999999999997158 ) ) ;
#13192=CARTESIAN_POINT ( 'NONE',  ( -5.231778553264134324, 14.66289471370907727, -30.14295307432606208 ) ) ;
#13215=CARTESIAN_POINT ( 'NONE',  ( 4.318543150850367773, 16.81600996003516357, -54.44999999999996021 ) ) ;
#13225=CARTESIAN_POINT ( 'NONE',  ( 5.852430833189966819, 16.41846101382252243, -67.95704692567387895 ) ) ;
#13226=CARTESIAN_POINT ( 'NONE',  ( -0.9307174358028534877, 23.37631862003491889, -59.54999999999995453 ) ) ;
#13242=CARTESIAN_POINT ( 'NONE',  ( 5.370428668309080500, 20.06498911391418360, -46.65704692567388179 ) ) ;
#13246=CARTESIAN_POINT ( 'NONE',  ( 1.081538986177402295, 11.64756916681001186, -59.54295307432605711 ) ) ;
#13262=CARTESIAN_POINT ( 'NONE',  ( -2.701047200102606016, 12.19889638921340413, -46.34999999999997300 ) ) ;
#13266=CARTESIAN_POINT ( 'NONE',  ( -4.129897239856814117, 16.99292663369196177, -57.30704692567387326 ) ) ;
#13267=CARTESIAN_POINT ( 'NONE',  ( -4.107178604518053611, 16.84948681541050775, -46.79999999999996874 ) ) ;
#13276=CARTESIAN_POINT ( 'NONE',  ( 1.985016409143818272, 21.39581405818570303, -59.84999999999996589 ) ) ;
#13278=CARTESIAN_POINT ( 'NONE',  ( 0.5331684895902240040, 13.15756906230466328, -47.55704692567388037 ) ) ;
#13282=CARTESIAN_POINT ( 'NONE',  ( 2.017261720333081598, 13.86079270138745834, -38.39295307432605142 ) ) ;
#13288=CARTESIAN_POINT ( 'NONE',  ( -0.5331684895902242260, 21.84243093769531185, -25.05704692567386971 ) ) ;
#13296=CARTESIAN_POINT ( 'NONE',  ( 0.9307174358028528216, 11.62368137996505801, -52.04999999999997584 ) ) ;
#13312=CARTESIAN_POINT ( 'NONE',  ( 4.001075405444606048, 21.50107540544455276, -71.99999999999997158 ) ) ;
#13317=CARTESIAN_POINT ( 'NONE',  ( 4.318543150850367773, 16.81600996003516357, -39.44999999999994600 ) ) ;
#13329=CARTESIAN_POINT ( 'NONE',  ( -3.771071394011080269, 19.25846386140493394, -48.59295307432606847 ) ) ;
#13335=CARTESIAN_POINT ( 'NONE',  ( 2.837723661809363307, 20.54310680552015356, -61.49295307432606705 ) ) ;
#13353=CARTESIAN_POINT ( 'NONE',  ( -4.103766977300021601, 13.60161616641083704, -27.00704692567387610 ) ) ;
#13370=CARTESIAN_POINT ( 'NONE',  ( -2.983759233219601903, 20.69971185032686023, -36.75704692567386900 ) ) ;
#13374=CARTESIAN_POINT ( 'NONE',  ( 4.314955953707388936, 13.40099666339979123, -29.24295307432605640 ) ) ;
#13376=CARTESIAN_POINT ( 'NONE',  ( -4.294655364005415699, 18.33481159033935626, -63.45704692567386473 ) ) ;
#13384=CARTESIAN_POINT ( 'NONE',  ( -3.895814058185739448, 15.51498359085620571, -43.64999999999996305 ) ) ;
#13387=CARTESIAN_POINT ( 'NONE',  ( -0.7798958854283041253, 23.40020640687986386, -25.05704692567386971 ) ) ;
#13389=CARTESIAN_POINT ( 'NONE',  ( -0.6839900399647736995, 21.81854315085035623, -68.54999999999998295 ) ) ;
#13399=CARTESIAN_POINT ( 'NONE',  ( -3.898383833589191827, 13.39623302270000771, -32.99295307432605995 ) ) ;
#13415=CARTESIAN_POINT ( 'NONE',  ( 0.6505131845895220088, 21.60717860451803674, -26.69999999999996732 ) ) ;
#13416=CARTESIAN_POINT ( 'NONE',  ( -1.887862790868997553, 21.20513934631180319, -41.39999999999996305 ) ) ;
#13424=CARTESIAN_POINT ( 'NONE',  ( -1.848958322955462474, 13.53486088429179546, -29.84295307432605782 ) ) ;
#13426=CARTESIAN_POINT ( 'NONE',  ( 2.439449611014226971, 12.39241881970633230, -65.40704692567388179 ) ) ;
#13427=CARTESIAN_POINT ( 'NONE',  ( -4.206979645153769098, 21.70697964515380107, -44.24999999999997868 ) ) ;
#13442=CARTESIAN_POINT ( 'NONE',  ( 5.611429750749524992, 18.24172506386835479, -40.80704692567388037 ) ) ;
#13446=CARTESIAN_POINT ( 'NONE',  ( 0.7417250638684235176, 23.11142975074950101, -58.19295307432606279 ) ) ;
#13460=CARTESIAN_POINT ( 'NONE',  ( -2.701047200102606016, 12.19889638921340413, -28.34999999999995524 ) ) ;
#13463=CARTESIAN_POINT ( 'NONE',  ( 2.121074495332174958, 21.32648900066323350, -49.35704692567387042 ) ) ;
#13464=CARTESIAN_POINT ( 'NONE',  ( 4.318543150850366885, 16.81600996003516713, -51.44999999999996732 ) ) ;
#13475=CARTESIAN_POINT ( 'NONE',  ( 4.107178604518054499, 18.15051318458946383, -51.29999999999996874 ) ) ;
#13477=CARTESIAN_POINT ( 'NONE',  ( 4.294655364005415699, 16.66518840966061887, -46.95704692567387184 ) ) ;
#13481=CARTESIAN_POINT ( 'NONE',  ( -0.8348115903393239501, 21.79465536400541126, -40.04295307432605000 ) ) ;
#13488=CARTESIAN_POINT ( 'NONE',  ( 2.983759233219601459, 14.30028814967311668, -26.25704692567387255 ) ) ;
#13494=CARTESIAN_POINT ( 'NONE',  ( 5.588711115410763597, 18.38516488214980882, -39.29999999999996874 ) ) ;
#13514=CARTESIAN_POINT ( 'NONE',  ( -4.001075405444606936, 13.49892459455542060, -67.49999999999995737 ) ) ;
#13519=CARTESIAN_POINT ( 'NONE',  ( -4.107178604518053611, 16.84948681541050775, -31.79999999999996874 ) ) ;
#13520=CARTESIAN_POINT ( 'NONE',  ( -0.6505131845895224529, 13.39282139548194195, -73.19999999999997442 ) ) ;
#13530=CARTESIAN_POINT ( 'NONE',  ( 4.342430937695320736, 16.96683151040971538, -49.94295307432606279 ) ) ;
#13536=CARTESIAN_POINT ( 'NONE',  ( 4.084459969179292216, 18.29395300287091430, -67.79295307432606421 ) ) ;
#13556=CARTESIAN_POINT ( 'NONE',  ( 4.001075405444606048, 21.50107540544455276, -62.99999999999997158 ) ) ;
#13561=( BOUNDED_SURFACE ( )  B_SPLINE_SURFACE ( 3, 2, ( 
 ( #2020, #37546, #24796, #2446, #12011, #34358, #8400, #5638, #17984, #25003, #18191, #15430, #28178, #40947, #37965, #31579, #15004, #12220, #22012, #28383, #21587, #27761, #27968, #25208, #37759, #8614, #34561, #5422, #11388, #41164, #8826, #9032, #21170, #41371, #34985, #5849, #1613, #14592, #27565, #24374, #19449, #31999, #3484, #26259, #32618, #35186, #22847, #6267, #25839, #6052, #9458, #15639, #32214, #13065, #16070, #28596, #38804, #28801, #38386, #25632, #22425, #9891, #12653, #16474, #42008, #35816, #22219, #35402, #22640, #31779, #6678, #38593, #2651, #19030, #2865, #10087, #15855, #26047, #3078, #41799, #25422, #32416, #9248, #36020, #41583, #29423, #39010, #23051, #19241, #12437, #29012, #12859, #9677, #35616, #6479, #3283, #16269, #29210, #85, #19649, #294, #13276, #39207, #18819, #10928, #4543, #23699, #1150, #32825, #40274, #14329, #30277, #39415, #20716, #3694, #27308, #938, #16888, #503, #33692, #26885, #36229, #14118, #23912, #4115, #36880, #17522, #10292, #30487, #17316, #11143, #7102, #27093, #7741, #10712, #7528, #24126, #39852, #17099, #30062, #40060, #20499, #33468, #16682, #1356, #4331, #6883, #7313, #13690, #36663, #26460, #718, #29852, #39632, #20284, #33250, #29639, #19858, #13475, #23261, #26671, #13904, #20077, #33040, #3906, #10506, #23487, #36450, #40484, #30698, #7951, #17728, #33891, #1567, #37095, #14545, #27518, #20917, #11339, #4750, #35659, #41627, #38431, #35028, #6522, #5890, #29055, #19490, #28845, #28640, #16313, #18863, #25467, #19283, #32459, #9294, #31824, #26091, #25882, #337, #10128, #38636, #22260, #42051, #19072, #41844, #15901, #32662, #38844, #3325, #29253, #9503, #35446, #12482, #3525, #16113, #12696, #6720, #127, #3122, #13106, #22890, #25676, #16519, #26302, #35856, #9721, #32042, #22465, #29468, #12903, #35233, #6306, #22683, #15682, #39049, #9933, #13317, #6094, #19692, #32256, #39247, #2695, #2910, #10753, #23738, #36703, #36276, #7785, #30528, #36921, #39464, #27133, #10550, #30105, #10338, #13739, #19906, #36492, #17356, #20327, #32873, #981, #33082, #548, #29895, #26716, #14157, #16929, #20760, #4159, #40101, #26506, #39681, #26928, #36063, #10969, #764, #6931, #23314, #7149, #14370, #20119, #30318, #7354, #3948, #29683, #7566, #13519, #40317, #3736, #33731, #1187, #27345, #20540, #33293, #23095, #23532, #4584, #17142, #13951, #39892, #33514, #4378, #23955, #17563, #1396, #16722, #15206, #18607, #28171, #17977, #24166, #7987, #8393, #4996, #37136, #18184, #2227, #21372, #11580, #11793, #31570, #14790, #41157, #14585, #27558, #11383, #12004, #14995, #2013 ),
 ( #1605, #37538, #24789, #1810, #30953, #24995, #40525, #34554, #27754, #37958, #37751, #34350, #5415, #8819, #40723, #34762, #2439, #21789, #27960, #37336, #24573, #5629, #5209, #24365, #31153, #40937, #33931, #8608, #21580, #15423, #30741, #28376, #18393, #11183, #20960, #31361, #4791, #17769, #8188, #21163, #34135, #6668, #13054, #15631, #3271, #28789, #6256, #28587, #31990, #38163, #12640, #35606, #38581, #9025, #19231, #9240, #18811, #6044, #2855, #32407, #35178, #26037, #22414, #16258, #2643, #15845, #3067, #12213, #29197, #19021, #25203, #41574, #12428, #32609, #25413, #6469, #25622, #38375, #5840, #12846, #31771, #16463, #22001, #39000, #19437, #3472, #38794, #9446, #41363, #41788, #9882, #22209, #35391, #32203, #16060, #29000, #41998, #25830, #75, #22837, #35805, #19635, #34977, #9666, #22630, #26249, #26660, #23251, #13266, #36440, #20492, #39621, #29841, #30053, #36872, #33030, #17305, #32813, #3684, #29629, #33460, #33241, #20275, #6875, #1140, #40051, #708, #39405, #10492, #14111, #10706, #7732, #7303, #23477, #4105, #39844, #927, #13894, #39197, #27084, #26874, #4323, #13680, #36216, #17089, #19846, #7090, #10280, #20068, #23690, #36655, #10074, #7518, #23040, #10921, #3896, #30269, #23904, #36008, #16670, #494, #13463, #26449, #20706, #33683, #16877, #4533, #29413, #282, #17513, #27508, #40476, #27301, #17720, #30690, #18136, #24116, #20909, #30478, #31106, #1348, #11531, #1960, #11331, #11135, #40885, #14321, #7942, #1764, #14943, #33881, #40265, #8558, #8346, #24947, #35285, #21118, #4742, #24523, #1557, #24317, #37286, #15155, #21325, #27912, #11741, #34089, #17928, #37087, #28119, #40672, #14536, #8141, #4947, #37491, #30904, #14745, #27702, #34298, #5162, #24736, #37701, #21535, #34503, #5361, #41104, #18339, #31311, #11953, #2171, #38482, #9345, #22310, #13578, #29528, #38688, #19966, #32093, #26562, #181, #16163, #41896, #32931, #26149, #35501, #13370, #23150, #3381, #36118, #3796, #9559, #16781, #16574, #39519, #6359, #395, #6990, #9980, #6776, #22942, #25725, #42102, #29103, #38899, #6574, #19539, #2961, #35910, #28900, #29739, #12955, #13161, #39303, #12745, #22516, #19334, #32306, #3175, #603, #19749, #25935, #29309, #9778, #32716, #6148, #22736, #35712, #15951, #32510, #16366, #3579, #39099, #26352, #19128, #10183, #10398, #23373, #20297, #516, #307, #30078, #32633, #39219, #33053, #33265, #23065, #3497, #39863, #39648, #14130, #23925, #10305, #36033, #733, #32838, #13488, #29651, #4348, #10519, #4129, #952, #23277, #7115, #13288, #17328, #29866, #10101, #19661, #3706, #13707, #36243 ),
 ( #6899, #10725, #20089, #26686, #19872, #39430, #16487, #3919, #13918, #16900, #29438, #23500, #16695, #26273, #26474, #36463, #23712, #7327, #20513, #17114, #36675, #26897, #7539, #33484, #30291, #1162, #27106, #40074, #10941, #6692, #28144, #7964, #1987, #8164, #33904, #1369, #8371, #14344, #11978, #20730, #8583, #14969, #41132, #34323, #21140, #36894, #14559, #37312, #30499, #5388, #17952, #27323, #7757, #4763, #30929, #24341, #40287, #34113, #40498, #37111, #11158, #20933, #17743, #30716, #24141, #18367, #4558, #40908, #34530, #11555, #31130, #33706, #17534, #2199, #18161, #1581, #21556, #27533, #15179, #1786, #11356, #4971, #31337, #14768, #27729, #27936, #11766, #40698, #24763, #24547, #37514, #21351, #5186, #37727, #12188, #6229, #25804, #28763, #25597, #32385, #2831, #35156, #6020, #35367, #38557, #9424, #21764, #22602, #22390, #41973, #25390, #31749, #41761, #2413, #18789, #34947, #15603, #38349, #9213, #8795, #12615, #5603, #35579, #5816, #18996, #16035, #31544, #15401, #28353, #41338, #25180, #6443, #19205, #38139, #31961, #2619, #32178, #24971, #28561, #41550, #34737, #8998, #21974, #3041, #12402, #22187, #37932, #28974, #18579, #15818, #12821, #38770, #9639, #19413, #3247, #16234, #29175, #52, #29389, #9858, #4082, #3876, #20469, #30246, #16647, #258, #7065, #39174, #19822, #35983, #10685, #16855, #10472, #36417, #29605, #16439, #10053, #23017, #26224, #13242, #23668, #22815, #17063, #36631, #29819, #7283, #38978, #4299, #33434, #20253, #3449, #26852, #35784, #17281, #20045, #6851, #6646, #39821, #33008, #32789, #33216, #30031, #10258, #901, #7493, #3659, #13034, #23453, #26013, #469, #13872, #19610, #682, #13655, #32584, #26636, #23225, #36193, #13442, #39597, #26425, #39382, #40858, #27679, #18112, #1532, #7919, #4922, #20682, #37064, #11110, #33858, #14510, #27482, #27064, #30877, #23880, #11713, #24093, #37262, #34272, #7706, #33659, #4512, #17494, #30455, #24710, #17903, #1326, #24290, #20887, #1740, #1118, #4719, #17698, #10898, #14299, #27277, #14720, #40239, #30667, #14090, #40648, #40027, #8116, #11506, #40451, #36848, #24499, #11307, #21093, #34067, #37468, #8323, #21302, #5133, #31082, #8531, #18310, #1935, #14915, #27883, #37672, #21505, #34477, #5335, #22134, #28712, #12560, #34894, #31700, #24918, #377, #12347, #21710, #2143, #28301, #25333, #18738, #34685, #28506, #5762, #31493, #2568, #2360, #5551, #15352, #41284, #12128, #18525, #13353, #41075, #35315, #29507, #5967, #25547, #15130, #23131, #39282, #38508, #25123, #2987, #28092, #10163, #38291, #38088, #37877, #15979, #9157, #8944, #9373 ),
 ( #36098, #21916, #22338, #15551, #41497, #8736, #2777, #35106, #6970, #11925, #26335, #6179, #31283, #41706, #18941, #31908, #15760, #19153, #32124, #33330, #20159, #33120, #13989, #7392, #3984, #27171, #17599, #23991, #27379, #36960, #26756, #32910, #16760, #17182, #13776, #3774, #26964, #11004, #30142, #20365, #20578, #40352, #23571, #7822, #23352, #36314, #16966, #20794, #23774, #10790, #39501, #33765, #30564, #4198, #29932, #1020, #4619, #1225, #10590, #39720, #1430, #7187, #14195, #36527, #14404, #33554, #39928, #40137, #11216, #36739, #24200, #37167, #19944, #7601, #804, #4415, #29721, #17392, #30354, #584, #13556, #26544, #10375, #5447, #2469, #27587, #8848, #37571, #25025, #37986, #40971, #34167, #14820, #15453, #2044, #37366, #24605, #24821, #30773, #15027, #18424, #28408, #40556, #21823, #8424, #34795, #5661, #31184, #37780, #8637, #21609, #21197, #18639, #41397, #31604, #24397, #12033, #21403, #27992, #8220, #40757, #4824, #34380, #2259, #5240, #17800, #11824, #18007, #11410, #27787, #11614, #41188, #1840, #12245, #34583, #25229, #5027, #18215, #31392, #20993, #8019, #15242, #33964, #30984, #28202, #1634, #14617, #3302, #9482, #35211, #2677, #9701, #15663, #13296, #22034, #9912, #16290, #29445, #35638, #22445, #38194, #15879, #22869, #22239, #35425, #38408, #9273, #32233, #25654, #6073, #29229, #35837, #106, #3503, #13086, #2888, #9058, #35009, #6287, #32022, #5871, #3103, #26070, #19261, #38615, #38824, #16496, #41824, #39027, #41607, #12463, #19052, #6699, #42030, #29033, #28619, #19668, #32640, #16094, #28824, #12882, #316, #19471, #12675, #25860, #18843, #25447, #32439, #22662, #31802, #6502, #36470, #20518, #14136, #16906, #7763, #17539, #27111, #29873, #20096, #17334, #29657, #7545, #33059, #40080, #39870, #7333, #33492, #10946, #741, #20736, #30505, #23931, #17121, #10312, #3925, #33712, #20303, #13494, #13713, #958, #6906, #33272, #23717, #4562, #3712, #36900, #26692, #1167, #1373, #4136, #13925, #26905, #10732, #39439, #26278, #39226, #10108, #523, #30296, #39654, #30085, #26483, #10525, #23072, #23508, #4353, #36680, #36038, #19880, #36250, #16700, #32847, #23285, #7123, #8167, #28147, #37517, #18371, #17749, #17955, #18165, #27327, #5393, #21143, #40293, #30720, #1585, #5610, #27539, #21560, #27733, #11361, #20937, #27941, #33908, #31547, #11162, #41135, #34533, #18584, #11771, #40702, #14349, #34116, #11982, #40504, #11559, #14563, #24346, #8375, #1790, #37315, #31342, #24974, #2203, #21769, #15184, #4975, #24147, #37116, #24552, #30933, #7968, #21355, #37935, #34328, #14772, #14975, #34741, #5190 ),
 ( #4768, #31135, #40913, #1991, #24767, #37730, #8587, #8797, #41341, #41764, #38354, #28356, #9427, #35583, #12621, #2835, #3046, #9862, #6023, #32388, #5819, #18792, #2622, #6446, #6234, #35371, #21981, #16237, #13038, #15822, #12407, #25600, #29178, #25808, #35159, #9217, #19418, #31752, #38774, #22190, #56, #16038, #38560, #9644, #3254, #18999, #26016, #35789, #38982, #19209, #28565, #31965, #22818, #22393, #15607, #28769, #32181, #25184, #28979, #41976, #6651, #34950, #19616, #12824, #2416, #15404, #22605, #12191, #38145, #9002, #41553, #25393, #40032, #4303, #6855, #36635, #20049, #39601, #19827, #23230, #29393, #3880, #26856, #29823, #264, #10476, #475, #10060, #39386, #36197, #23672, #26432, #17287, #13660, #7498, #35989, #7070, #36422, #3454, #20474, #10264, #16444, #32793, #3665, #23885, #16651, #39826, #16860, #29609, #39178, #4086, #23021, #7712, #13246, #30250, #10689, #36852, #30035, #690, #32588, #33012, #1122, #13446, #26643, #23457, #7287, #20257, #33222, #17070, #33442, #14093, #27067, #10901, #26229, #906, #13877, #11717, #11511, #28097, #37882, #24297, #7924, #14725, #4722, #27487, #1535, #18315, #24504, #18116, #1940, #37267, #21097, #14301, #31288, #1743, #11113, #33664, #17701, #27682, #8120, #24098, #17906, #34070, #20890, #37067, #30670, #14515, #33863, #40456, #2147, #30459, #24716, #15134, #37471, #14922, #4515, #11930, #41082, #27889, #11310, #34482, #17497, #24924, #40654, #4925, #27280, #5341, #8327, #30883, #40863, #37678, #21304, #8535, #20686, #34276, #1330, #31087, #40243, #5138, #21512, #9593, #12566, #9377, #16192, #28718, #18949, #31913, #19158, #22342, #35320, #5556, #6391, #6183, #25757, #9164, #15557, #25551, #28305, #2572, #18742, #41502, #22139, #35110, #34689, #38512, #31498, #19368, #31704, #2783, #41927, #15356, #41289, #12135, #25129, #38094, #32339, #32128, #8949, #15765, #28513, #2993, #8741, #12354, #25338, #18530, #21923, #34899, #15987, #5768, #38298, #21717, #28930, #2366, #41711, #12775, #5972, #38724, #22552, #35532, #3206, #29133, #8, #12989, #25970, #10214, #6807, #19999, #10644, #20210, #29562, #32746, #29982, #211, #33171, #3614, #23621, #10428, #7020, #4038, #26810, #424, #20424, #30198, #39776, #29772, #22971, #16605, #33388, #32964, #26180, #13399, #13608, #19568, #3830, #36372, #4254, #16398, #36580, #26382, #13829, #7448, #16809, #26593, #39551, #23406, #10011, #17238, #1076, #14048, #13192, #857, #39332, #635, #39129, #23183, #35743, #36148, #17021, #7240, #6603, #38932, #19780, #29342, #9809, #22767, #32540, #3407, #35941, #27435, #11462, #4472 ),
 ( #37217, #34026, #1892, #24247, #14463, #40404, #30829, #4878, #17857, #10848, #5086, #1691, #24454, #17654, #24047, #8072, #20634, #37016, #40194, #20844, #4674, #30619, #39983, #21048, #36801, #34225, #11064, #11265, #37423, #7663, #33612, #17453, #30411, #1282, #18066, #14675, #14252, #27634, #7877, #40606, #27020, #33818, #1485, #27230, #8281, #21256, #31038, #14874, #27842, #40818, #23835, #4179, #29702, #36719, #36509, #33098, #17162, #10771, #13536, #4396, #14174, #23755, #13758, #6949, #565, #17374, #16946, #10145, #39482, #39697, #3542, #29913, #20345, #30334, #356, #7584, #10356, #39909, #20559, #3965, #10570, #23550, #7371, #36080, #33534, #1207, #27151, #39264, #26947, #23332, #784, #23112, #26523, #19711, #36293, #30124, #20138, #32680, #26737, #32890, #13335, #7167, #33311, #13968, #16739, #40117, #1000, #22909, #26317, #35873, #6738, #16536, #29486, #19924, #3754, #27364, #40337, #2243, #24183, #18200, #24381, #8005, #17580, #24591, #30545, #28185, #36940, #24804, #31168, #15223, #8409, #37350, #10986, #30757, #37766, #37153, #8204, #11199, #20975, #5011, #40540, #33949, #2029, #8621, #15011, #18408, #27975, #17785, #23974, #7802, #21177, #4807, #20777, #17992, #40956, #34153, #11396, #11596, #31378, #14599, #11808, #14387, #1620, #27573, #21594, #14805, #1826, #1413, #34568, #5431, #30969, #27770, #40741, #33747, #34366, #37556, #21386, #5224, #4601, #9466, #32423, #28393, #35410, #42015, #2873, #41807, #6486, #19039, #9256, #22226, #19249, #12661, #25640, #37972, #9685, #38601, #16078, #41591, #5857, #15864, #18622, #34993, #9043, #31788, #12448, #25431, #25010, #28810, #21807, #22648, #22020, #35194, #32220, #5647, #31586, #2453, #15439, #41379, #35623, #3086, #12229, #6060, #18827, #29019, #41172, #2660, #15647, #8832, #25216, #38178, #12866, #28604, #38394, #12018, #25847, #34777, #32007, #19456, #3289, #16275, #10512, #13071, #19655, #13481, #725, #3490, #26056, #20290, #20083, #36670, #4339, #32831, #16480, #23268, #13282, #36027, #10094, #26891, #33047, #26677, #23493, #3700, #29645, #22853, #39858, #10298, #32626, #91, #26265, #36235, #16689, #29431, #26467, #509, #301, #39213, #23058, #6890, #19864, #39423, #10719, #39015, #33256, #23706, #3912, #36456, #9897, #20506, #7534, #7320, #7108, #944, #35823, #33476, #16893, #29859, #6685, #13911, #13697, #39639, #4122, #17106, #30069, #29217, #31688, #31272, #27872, #41061, #2557, #41274, #8518, #11701, #8934, #21292, #12118, #24699, #15540, #31482, #28080, #25112, #5751, #21495, #41487, #9147, #18728, #8724, #1924, #37661, #12335, #11913, #5122 ),
 ( #34261, #15119, #34466, #18101, #31071, #14903, #40848, #5326, #18300, #28493, #27668, #21905, #25321, #34673, #38075, #1728, #22123, #38281, #34884, #8312, #35095, #14709, #17893, #24907, #2135, #11495, #30866, #37866, #21696, #40638, #24488, #5539, #37457, #18513, #2349, #15336, #28290, #39321, #35305, #29329, #6793, #9796, #6591, #13389, #38919, #16180, #29119, #16385, #19556, #32528, #2765, #3600, #3396, #22960, #6379, #12762, #22754, #25535, #41914, #15969, #38708, #19351, #32326, #31897, #35729, #28702, #16593, #28917, #24153, #39118, #12549, #38499, #9362, #22328, #6168, #29548, #198, #19145, #12974, #25743, #13180, #5956, #9578, #22536, #15750, #32113, #2978, #26166, #35520, #3193, #18930, #9997, #41696, #35929, #19767, #32734, #413, #26369, #10201, #23170, #29970, #7867, #17226, #40181, #39538, #39762, #39970, #7009, #27218, #844, #19986, #10417, #23394, #27426, #7227, #1271, #7435, #33159, #620, #7647, #13596, #11255, #32950, #20835, #14239, #40394, #33601, #20410, #36135, #13817, #33807, #20199, #33375, #36357, #4024, #1061, #23609, #17007, #11051, #4662, #24034, #1475, #37005, #26799, #3817, #16797, #4242, #10631, #29759, #14036, #17643, #27008, #36570, #36787, #14450, #10836, #30607, #23821, #20622, #4460, #26581, #17441, #30399, #1680, #38030, #34839, #37615, #34214, #5283, #8894, #5493, #14864, #18054, #15291, #27626, #18468, #31028, #21865, #37822, #34424, #31435, #12074, #27831, #5708, #15499, #25068, #15073, #8268, #1881, #18683, #18257, #11452, #40803, #41018, #4865, #31228, #21651, #31646, #14664, #2511, #11656, #41232, #28452, #2089, #11869, #24863, #8678, #37410, #41440, #24238, #37207, #40596, #28245, #24654, #28036, #24443, #8472, #21036, #21449, #2303, #34628, #34013, #8062, #17845, #30818, #21242, #5074, #41653, #6334, #38456, #19099, #35258, #9960, #3151, #9749, #35689, #15925, #12722, #5917, #22920, #35474, #2722, #25273, #9319, #19308, #41871, #15707, #9532, #28874, #12510, #28660, #22286, #6121, #25494, #32066, #35885, #22083, #16340, #6749, #29078, #19518, #38242, #3553, #19723, #32487, #2936, #26119, #9103, #32691, #32284, #25700, #31854, #39078, #16141, #38664, #3353, #29283, #22492, #154, #16547, #42075, #29498, #22710, #12290, #12931, #13136, #35052, #25907, #38874, #7812, #20356, #10582, #23560, #10781, #1011, #13979, #39275, #40128, #26957, #17384, #796, #7178, #4190, #19936, #36305, #10367, #33110, #13769, #26748, #26328, #30134, #23123, #10996, #23342, #36519, #33545, #6960, #32901, #3766, #16750, #29713, #23983, #17173, #575, #7381, #20150, #39919, #368, #3975, #16957, #10156 ) ),
 .UNSPECIFIED., .T., .F., .T. ) 
 B_SPLINE_SURFACE_WITH_KNOTS ( ( 4, 3, 4 ),
 ( 3, 2, 2, 2, 2, 2, 2, 2, 2, 2, 2, 2, 2, 2, 2, 2, 2, 2, 2, 2, 2, 2, 2, 2, 2, 2, 2, 2, 2, 2, 2, 2, 2, 2, 2, 2, 2, 2, 2, 2, 2, 2, 2, 2, 2, 2, 2, 2, 2, 2, 2, 2, 2, 2, 2, 2, 2, 2, 2, 2, 2, 2, 2, 2, 2, 2, 2, 2, 2, 2, 2, 2, 2, 2, 2, 2, 2, 2, 2, 2, 2, 2, 2, 2, 2, 2, 2, 2, 2, 2, 2, 2, 2, 2, 2, 2, 2, 2, 2, 2, 2, 2, 2, 2, 2, 2, 2, 2, 2, 2, 2, 2, 2, 2, 2, 2, 2, 2, 2, 2, 2, 2, 2, 2, 2, 2, 2, 2, 2, 2, 2, 2, 2, 2, 2, 2, 2, 2, 2, 2, 2, 2, 2, 2, 2, 2, 2, 2, 2, 2, 2, 2, 2, 2, 2, 2, 2, 2, 2, 2, 2, 2, 2, 2, 2, 3 ),
 ( 0.000000000000000000, 0.5000000000000000000, 1.000000000000000000 ),
 ( 0.000000000000000000, 0.005882352941176470507, 0.01176470588235294101, 0.01764705882352941152, 0.02352941176470588203, 0.02941176470588235253, 0.03529411764705882304, 0.04117647058823529355, 0.04705882352941176405, 0.05294117647058823456, 0.05882352941176470507, 0.06470588235294118251, 0.07058823529411764608, 0.07647058823529412352, 0.08235294117647058709, 0.08823529411764706454, 0.09411764705882352811, 0.1000000000000000056, 0.1058823529411764691, 0.1117647058823529466, 0.1176470588235294101, 0.1235294117647058876, 0.1294117647058823650, 0.1352941176470588147, 0.1411764705882352922, 0.1470588235294117696, 0.1529411764705882470, 0.1588235294117646967, 0.1647058823529411742, 0.1705882352941176516, 0.1764705882352941291, 0.1823529411764705788, 0.1882352941176470562, 0.1941176470588235337, 0.2000000000000000111, 0.2058823529411764608, 0.2117647058823529382, 0.2176470588235294157, 0.2235294117647058931, 0.2294117647058823428, 0.2352941176470588203, 0.2411764705882352977, 0.2470588235294117752, 0.2529411764705882248, 0.2588235294117647300, 0.2647058823529411797, 0.2705882352941176294, 0.2764705882352941346, 0.2823529411764705843, 0.2882352941176470340, 0.2941176470588235392, 0.2999999999999999889, 0.3058823529411764941, 0.3117647058823529438, 0.3176470588235293935, 0.3235294117647058987, 0.3294117647058823484, 0.3352941176470587981, 0.3411764705882353033, 0.3470588235294117530, 0.3529411764705882582, 0.3588235294117647078, 0.3647058823529411575, 0.3705882352941176627, 0.3764705882352941124, 0.3823529411764705621, 0.3882352941176470673, 0.3941176470588235170, 0.4000000000000000222, 0.4058823529411764719, 0.4117647058823529216, 0.4176470588235294268, 0.4235294117647058765, 0.4294117647058823262, 0.4352941176470588314, 0.4411764705882352811, 0.4470588235294117863, 0.4529411764705882359, 0.4588235294117646856, 0.4647058823529411908, 0.4705882352941176405, 0.4764705882352940902, 0.4823529411764705954, 0.4882352941176470451, 0.4941176470588235503, 0.5000000000000000000, 0.5058823529411764497, 0.5117647058823528994, 0.5176470588235294601, 0.5235294117647059098, 0.5294117647058823595, 0.5352941176470588092, 0.5411764705882352589, 0.5470588235294118196, 0.5529411764705882693, 0.5588235294117647189, 0.5647058823529411686, 0.5705882352941176183, 0.5764705882352940680, 0.5823529411764706287, 0.5882352941176470784, 0.5941176470588235281, 0.5999999999999999778, 0.6058823529411764275, 0.6117647058823529882, 0.6176470588235294379, 0.6235294117647058876, 0.6294117647058823373, 0.6352941176470587870, 0.6411764705882353477, 0.6470588235294117974, 0.6529411764705882470, 0.6588235294117646967, 0.6647058823529411464, 0.6705882352941175961, 0.6764705882352941568, 0.6823529411764706065, 0.6882352941176470562, 0.6941176470588235059, 0.6999999999999999556, 0.7058823529411765163, 0.7117647058823529660, 0.7176470588235294157, 0.7235294117647058654, 0.7294117647058823151, 0.7352941176470588758, 0.7411764705882353255, 0.7470588235294117752, 0.7529411764705882248, 0.7588235294117646745, 0.7647058823529411242, 0.7705882352941176849, 0.7764705882352941346, 0.7823529411764705843, 0.7882352941176470340, 0.7941176470588234837, 0.8000000000000000444, 0.8058823529411764941, 0.8117647058823529438, 0.8176470588235293935, 0.8235294117647058432, 0.8294117647058824039, 0.8352941176470588536, 0.8411764705882353033, 0.8470588235294117530, 0.8529411764705882026, 0.8588235294117646523, 0.8647058823529412130, 0.8705882352941176627, 0.8764705882352941124, 0.8823529411764705621, 0.8882352941176470118, 0.8941176470588235725, 0.9000000000000000222, 0.9058823529411764719, 0.9117647058823529216, 0.9176470588235293713, 0.9235294117647059320, 0.9294117647058823817, 0.9352941176470588314, 0.9411764705882352811, 0.9470588235294117307, 0.9529411764705881804, 0.9588235294117647411, 0.9647058823529411908, 0.9705882352941176405 ),
 .UNSPECIFIED. ) 
 GEOMETRIC_REPRESENTATION_ITEM ( )  RATIONAL_B_SPLINE_SURFACE ( (
 ( 1.000000000000000000, 0.9510565162951535312, 1.000000000000000000, 0.9510565162951535312, 1.000000000000000000, 0.9510565162951535312, 1.000000000000000000, 0.9510565162951535312, 1.000000000000000000, 0.9510565162951535312, 1.000000000000000000, 0.9510565162951535312, 1.000000000000000000, 0.9510565162951535312, 1.000000000000000000, 0.9510565162951535312, 1.000000000000000000, 0.9510565162951535312, 1.000000000000000000, 0.9510565162951535312, 1.000000000000000000, 0.9510565162951535312, 1.000000000000000000, 0.9510565162951535312, 1.000000000000000000, 0.9510565162951535312, 1.000000000000000000, 0.9510565162951535312, 1.000000000000000000, 0.9510565162951535312, 1.000000000000000000, 0.9510565162951535312, 1.000000000000000000, 0.9510565162951535312, 1.000000000000000000, 0.9510565162951535312, 1.000000000000000000, 0.9510565162951535312, 1.000000000000000000, 0.9510565162951535312, 1.000000000000000000, 0.9510565162951535312, 1.000000000000000000, 0.9510565162951535312, 1.000000000000000000, 0.9510565162951535312, 1.000000000000000000, 0.9510565162951535312, 1.000000000000000000, 0.9510565162951535312, 1.000000000000000000, 0.9510565162951535312, 1.000000000000000000, 0.9510565162951535312, 1.000000000000000000, 0.9510565162951535312, 1.000000000000000000, 0.9510565162951535312, 1.000000000000000000, 0.9510565162951535312, 1.000000000000000000, 0.9510565162951535312, 1.000000000000000000, 0.9510565162951535312, 1.000000000000000000, 0.9510565162951535312, 1.000000000000000000, 0.9510565162951535312, 1.000000000000000000, 0.9510565162951535312, 1.000000000000000000, 0.9510565162951535312, 1.000000000000000000, 0.9510565162951535312, 1.000000000000000000, 0.9510565162951535312, 1.000000000000000000, 0.9510565162951535312, 1.000000000000000000, 0.9510565162951535312, 1.000000000000000000, 0.9510565162951535312, 1.000000000000000000, 0.9510565162951535312, 1.000000000000000000, 0.9510565162951535312, 1.000000000000000000, 0.9510565162951535312, 1.000000000000000000, 0.9510565162951535312, 1.000000000000000000, 0.9510565162951535312, 1.000000000000000000, 0.9510565162951535312, 1.000000000000000000, 0.9510565162951535312, 1.000000000000000000, 0.9510565162951535312, 1.000000000000000000, 0.9510565162951535312, 1.000000000000000000, 0.9510565162951535312, 1.000000000000000000, 0.9510565162951535312, 1.000000000000000000, 0.9510565162951535312, 1.000000000000000000, 0.9510565162951535312, 1.000000000000000000, 0.9510565162951535312, 1.000000000000000000, 0.9510565162951535312, 1.000000000000000000, 0.9510565162951535312, 1.000000000000000000, 0.9510565162951535312, 1.000000000000000000, 0.9510565162951535312, 1.000000000000000000, 0.9510565162951535312, 1.000000000000000000, 0.9510565162951535312, 1.000000000000000000, 0.9510565162951535312, 1.000000000000000000, 0.9510565162951535312, 1.000000000000000000, 0.9510565162951535312, 1.000000000000000000, 0.9510565162951535312, 1.000000000000000000, 0.9510565162951535312, 1.000000000000000000, 0.9510565162951535312, 1.000000000000000000, 0.9510565162951535312, 1.000000000000000000, 0.9510565162951535312, 1.000000000000000000, 0.9510565162951535312, 1.000000000000000000, 0.9510565162951535312, 1.000000000000000000, 0.9510565162951535312, 1.000000000000000000, 0.9510565162951535312, 1.000000000000000000, 0.9510565162951535312, 1.000000000000000000, 0.9510565162951535312, 1.000000000000000000, 0.9510565162951535312, 1.000000000000000000, 0.9510565162951535312, 1.000000000000000000, 0.9510565162951535312, 1.000000000000000000, 0.9510565162951535312, 1.000000000000000000, 0.9510565162951535312, 1.000000000000000000, 0.9510565162951535312, 1.000000000000000000, 0.9510565162951535312, 1.000000000000000000, 0.9510565162951535312, 1.000000000000000000, 0.9510565162951535312, 1.000000000000000000, 0.9510565162951535312, 1.000000000000000000, 0.9510565162951535312, 1.000000000000000000, 0.9510565162951535312, 1.000000000000000000, 0.9510565162951535312, 1.000000000000000000, 0.9510565162951535312, 1.000000000000000000, 0.9510565162951535312, 1.000000000000000000, 0.9510565162951535312, 1.000000000000000000, 0.9510565162951535312, 1.000000000000000000, 0.9510565162951535312, 1.000000000000000000, 0.9510565162951535312, 1.000000000000000000, 0.9510565162951535312, 1.000000000000000000, 0.9510565162951535312, 1.000000000000000000, 0.9510565162951535312, 1.000000000000000000, 0.9510565162951535312, 1.000000000000000000, 0.9510565162951535312, 1.000000000000000000, 0.9510565162951535312, 1.000000000000000000, 0.9510565162951535312, 1.000000000000000000, 0.9510565162951535312, 1.000000000000000000, 0.9510565162951535312, 1.000000000000000000, 0.9510565162951535312, 1.000000000000000000, 0.9510565162951535312, 1.000000000000000000, 0.9510565162951535312, 1.000000000000000000, 0.9510565162951535312, 1.000000000000000000, 0.9510565162951535312, 1.000000000000000000, 0.9510565162951535312, 1.000000000000000000, 0.9510565162951535312, 1.000000000000000000, 0.9510565162951535312, 1.000000000000000000, 0.9510565162951535312, 1.000000000000000000, 0.9510565162951535312, 1.000000000000000000, 0.9510565162951535312, 1.000000000000000000, 0.9510565162951535312, 1.000000000000000000, 0.9510565162951535312, 1.000000000000000000, 0.9510565162951535312, 1.000000000000000000, 0.9510565162951535312, 1.000000000000000000, 0.9510565162951535312, 1.000000000000000000, 0.9510565162951535312, 1.000000000000000000, 0.9510565162951535312, 1.000000000000000000, 0.9510565162951535312, 1.000000000000000000, 0.9510565162951535312, 1.000000000000000000, 0.9510565162951535312, 1.000000000000000000, 0.9510565162951535312, 1.000000000000000000, 0.9510565162951535312, 1.000000000000000000, 0.9510565162951535312, 1.000000000000000000, 0.9510565162951535312, 1.000000000000000000, 0.9510565162951535312, 1.000000000000000000, 0.9510565162951535312, 1.000000000000000000, 0.9510565162951535312, 1.000000000000000000, 0.9510565162951535312, 1.000000000000000000, 0.9510565162951535312, 1.000000000000000000, 0.9510565162951535312, 1.000000000000000000, 0.9510565162951535312, 1.000000000000000000, 0.9510565162951535312, 1.000000000000000000, 0.9510565162951535312, 1.000000000000000000, 0.9510565162951535312, 1.000000000000000000, 0.9510565162951535312, 1.000000000000000000, 0.9510565162951535312, 1.000000000000000000, 0.9510565162951535312, 1.000000000000000000, 0.9510565162951535312, 1.000000000000000000, 0.9510565162951535312, 1.000000000000000000, 0.9510565162951535312, 1.000000000000000000, 0.9510565162951535312, 1.000000000000000000, 0.9510565162951535312, 1.000000000000000000, 0.9510565162951535312, 1.000000000000000000, 0.9510565162951535312, 1.000000000000000000, 0.9510565162951535312, 1.000000000000000000, 0.9510565162951535312, 1.000000000000000000, 0.9510565162951535312, 1.000000000000000000, 0.9510565162951535312, 1.000000000000000000, 0.9510565162951535312, 1.000000000000000000, 0.9510565162951535312, 1.000000000000000000, 0.9510565162951535312, 1.000000000000000000, 0.9510565162951535312, 1.000000000000000000, 0.9510565162951535312, 1.000000000000000000, 0.9510565162951535312, 1.000000000000000000, 0.9510565162951535312, 1.000000000000000000, 0.9510565162951535312, 1.000000000000000000, 0.9510565162951535312, 1.000000000000000000, 0.9510565162951535312, 1.000000000000000000, 0.9510565162951535312, 1.000000000000000000, 0.9510565162951535312, 1.000000000000000000, 0.9510565162951535312, 1.000000000000000000),
 ( 0.3333333333333333703, 0.3170188387650512141, 0.3333333333333333703, 0.3170188387650512141, 0.3333333333333333703, 0.3170188387650512141, 0.3333333333333333703, 0.3170188387650512141, 0.3333333333333333703, 0.3170188387650512141, 0.3333333333333333703, 0.3170188387650512141, 0.3333333333333333703, 0.3170188387650512141, 0.3333333333333333703, 0.3170188387650512141, 0.3333333333333333703, 0.3170188387650512141, 0.3333333333333333703, 0.3170188387650512141, 0.3333333333333333703, 0.3170188387650512141, 0.3333333333333333703, 0.3170188387650512141, 0.3333333333333333703, 0.3170188387650512141, 0.3333333333333333703, 0.3170188387650512141, 0.3333333333333333703, 0.3170188387650512141, 0.3333333333333333703, 0.3170188387650512141, 0.3333333333333333703, 0.3170188387650512141, 0.3333333333333333703, 0.3170188387650512141, 0.3333333333333333703, 0.3170188387650512141, 0.3333333333333333703, 0.3170188387650512141, 0.3333333333333333703, 0.3170188387650512141, 0.3333333333333333703, 0.3170188387650512141, 0.3333333333333333703, 0.3170188387650512141, 0.3333333333333333703, 0.3170188387650512141, 0.3333333333333333703, 0.3170188387650512141, 0.3333333333333333703, 0.3170188387650512141, 0.3333333333333333703, 0.3170188387650512141, 0.3333333333333333703, 0.3170188387650512141, 0.3333333333333333703, 0.3170188387650512141, 0.3333333333333333703, 0.3170188387650512141, 0.3333333333333333703, 0.3170188387650512141, 0.3333333333333333703, 0.3170188387650512141, 0.3333333333333333703, 0.3170188387650512141, 0.3333333333333333703, 0.3170188387650512141, 0.3333333333333333703, 0.3170188387650512141, 0.3333333333333333703, 0.3170188387650512141, 0.3333333333333333703, 0.3170188387650512141, 0.3333333333333333703, 0.3170188387650512141, 0.3333333333333333703, 0.3170188387650512141, 0.3333333333333333703, 0.3170188387650512141, 0.3333333333333333703, 0.3170188387650512141, 0.3333333333333333703, 0.3170188387650512141, 0.3333333333333333703, 0.3170188387650512141, 0.3333333333333333703, 0.3170188387650512141, 0.3333333333333333703, 0.3170188387650512141, 0.3333333333333333703, 0.3170188387650512141, 0.3333333333333333703, 0.3170188387650512141, 0.3333333333333333703, 0.3170188387650512141, 0.3333333333333333703, 0.3170188387650512141, 0.3333333333333333703, 0.3170188387650512141, 0.3333333333333333703, 0.3170188387650512141, 0.3333333333333333703, 0.3170188387650512141, 0.3333333333333333703, 0.3170188387650512141, 0.3333333333333333703, 0.3170188387650512141, 0.3333333333333333703, 0.3170188387650512141, 0.3333333333333333703, 0.3170188387650512141, 0.3333333333333333703, 0.3170188387650512141, 0.3333333333333333703, 0.3170188387650512141, 0.3333333333333333703, 0.3170188387650512141, 0.3333333333333333703, 0.3170188387650512141, 0.3333333333333333703, 0.3170188387650512141, 0.3333333333333333703, 0.3170188387650512141, 0.3333333333333333703, 0.3170188387650512141, 0.3333333333333333703, 0.3170188387650512141, 0.3333333333333333703, 0.3170188387650512141, 0.3333333333333333703, 0.3170188387650512141, 0.3333333333333333703, 0.3170188387650512141, 0.3333333333333333703, 0.3170188387650512141, 0.3333333333333333703, 0.3170188387650512141, 0.3333333333333333703, 0.3170188387650512141, 0.3333333333333333703, 0.3170188387650512141, 0.3333333333333333703, 0.3170188387650512141, 0.3333333333333333703, 0.3170188387650512141, 0.3333333333333333703, 0.3170188387650512141, 0.3333333333333333703, 0.3170188387650512141, 0.3333333333333333703, 0.3170188387650512141, 0.3333333333333333703, 0.3170188387650512141, 0.3333333333333333703, 0.3170188387650512141, 0.3333333333333333703, 0.3170188387650512141, 0.3333333333333333703, 0.3170188387650512141, 0.3333333333333333703, 0.3170188387650512141, 0.3333333333333333703, 0.3170188387650512141, 0.3333333333333333703, 0.3170188387650512141, 0.3333333333333333703, 0.3170188387650512141, 0.3333333333333333703, 0.3170188387650512141, 0.3333333333333333703, 0.3170188387650512141, 0.3333333333333333703, 0.3170188387650512141, 0.3333333333333333703, 0.3170188387650512141, 0.3333333333333333703, 0.3170188387650512141, 0.3333333333333333703, 0.3170188387650512141, 0.3333333333333333703, 0.3170188387650512141, 0.3333333333333333703, 0.3170188387650512141, 0.3333333333333333703, 0.3170188387650512141, 0.3333333333333333703, 0.3170188387650512141, 0.3333333333333333703, 0.3170188387650512141, 0.3333333333333333703, 0.3170188387650512141, 0.3333333333333333703, 0.3170188387650512141, 0.3333333333333333703, 0.3170188387650512141, 0.3333333333333333703, 0.3170188387650512141, 0.3333333333333333703, 0.3170188387650512141, 0.3333333333333333703, 0.3170188387650512141, 0.3333333333333333703, 0.3170188387650512141, 0.3333333333333333703, 0.3170188387650512141, 0.3333333333333333703, 0.3170188387650512141, 0.3333333333333333703, 0.3170188387650512141, 0.3333333333333333703, 0.3170188387650512141, 0.3333333333333333703, 0.3170188387650512141, 0.3333333333333333703, 0.3170188387650512141, 0.3333333333333333703, 0.3170188387650512141, 0.3333333333333333703, 0.3170188387650512141, 0.3333333333333333703, 0.3170188387650512141, 0.3333333333333333703, 0.3170188387650512141, 0.3333333333333333703, 0.3170188387650512141, 0.3333333333333333703, 0.3170188387650512141, 0.3333333333333333703, 0.3170188387650512141, 0.3333333333333333703, 0.3170188387650512141, 0.3333333333333333703, 0.3170188387650512141, 0.3333333333333333703, 0.3170188387650512141, 0.3333333333333333703, 0.3170188387650512141, 0.3333333333333333703, 0.3170188387650512141, 0.3333333333333333703, 0.3170188387650512141, 0.3333333333333333703, 0.3170188387650512141, 0.3333333333333333703, 0.3170188387650512141, 0.3333333333333333703, 0.3170188387650512141, 0.3333333333333333703, 0.3170188387650512141, 0.3333333333333333703, 0.3170188387650512141, 0.3333333333333333703, 0.3170188387650512141, 0.3333333333333333703, 0.3170188387650512141, 0.3333333333333333703, 0.3170188387650512141, 0.3333333333333333703, 0.3170188387650512141, 0.3333333333333333703, 0.3170188387650512141, 0.3333333333333333703, 0.3170188387650512141, 0.3333333333333333703, 0.3170188387650512141, 0.3333333333333333703, 0.3170188387650512141, 0.3333333333333333703, 0.3170188387650512141, 0.3333333333333333703, 0.3170188387650512141, 0.3333333333333333703, 0.3170188387650512141, 0.3333333333333333703, 0.3170188387650512141, 0.3333333333333333703, 0.3170188387650512141, 0.3333333333333333703, 0.3170188387650512141, 0.3333333333333333703, 0.3170188387650512141, 0.3333333333333333703, 0.3170188387650512141, 0.3333333333333333703, 0.3170188387650512141, 0.3333333333333333703, 0.3170188387650512141, 0.3333333333333333703, 0.3170188387650512141, 0.3333333333333333703, 0.3170188387650512141, 0.3333333333333333703, 0.3170188387650512141, 0.3333333333333333703, 0.3170188387650512141, 0.3333333333333333703, 0.3170188387650512141, 0.3333333333333333703, 0.3170188387650512141, 0.3333333333333333703, 0.3170188387650512141, 0.3333333333333333703, 0.3170188387650512141, 0.3333333333333333703, 0.3170188387650512141, 0.3333333333333333703, 0.3170188387650512141, 0.3333333333333333703, 0.3170188387650512141, 0.3333333333333333703, 0.3170188387650512141, 0.3333333333333333703, 0.3170188387650512141, 0.3333333333333333703, 0.3170188387650512141, 0.3333333333333333703, 0.3170188387650512141, 0.3333333333333333703, 0.3170188387650512141, 0.3333333333333333703, 0.3170188387650512141, 0.3333333333333333703, 0.3170188387650512141, 0.3333333333333333703, 0.3170188387650512141, 0.3333333333333333703, 0.3170188387650512141, 0.3333333333333333703, 0.3170188387650512141, 0.3333333333333333703),
 ( 0.3333333333333333703, 0.3170188387650512141, 0.3333333333333333703, 0.3170188387650512141, 0.3333333333333333703, 0.3170188387650512141, 0.3333333333333333703, 0.3170188387650512141, 0.3333333333333333703, 0.3170188387650512141, 0.3333333333333333703, 0.3170188387650512141, 0.3333333333333333703, 0.3170188387650512141, 0.3333333333333333703, 0.3170188387650512141, 0.3333333333333333703, 0.3170188387650512141, 0.3333333333333333703, 0.3170188387650512141, 0.3333333333333333703, 0.3170188387650512141, 0.3333333333333333703, 0.3170188387650512141, 0.3333333333333333703, 0.3170188387650512141, 0.3333333333333333703, 0.3170188387650512141, 0.3333333333333333703, 0.3170188387650512141, 0.3333333333333333703, 0.3170188387650512141, 0.3333333333333333703, 0.3170188387650512141, 0.3333333333333333703, 0.3170188387650512141, 0.3333333333333333703, 0.3170188387650512141, 0.3333333333333333703, 0.3170188387650512141, 0.3333333333333333703, 0.3170188387650512141, 0.3333333333333333703, 0.3170188387650512141, 0.3333333333333333703, 0.3170188387650512141, 0.3333333333333333703, 0.3170188387650512141, 0.3333333333333333703, 0.3170188387650512141, 0.3333333333333333703, 0.3170188387650512141, 0.3333333333333333703, 0.3170188387650512141, 0.3333333333333333703, 0.3170188387650512141, 0.3333333333333333703, 0.3170188387650512141, 0.3333333333333333703, 0.3170188387650512141, 0.3333333333333333703, 0.3170188387650512141, 0.3333333333333333703, 0.3170188387650512141, 0.3333333333333333703, 0.3170188387650512141, 0.3333333333333333703, 0.3170188387650512141, 0.3333333333333333703, 0.3170188387650512141, 0.3333333333333333703, 0.3170188387650512141, 0.3333333333333333703, 0.3170188387650512141, 0.3333333333333333703, 0.3170188387650512141, 0.3333333333333333703, 0.3170188387650512141, 0.3333333333333333703, 0.3170188387650512141, 0.3333333333333333703, 0.3170188387650512141, 0.3333333333333333703, 0.3170188387650512141, 0.3333333333333333703, 0.3170188387650512141, 0.3333333333333333703, 0.3170188387650512141, 0.3333333333333333703, 0.3170188387650512141, 0.3333333333333333703, 0.3170188387650512141, 0.3333333333333333703, 0.3170188387650512141, 0.3333333333333333703, 0.3170188387650512141, 0.3333333333333333703, 0.3170188387650512141, 0.3333333333333333703, 0.3170188387650512141, 0.3333333333333333703, 0.3170188387650512141, 0.3333333333333333703, 0.3170188387650512141, 0.3333333333333333703, 0.3170188387650512141, 0.3333333333333333703, 0.3170188387650512141, 0.3333333333333333703, 0.3170188387650512141, 0.3333333333333333703, 0.3170188387650512141, 0.3333333333333333703, 0.3170188387650512141, 0.3333333333333333703, 0.3170188387650512141, 0.3333333333333333703, 0.3170188387650512141, 0.3333333333333333703, 0.3170188387650512141, 0.3333333333333333703, 0.3170188387650512141, 0.3333333333333333703, 0.3170188387650512141, 0.3333333333333333703, 0.3170188387650512141, 0.3333333333333333703, 0.3170188387650512141, 0.3333333333333333703, 0.3170188387650512141, 0.3333333333333333703, 0.3170188387650512141, 0.3333333333333333703, 0.3170188387650512141, 0.3333333333333333703, 0.3170188387650512141, 0.3333333333333333703, 0.3170188387650512141, 0.3333333333333333703, 0.3170188387650512141, 0.3333333333333333703, 0.3170188387650512141, 0.3333333333333333703, 0.3170188387650512141, 0.3333333333333333703, 0.3170188387650512141, 0.3333333333333333703, 0.3170188387650512141, 0.3333333333333333703, 0.3170188387650512141, 0.3333333333333333703, 0.3170188387650512141, 0.3333333333333333703, 0.3170188387650512141, 0.3333333333333333703, 0.3170188387650512141, 0.3333333333333333703, 0.3170188387650512141, 0.3333333333333333703, 0.3170188387650512141, 0.3333333333333333703, 0.3170188387650512141, 0.3333333333333333703, 0.3170188387650512141, 0.3333333333333333703, 0.3170188387650512141, 0.3333333333333333703, 0.3170188387650512141, 0.3333333333333333703, 0.3170188387650512141, 0.3333333333333333703, 0.3170188387650512141, 0.3333333333333333703, 0.3170188387650512141, 0.3333333333333333703, 0.3170188387650512141, 0.3333333333333333703, 0.3170188387650512141, 0.3333333333333333703, 0.3170188387650512141, 0.3333333333333333703, 0.3170188387650512141, 0.3333333333333333703, 0.3170188387650512141, 0.3333333333333333703, 0.3170188387650512141, 0.3333333333333333703, 0.3170188387650512141, 0.3333333333333333703, 0.3170188387650512141, 0.3333333333333333703, 0.3170188387650512141, 0.3333333333333333703, 0.3170188387650512141, 0.3333333333333333703, 0.3170188387650512141, 0.3333333333333333703, 0.3170188387650512141, 0.3333333333333333703, 0.3170188387650512141, 0.3333333333333333703, 0.3170188387650512141, 0.3333333333333333703, 0.3170188387650512141, 0.3333333333333333703, 0.3170188387650512141, 0.3333333333333333703, 0.3170188387650512141, 0.3333333333333333703, 0.3170188387650512141, 0.3333333333333333703, 0.3170188387650512141, 0.3333333333333333703, 0.3170188387650512141, 0.3333333333333333703, 0.3170188387650512141, 0.3333333333333333703, 0.3170188387650512141, 0.3333333333333333703, 0.3170188387650512141, 0.3333333333333333703, 0.3170188387650512141, 0.3333333333333333703, 0.3170188387650512141, 0.3333333333333333703, 0.3170188387650512141, 0.3333333333333333703, 0.3170188387650512141, 0.3333333333333333703, 0.3170188387650512141, 0.3333333333333333703, 0.3170188387650512141, 0.3333333333333333703, 0.3170188387650512141, 0.3333333333333333703, 0.3170188387650512141, 0.3333333333333333703, 0.3170188387650512141, 0.3333333333333333703, 0.3170188387650512141, 0.3333333333333333703, 0.3170188387650512141, 0.3333333333333333703, 0.3170188387650512141, 0.3333333333333333703, 0.3170188387650512141, 0.3333333333333333703, 0.3170188387650512141, 0.3333333333333333703, 0.3170188387650512141, 0.3333333333333333703, 0.3170188387650512141, 0.3333333333333333703, 0.3170188387650512141, 0.3333333333333333703, 0.3170188387650512141, 0.3333333333333333703, 0.3170188387650512141, 0.3333333333333333703, 0.3170188387650512141, 0.3333333333333333703, 0.3170188387650512141, 0.3333333333333333703, 0.3170188387650512141, 0.3333333333333333703, 0.3170188387650512141, 0.3333333333333333703, 0.3170188387650512141, 0.3333333333333333703, 0.3170188387650512141, 0.3333333333333333703, 0.3170188387650512141, 0.3333333333333333703, 0.3170188387650512141, 0.3333333333333333703, 0.3170188387650512141, 0.3333333333333333703, 0.3170188387650512141, 0.3333333333333333703, 0.3170188387650512141, 0.3333333333333333703, 0.3170188387650512141, 0.3333333333333333703, 0.3170188387650512141, 0.3333333333333333703, 0.3170188387650512141, 0.3333333333333333703, 0.3170188387650512141, 0.3333333333333333703, 0.3170188387650512141, 0.3333333333333333703, 0.3170188387650512141, 0.3333333333333333703, 0.3170188387650512141, 0.3333333333333333703, 0.3170188387650512141, 0.3333333333333333703, 0.3170188387650512141, 0.3333333333333333703, 0.3170188387650512141, 0.3333333333333333703, 0.3170188387650512141, 0.3333333333333333703, 0.3170188387650512141, 0.3333333333333333703, 0.3170188387650512141, 0.3333333333333333703, 0.3170188387650512141, 0.3333333333333333703, 0.3170188387650512141, 0.3333333333333333703, 0.3170188387650512141, 0.3333333333333333703, 0.3170188387650512141, 0.3333333333333333703, 0.3170188387650512141, 0.3333333333333333703, 0.3170188387650512141, 0.3333333333333333703, 0.3170188387650512141, 0.3333333333333333703, 0.3170188387650512141, 0.3333333333333333703, 0.3170188387650512141, 0.3333333333333333703, 0.3170188387650512141, 0.3333333333333333703, 0.3170188387650512141, 0.3333333333333333703, 0.3170188387650512141, 0.3333333333333333703),
 ( 1.000000000000000000, 0.9510565162951535312, 1.000000000000000000, 0.9510565162951535312, 1.000000000000000000, 0.9510565162951535312, 1.000000000000000000, 0.9510565162951535312, 1.000000000000000000, 0.9510565162951535312, 1.000000000000000000, 0.9510565162951535312, 1.000000000000000000, 0.9510565162951535312, 1.000000000000000000, 0.9510565162951535312, 1.000000000000000000, 0.9510565162951535312, 1.000000000000000000, 0.9510565162951535312, 1.000000000000000000, 0.9510565162951535312, 1.000000000000000000, 0.9510565162951535312, 1.000000000000000000, 0.9510565162951535312, 1.000000000000000000, 0.9510565162951535312, 1.000000000000000000, 0.9510565162951535312, 1.000000000000000000, 0.9510565162951535312, 1.000000000000000000, 0.9510565162951535312, 1.000000000000000000, 0.9510565162951535312, 1.000000000000000000, 0.9510565162951535312, 1.000000000000000000, 0.9510565162951535312, 1.000000000000000000, 0.9510565162951535312, 1.000000000000000000, 0.9510565162951535312, 1.000000000000000000, 0.9510565162951535312, 1.000000000000000000, 0.9510565162951535312, 1.000000000000000000, 0.9510565162951535312, 1.000000000000000000, 0.9510565162951535312, 1.000000000000000000, 0.9510565162951535312, 1.000000000000000000, 0.9510565162951535312, 1.000000000000000000, 0.9510565162951535312, 1.000000000000000000, 0.9510565162951535312, 1.000000000000000000, 0.9510565162951535312, 1.000000000000000000, 0.9510565162951535312, 1.000000000000000000, 0.9510565162951535312, 1.000000000000000000, 0.9510565162951535312, 1.000000000000000000, 0.9510565162951535312, 1.000000000000000000, 0.9510565162951535312, 1.000000000000000000, 0.9510565162951535312, 1.000000000000000000, 0.9510565162951535312, 1.000000000000000000, 0.9510565162951535312, 1.000000000000000000, 0.9510565162951535312, 1.000000000000000000, 0.9510565162951535312, 1.000000000000000000, 0.9510565162951535312, 1.000000000000000000, 0.9510565162951535312, 1.000000000000000000, 0.9510565162951535312, 1.000000000000000000, 0.9510565162951535312, 1.000000000000000000, 0.9510565162951535312, 1.000000000000000000, 0.9510565162951535312, 1.000000000000000000, 0.9510565162951535312, 1.000000000000000000, 0.9510565162951535312, 1.000000000000000000, 0.9510565162951535312, 1.000000000000000000, 0.9510565162951535312, 1.000000000000000000, 0.9510565162951535312, 1.000000000000000000, 0.9510565162951535312, 1.000000000000000000, 0.9510565162951535312, 1.000000000000000000, 0.9510565162951535312, 1.000000000000000000, 0.9510565162951535312, 1.000000000000000000, 0.9510565162951535312, 1.000000000000000000, 0.9510565162951535312, 1.000000000000000000, 0.9510565162951535312, 1.000000000000000000, 0.9510565162951535312, 1.000000000000000000, 0.9510565162951535312, 1.000000000000000000, 0.9510565162951535312, 1.000000000000000000, 0.9510565162951535312, 1.000000000000000000, 0.9510565162951535312, 1.000000000000000000, 0.9510565162951535312, 1.000000000000000000, 0.9510565162951535312, 1.000000000000000000, 0.9510565162951535312, 1.000000000000000000, 0.9510565162951535312, 1.000000000000000000, 0.9510565162951535312, 1.000000000000000000, 0.9510565162951535312, 1.000000000000000000, 0.9510565162951535312, 1.000000000000000000, 0.9510565162951535312, 1.000000000000000000, 0.9510565162951535312, 1.000000000000000000, 0.9510565162951535312, 1.000000000000000000, 0.9510565162951535312, 1.000000000000000000, 0.9510565162951535312, 1.000000000000000000, 0.9510565162951535312, 1.000000000000000000, 0.9510565162951535312, 1.000000000000000000, 0.9510565162951535312, 1.000000000000000000, 0.9510565162951535312, 1.000000000000000000, 0.9510565162951535312, 1.000000000000000000, 0.9510565162951535312, 1.000000000000000000, 0.9510565162951535312, 1.000000000000000000, 0.9510565162951535312, 1.000000000000000000, 0.9510565162951535312, 1.000000000000000000, 0.9510565162951535312, 1.000000000000000000, 0.9510565162951535312, 1.000000000000000000, 0.9510565162951535312, 1.000000000000000000, 0.9510565162951535312, 1.000000000000000000, 0.9510565162951535312, 1.000000000000000000, 0.9510565162951535312, 1.000000000000000000, 0.9510565162951535312, 1.000000000000000000, 0.9510565162951535312, 1.000000000000000000, 0.9510565162951535312, 1.000000000000000000, 0.9510565162951535312, 1.000000000000000000, 0.9510565162951535312, 1.000000000000000000, 0.9510565162951535312, 1.000000000000000000, 0.9510565162951535312, 1.000000000000000000, 0.9510565162951535312, 1.000000000000000000, 0.9510565162951535312, 1.000000000000000000, 0.9510565162951535312, 1.000000000000000000, 0.9510565162951535312, 1.000000000000000000, 0.9510565162951535312, 1.000000000000000000, 0.9510565162951535312, 1.000000000000000000, 0.9510565162951535312, 1.000000000000000000, 0.9510565162951535312, 1.000000000000000000, 0.9510565162951535312, 1.000000000000000000, 0.9510565162951535312, 1.000000000000000000, 0.9510565162951535312, 1.000000000000000000, 0.9510565162951535312, 1.000000000000000000, 0.9510565162951535312, 1.000000000000000000, 0.9510565162951535312, 1.000000000000000000, 0.9510565162951535312, 1.000000000000000000, 0.9510565162951535312, 1.000000000000000000, 0.9510565162951535312, 1.000000000000000000, 0.9510565162951535312, 1.000000000000000000, 0.9510565162951535312, 1.000000000000000000, 0.9510565162951535312, 1.000000000000000000, 0.9510565162951535312, 1.000000000000000000, 0.9510565162951535312, 1.000000000000000000, 0.9510565162951535312, 1.000000000000000000, 0.9510565162951535312, 1.000000000000000000, 0.9510565162951535312, 1.000000000000000000, 0.9510565162951535312, 1.000000000000000000, 0.9510565162951535312, 1.000000000000000000, 0.9510565162951535312, 1.000000000000000000, 0.9510565162951535312, 1.000000000000000000, 0.9510565162951535312, 1.000000000000000000, 0.9510565162951535312, 1.000000000000000000, 0.9510565162951535312, 1.000000000000000000, 0.9510565162951535312, 1.000000000000000000, 0.9510565162951535312, 1.000000000000000000, 0.9510565162951535312, 1.000000000000000000, 0.9510565162951535312, 1.000000000000000000, 0.9510565162951535312, 1.000000000000000000, 0.9510565162951535312, 1.000000000000000000, 0.9510565162951535312, 1.000000000000000000, 0.9510565162951535312, 1.000000000000000000, 0.9510565162951535312, 1.000000000000000000, 0.9510565162951535312, 1.000000000000000000, 0.9510565162951535312, 1.000000000000000000, 0.9510565162951535312, 1.000000000000000000, 0.9510565162951535312, 1.000000000000000000, 0.9510565162951535312, 1.000000000000000000, 0.9510565162951535312, 1.000000000000000000, 0.9510565162951535312, 1.000000000000000000, 0.9510565162951535312, 1.000000000000000000, 0.9510565162951535312, 1.000000000000000000, 0.9510565162951535312, 1.000000000000000000, 0.9510565162951535312, 1.000000000000000000, 0.9510565162951535312, 1.000000000000000000, 0.9510565162951535312, 1.000000000000000000, 0.9510565162951535312, 1.000000000000000000, 0.9510565162951535312, 1.000000000000000000, 0.9510565162951535312, 1.000000000000000000, 0.9510565162951535312, 1.000000000000000000, 0.9510565162951535312, 1.000000000000000000, 0.9510565162951535312, 1.000000000000000000, 0.9510565162951535312, 1.000000000000000000, 0.9510565162951535312, 1.000000000000000000, 0.9510565162951535312, 1.000000000000000000, 0.9510565162951535312, 1.000000000000000000, 0.9510565162951535312, 1.000000000000000000, 0.9510565162951535312, 1.000000000000000000, 0.9510565162951535312, 1.000000000000000000),
 ( 0.3333333333333333703, 0.3170188387650512141, 0.3333333333333333703, 0.3170188387650512141, 0.3333333333333333703, 0.3170188387650512141, 0.3333333333333333703, 0.3170188387650512141, 0.3333333333333333703, 0.3170188387650512141, 0.3333333333333333703, 0.3170188387650512141, 0.3333333333333333703, 0.3170188387650512141, 0.3333333333333333703, 0.3170188387650512141, 0.3333333333333333703, 0.3170188387650512141, 0.3333333333333333703, 0.3170188387650512141, 0.3333333333333333703, 0.3170188387650512141, 0.3333333333333333703, 0.3170188387650512141, 0.3333333333333333703, 0.3170188387650512141, 0.3333333333333333703, 0.3170188387650512141, 0.3333333333333333703, 0.3170188387650512141, 0.3333333333333333703, 0.3170188387650512141, 0.3333333333333333703, 0.3170188387650512141, 0.3333333333333333703, 0.3170188387650512141, 0.3333333333333333703, 0.3170188387650512141, 0.3333333333333333703, 0.3170188387650512141, 0.3333333333333333703, 0.3170188387650512141, 0.3333333333333333703, 0.3170188387650512141, 0.3333333333333333703, 0.3170188387650512141, 0.3333333333333333703, 0.3170188387650512141, 0.3333333333333333703, 0.3170188387650512141, 0.3333333333333333703, 0.3170188387650512141, 0.3333333333333333703, 0.3170188387650512141, 0.3333333333333333703, 0.3170188387650512141, 0.3333333333333333703, 0.3170188387650512141, 0.3333333333333333703, 0.3170188387650512141, 0.3333333333333333703, 0.3170188387650512141, 0.3333333333333333703, 0.3170188387650512141, 0.3333333333333333703, 0.3170188387650512141, 0.3333333333333333703, 0.3170188387650512141, 0.3333333333333333703, 0.3170188387650512141, 0.3333333333333333703, 0.3170188387650512141, 0.3333333333333333703, 0.3170188387650512141, 0.3333333333333333703, 0.3170188387650512141, 0.3333333333333333703, 0.3170188387650512141, 0.3333333333333333703, 0.3170188387650512141, 0.3333333333333333703, 0.3170188387650512141, 0.3333333333333333703, 0.3170188387650512141, 0.3333333333333333703, 0.3170188387650512141, 0.3333333333333333703, 0.3170188387650512141, 0.3333333333333333703, 0.3170188387650512141, 0.3333333333333333703, 0.3170188387650512141, 0.3333333333333333703, 0.3170188387650512141, 0.3333333333333333703, 0.3170188387650512141, 0.3333333333333333703, 0.3170188387650512141, 0.3333333333333333703, 0.3170188387650512141, 0.3333333333333333703, 0.3170188387650512141, 0.3333333333333333703, 0.3170188387650512141, 0.3333333333333333703, 0.3170188387650512141, 0.3333333333333333703, 0.3170188387650512141, 0.3333333333333333703, 0.3170188387650512141, 0.3333333333333333703, 0.3170188387650512141, 0.3333333333333333703, 0.3170188387650512141, 0.3333333333333333703, 0.3170188387650512141, 0.3333333333333333703, 0.3170188387650512141, 0.3333333333333333703, 0.3170188387650512141, 0.3333333333333333703, 0.3170188387650512141, 0.3333333333333333703, 0.3170188387650512141, 0.3333333333333333703, 0.3170188387650512141, 0.3333333333333333703, 0.3170188387650512141, 0.3333333333333333703, 0.3170188387650512141, 0.3333333333333333703, 0.3170188387650512141, 0.3333333333333333703, 0.3170188387650512141, 0.3333333333333333703, 0.3170188387650512141, 0.3333333333333333703, 0.3170188387650512141, 0.3333333333333333703, 0.3170188387650512141, 0.3333333333333333703, 0.3170188387650512141, 0.3333333333333333703, 0.3170188387650512141, 0.3333333333333333703, 0.3170188387650512141, 0.3333333333333333703, 0.3170188387650512141, 0.3333333333333333703, 0.3170188387650512141, 0.3333333333333333703, 0.3170188387650512141, 0.3333333333333333703, 0.3170188387650512141, 0.3333333333333333703, 0.3170188387650512141, 0.3333333333333333703, 0.3170188387650512141, 0.3333333333333333703, 0.3170188387650512141, 0.3333333333333333703, 0.3170188387650512141, 0.3333333333333333703, 0.3170188387650512141, 0.3333333333333333703, 0.3170188387650512141, 0.3333333333333333703, 0.3170188387650512141, 0.3333333333333333703, 0.3170188387650512141, 0.3333333333333333703, 0.3170188387650512141, 0.3333333333333333703, 0.3170188387650512141, 0.3333333333333333703, 0.3170188387650512141, 0.3333333333333333703, 0.3170188387650512141, 0.3333333333333333703, 0.3170188387650512141, 0.3333333333333333703, 0.3170188387650512141, 0.3333333333333333703, 0.3170188387650512141, 0.3333333333333333703, 0.3170188387650512141, 0.3333333333333333703, 0.3170188387650512141, 0.3333333333333333703, 0.3170188387650512141, 0.3333333333333333703, 0.3170188387650512141, 0.3333333333333333703, 0.3170188387650512141, 0.3333333333333333703, 0.3170188387650512141, 0.3333333333333333703, 0.3170188387650512141, 0.3333333333333333703, 0.3170188387650512141, 0.3333333333333333703, 0.3170188387650512141, 0.3333333333333333703, 0.3170188387650512141, 0.3333333333333333703, 0.3170188387650512141, 0.3333333333333333703, 0.3170188387650512141, 0.3333333333333333703, 0.3170188387650512141, 0.3333333333333333703, 0.3170188387650512141, 0.3333333333333333703, 0.3170188387650512141, 0.3333333333333333703, 0.3170188387650512141, 0.3333333333333333703, 0.3170188387650512141, 0.3333333333333333703, 0.3170188387650512141, 0.3333333333333333703, 0.3170188387650512141, 0.3333333333333333703, 0.3170188387650512141, 0.3333333333333333703, 0.3170188387650512141, 0.3333333333333333703, 0.3170188387650512141, 0.3333333333333333703, 0.3170188387650512141, 0.3333333333333333703, 0.3170188387650512141, 0.3333333333333333703, 0.3170188387650512141, 0.3333333333333333703, 0.3170188387650512141, 0.3333333333333333703, 0.3170188387650512141, 0.3333333333333333703, 0.3170188387650512141, 0.3333333333333333703, 0.3170188387650512141, 0.3333333333333333703, 0.3170188387650512141, 0.3333333333333333703, 0.3170188387650512141, 0.3333333333333333703, 0.3170188387650512141, 0.3333333333333333703, 0.3170188387650512141, 0.3333333333333333703, 0.3170188387650512141, 0.3333333333333333703, 0.3170188387650512141, 0.3333333333333333703, 0.3170188387650512141, 0.3333333333333333703, 0.3170188387650512141, 0.3333333333333333703, 0.3170188387650512141, 0.3333333333333333703, 0.3170188387650512141, 0.3333333333333333703, 0.3170188387650512141, 0.3333333333333333703, 0.3170188387650512141, 0.3333333333333333703, 0.3170188387650512141, 0.3333333333333333703, 0.3170188387650512141, 0.3333333333333333703, 0.3170188387650512141, 0.3333333333333333703, 0.3170188387650512141, 0.3333333333333333703, 0.3170188387650512141, 0.3333333333333333703, 0.3170188387650512141, 0.3333333333333333703, 0.3170188387650512141, 0.3333333333333333703, 0.3170188387650512141, 0.3333333333333333703, 0.3170188387650512141, 0.3333333333333333703, 0.3170188387650512141, 0.3333333333333333703, 0.3170188387650512141, 0.3333333333333333703, 0.3170188387650512141, 0.3333333333333333703, 0.3170188387650512141, 0.3333333333333333703, 0.3170188387650512141, 0.3333333333333333703, 0.3170188387650512141, 0.3333333333333333703, 0.3170188387650512141, 0.3333333333333333703, 0.3170188387650512141, 0.3333333333333333703, 0.3170188387650512141, 0.3333333333333333703, 0.3170188387650512141, 0.3333333333333333703, 0.3170188387650512141, 0.3333333333333333703, 0.3170188387650512141, 0.3333333333333333703, 0.3170188387650512141, 0.3333333333333333703, 0.3170188387650512141, 0.3333333333333333703, 0.3170188387650512141, 0.3333333333333333703, 0.3170188387650512141, 0.3333333333333333703, 0.3170188387650512141, 0.3333333333333333703, 0.3170188387650512141, 0.3333333333333333703, 0.3170188387650512141, 0.3333333333333333703, 0.3170188387650512141, 0.3333333333333333703, 0.3170188387650512141, 0.3333333333333333703, 0.3170188387650512141, 0.3333333333333333703, 0.3170188387650512141, 0.3333333333333333703),
 ( 0.3333333333333333703, 0.3170188387650512141, 0.3333333333333333703, 0.3170188387650512141, 0.3333333333333333703, 0.3170188387650512141, 0.3333333333333333703, 0.3170188387650512141, 0.3333333333333333703, 0.3170188387650512141, 0.3333333333333333703, 0.3170188387650512141, 0.3333333333333333703, 0.3170188387650512141, 0.3333333333333333703, 0.3170188387650512141, 0.3333333333333333703, 0.3170188387650512141, 0.3333333333333333703, 0.3170188387650512141, 0.3333333333333333703, 0.3170188387650512141, 0.3333333333333333703, 0.3170188387650512141, 0.3333333333333333703, 0.3170188387650512141, 0.3333333333333333703, 0.3170188387650512141, 0.3333333333333333703, 0.3170188387650512141, 0.3333333333333333703, 0.3170188387650512141, 0.3333333333333333703, 0.3170188387650512141, 0.3333333333333333703, 0.3170188387650512141, 0.3333333333333333703, 0.3170188387650512141, 0.3333333333333333703, 0.3170188387650512141, 0.3333333333333333703, 0.3170188387650512141, 0.3333333333333333703, 0.3170188387650512141, 0.3333333333333333703, 0.3170188387650512141, 0.3333333333333333703, 0.3170188387650512141, 0.3333333333333333703, 0.3170188387650512141, 0.3333333333333333703, 0.3170188387650512141, 0.3333333333333333703, 0.3170188387650512141, 0.3333333333333333703, 0.3170188387650512141, 0.3333333333333333703, 0.3170188387650512141, 0.3333333333333333703, 0.3170188387650512141, 0.3333333333333333703, 0.3170188387650512141, 0.3333333333333333703, 0.3170188387650512141, 0.3333333333333333703, 0.3170188387650512141, 0.3333333333333333703, 0.3170188387650512141, 0.3333333333333333703, 0.3170188387650512141, 0.3333333333333333703, 0.3170188387650512141, 0.3333333333333333703, 0.3170188387650512141, 0.3333333333333333703, 0.3170188387650512141, 0.3333333333333333703, 0.3170188387650512141, 0.3333333333333333703, 0.3170188387650512141, 0.3333333333333333703, 0.3170188387650512141, 0.3333333333333333703, 0.3170188387650512141, 0.3333333333333333703, 0.3170188387650512141, 0.3333333333333333703, 0.3170188387650512141, 0.3333333333333333703, 0.3170188387650512141, 0.3333333333333333703, 0.3170188387650512141, 0.3333333333333333703, 0.3170188387650512141, 0.3333333333333333703, 0.3170188387650512141, 0.3333333333333333703, 0.3170188387650512141, 0.3333333333333333703, 0.3170188387650512141, 0.3333333333333333703, 0.3170188387650512141, 0.3333333333333333703, 0.3170188387650512141, 0.3333333333333333703, 0.3170188387650512141, 0.3333333333333333703, 0.3170188387650512141, 0.3333333333333333703, 0.3170188387650512141, 0.3333333333333333703, 0.3170188387650512141, 0.3333333333333333703, 0.3170188387650512141, 0.3333333333333333703, 0.3170188387650512141, 0.3333333333333333703, 0.3170188387650512141, 0.3333333333333333703, 0.3170188387650512141, 0.3333333333333333703, 0.3170188387650512141, 0.3333333333333333703, 0.3170188387650512141, 0.3333333333333333703, 0.3170188387650512141, 0.3333333333333333703, 0.3170188387650512141, 0.3333333333333333703, 0.3170188387650512141, 0.3333333333333333703, 0.3170188387650512141, 0.3333333333333333703, 0.3170188387650512141, 0.3333333333333333703, 0.3170188387650512141, 0.3333333333333333703, 0.3170188387650512141, 0.3333333333333333703, 0.3170188387650512141, 0.3333333333333333703, 0.3170188387650512141, 0.3333333333333333703, 0.3170188387650512141, 0.3333333333333333703, 0.3170188387650512141, 0.3333333333333333703, 0.3170188387650512141, 0.3333333333333333703, 0.3170188387650512141, 0.3333333333333333703, 0.3170188387650512141, 0.3333333333333333703, 0.3170188387650512141, 0.3333333333333333703, 0.3170188387650512141, 0.3333333333333333703, 0.3170188387650512141, 0.3333333333333333703, 0.3170188387650512141, 0.3333333333333333703, 0.3170188387650512141, 0.3333333333333333703, 0.3170188387650512141, 0.3333333333333333703, 0.3170188387650512141, 0.3333333333333333703, 0.3170188387650512141, 0.3333333333333333703, 0.3170188387650512141, 0.3333333333333333703, 0.3170188387650512141, 0.3333333333333333703, 0.3170188387650512141, 0.3333333333333333703, 0.3170188387650512141, 0.3333333333333333703, 0.3170188387650512141, 0.3333333333333333703, 0.3170188387650512141, 0.3333333333333333703, 0.3170188387650512141, 0.3333333333333333703, 0.3170188387650512141, 0.3333333333333333703, 0.3170188387650512141, 0.3333333333333333703, 0.3170188387650512141, 0.3333333333333333703, 0.3170188387650512141, 0.3333333333333333703, 0.3170188387650512141, 0.3333333333333333703, 0.3170188387650512141, 0.3333333333333333703, 0.3170188387650512141, 0.3333333333333333703, 0.3170188387650512141, 0.3333333333333333703, 0.3170188387650512141, 0.3333333333333333703, 0.3170188387650512141, 0.3333333333333333703, 0.3170188387650512141, 0.3333333333333333703, 0.3170188387650512141, 0.3333333333333333703, 0.3170188387650512141, 0.3333333333333333703, 0.3170188387650512141, 0.3333333333333333703, 0.3170188387650512141, 0.3333333333333333703, 0.3170188387650512141, 0.3333333333333333703, 0.3170188387650512141, 0.3333333333333333703, 0.3170188387650512141, 0.3333333333333333703, 0.3170188387650512141, 0.3333333333333333703, 0.3170188387650512141, 0.3333333333333333703, 0.3170188387650512141, 0.3333333333333333703, 0.3170188387650512141, 0.3333333333333333703, 0.3170188387650512141, 0.3333333333333333703, 0.3170188387650512141, 0.3333333333333333703, 0.3170188387650512141, 0.3333333333333333703, 0.3170188387650512141, 0.3333333333333333703, 0.3170188387650512141, 0.3333333333333333703, 0.3170188387650512141, 0.3333333333333333703, 0.3170188387650512141, 0.3333333333333333703, 0.3170188387650512141, 0.3333333333333333703, 0.3170188387650512141, 0.3333333333333333703, 0.3170188387650512141, 0.3333333333333333703, 0.3170188387650512141, 0.3333333333333333703, 0.3170188387650512141, 0.3333333333333333703, 0.3170188387650512141, 0.3333333333333333703, 0.3170188387650512141, 0.3333333333333333703, 0.3170188387650512141, 0.3333333333333333703, 0.3170188387650512141, 0.3333333333333333703, 0.3170188387650512141, 0.3333333333333333703, 0.3170188387650512141, 0.3333333333333333703, 0.3170188387650512141, 0.3333333333333333703, 0.3170188387650512141, 0.3333333333333333703, 0.3170188387650512141, 0.3333333333333333703, 0.3170188387650512141, 0.3333333333333333703, 0.3170188387650512141, 0.3333333333333333703, 0.3170188387650512141, 0.3333333333333333703, 0.3170188387650512141, 0.3333333333333333703, 0.3170188387650512141, 0.3333333333333333703, 0.3170188387650512141, 0.3333333333333333703, 0.3170188387650512141, 0.3333333333333333703, 0.3170188387650512141, 0.3333333333333333703, 0.3170188387650512141, 0.3333333333333333703, 0.3170188387650512141, 0.3333333333333333703, 0.3170188387650512141, 0.3333333333333333703, 0.3170188387650512141, 0.3333333333333333703, 0.3170188387650512141, 0.3333333333333333703, 0.3170188387650512141, 0.3333333333333333703, 0.3170188387650512141, 0.3333333333333333703, 0.3170188387650512141, 0.3333333333333333703, 0.3170188387650512141, 0.3333333333333333703, 0.3170188387650512141, 0.3333333333333333703, 0.3170188387650512141, 0.3333333333333333703, 0.3170188387650512141, 0.3333333333333333703, 0.3170188387650512141, 0.3333333333333333703, 0.3170188387650512141, 0.3333333333333333703, 0.3170188387650512141, 0.3333333333333333703, 0.3170188387650512141, 0.3333333333333333703, 0.3170188387650512141, 0.3333333333333333703, 0.3170188387650512141, 0.3333333333333333703, 0.3170188387650512141, 0.3333333333333333703, 0.3170188387650512141, 0.3333333333333333703, 0.3170188387650512141, 0.3333333333333333703, 0.3170188387650512141, 0.3333333333333333703, 0.3170188387650512141, 0.3333333333333333703),
 ( 1.000000000000000000, 0.9510565162951535312, 1.000000000000000000, 0.9510565162951535312, 1.000000000000000000, 0.9510565162951535312, 1.000000000000000000, 0.9510565162951535312, 1.000000000000000000, 0.9510565162951535312, 1.000000000000000000, 0.9510565162951535312, 1.000000000000000000, 0.9510565162951535312, 1.000000000000000000, 0.9510565162951535312, 1.000000000000000000, 0.9510565162951535312, 1.000000000000000000, 0.9510565162951535312, 1.000000000000000000, 0.9510565162951535312, 1.000000000000000000, 0.9510565162951535312, 1.000000000000000000, 0.9510565162951535312, 1.000000000000000000, 0.9510565162951535312, 1.000000000000000000, 0.9510565162951535312, 1.000000000000000000, 0.9510565162951535312, 1.000000000000000000, 0.9510565162951535312, 1.000000000000000000, 0.9510565162951535312, 1.000000000000000000, 0.9510565162951535312, 1.000000000000000000, 0.9510565162951535312, 1.000000000000000000, 0.9510565162951535312, 1.000000000000000000, 0.9510565162951535312, 1.000000000000000000, 0.9510565162951535312, 1.000000000000000000, 0.9510565162951535312, 1.000000000000000000, 0.9510565162951535312, 1.000000000000000000, 0.9510565162951535312, 1.000000000000000000, 0.9510565162951535312, 1.000000000000000000, 0.9510565162951535312, 1.000000000000000000, 0.9510565162951535312, 1.000000000000000000, 0.9510565162951535312, 1.000000000000000000, 0.9510565162951535312, 1.000000000000000000, 0.9510565162951535312, 1.000000000000000000, 0.9510565162951535312, 1.000000000000000000, 0.9510565162951535312, 1.000000000000000000, 0.9510565162951535312, 1.000000000000000000, 0.9510565162951535312, 1.000000000000000000, 0.9510565162951535312, 1.000000000000000000, 0.9510565162951535312, 1.000000000000000000, 0.9510565162951535312, 1.000000000000000000, 0.9510565162951535312, 1.000000000000000000, 0.9510565162951535312, 1.000000000000000000, 0.9510565162951535312, 1.000000000000000000, 0.9510565162951535312, 1.000000000000000000, 0.9510565162951535312, 1.000000000000000000, 0.9510565162951535312, 1.000000000000000000, 0.9510565162951535312, 1.000000000000000000, 0.9510565162951535312, 1.000000000000000000, 0.9510565162951535312, 1.000000000000000000, 0.9510565162951535312, 1.000000000000000000, 0.9510565162951535312, 1.000000000000000000, 0.9510565162951535312, 1.000000000000000000, 0.9510565162951535312, 1.000000000000000000, 0.9510565162951535312, 1.000000000000000000, 0.9510565162951535312, 1.000000000000000000, 0.9510565162951535312, 1.000000000000000000, 0.9510565162951535312, 1.000000000000000000, 0.9510565162951535312, 1.000000000000000000, 0.9510565162951535312, 1.000000000000000000, 0.9510565162951535312, 1.000000000000000000, 0.9510565162951535312, 1.000000000000000000, 0.9510565162951535312, 1.000000000000000000, 0.9510565162951535312, 1.000000000000000000, 0.9510565162951535312, 1.000000000000000000, 0.9510565162951535312, 1.000000000000000000, 0.9510565162951535312, 1.000000000000000000, 0.9510565162951535312, 1.000000000000000000, 0.9510565162951535312, 1.000000000000000000, 0.9510565162951535312, 1.000000000000000000, 0.9510565162951535312, 1.000000000000000000, 0.9510565162951535312, 1.000000000000000000, 0.9510565162951535312, 1.000000000000000000, 0.9510565162951535312, 1.000000000000000000, 0.9510565162951535312, 1.000000000000000000, 0.9510565162951535312, 1.000000000000000000, 0.9510565162951535312, 1.000000000000000000, 0.9510565162951535312, 1.000000000000000000, 0.9510565162951535312, 1.000000000000000000, 0.9510565162951535312, 1.000000000000000000, 0.9510565162951535312, 1.000000000000000000, 0.9510565162951535312, 1.000000000000000000, 0.9510565162951535312, 1.000000000000000000, 0.9510565162951535312, 1.000000000000000000, 0.9510565162951535312, 1.000000000000000000, 0.9510565162951535312, 1.000000000000000000, 0.9510565162951535312, 1.000000000000000000, 0.9510565162951535312, 1.000000000000000000, 0.9510565162951535312, 1.000000000000000000, 0.9510565162951535312, 1.000000000000000000, 0.9510565162951535312, 1.000000000000000000, 0.9510565162951535312, 1.000000000000000000, 0.9510565162951535312, 1.000000000000000000, 0.9510565162951535312, 1.000000000000000000, 0.9510565162951535312, 1.000000000000000000, 0.9510565162951535312, 1.000000000000000000, 0.9510565162951535312, 1.000000000000000000, 0.9510565162951535312, 1.000000000000000000, 0.9510565162951535312, 1.000000000000000000, 0.9510565162951535312, 1.000000000000000000, 0.9510565162951535312, 1.000000000000000000, 0.9510565162951535312, 1.000000000000000000, 0.9510565162951535312, 1.000000000000000000, 0.9510565162951535312, 1.000000000000000000, 0.9510565162951535312, 1.000000000000000000, 0.9510565162951535312, 1.000000000000000000, 0.9510565162951535312, 1.000000000000000000, 0.9510565162951535312, 1.000000000000000000, 0.9510565162951535312, 1.000000000000000000, 0.9510565162951535312, 1.000000000000000000, 0.9510565162951535312, 1.000000000000000000, 0.9510565162951535312, 1.000000000000000000, 0.9510565162951535312, 1.000000000000000000, 0.9510565162951535312, 1.000000000000000000, 0.9510565162951535312, 1.000000000000000000, 0.9510565162951535312, 1.000000000000000000, 0.9510565162951535312, 1.000000000000000000, 0.9510565162951535312, 1.000000000000000000, 0.9510565162951535312, 1.000000000000000000, 0.9510565162951535312, 1.000000000000000000, 0.9510565162951535312, 1.000000000000000000, 0.9510565162951535312, 1.000000000000000000, 0.9510565162951535312, 1.000000000000000000, 0.9510565162951535312, 1.000000000000000000, 0.9510565162951535312, 1.000000000000000000, 0.9510565162951535312, 1.000000000000000000, 0.9510565162951535312, 1.000000000000000000, 0.9510565162951535312, 1.000000000000000000, 0.9510565162951535312, 1.000000000000000000, 0.9510565162951535312, 1.000000000000000000, 0.9510565162951535312, 1.000000000000000000, 0.9510565162951535312, 1.000000000000000000, 0.9510565162951535312, 1.000000000000000000, 0.9510565162951535312, 1.000000000000000000, 0.9510565162951535312, 1.000000000000000000, 0.9510565162951535312, 1.000000000000000000, 0.9510565162951535312, 1.000000000000000000, 0.9510565162951535312, 1.000000000000000000, 0.9510565162951535312, 1.000000000000000000, 0.9510565162951535312, 1.000000000000000000, 0.9510565162951535312, 1.000000000000000000, 0.9510565162951535312, 1.000000000000000000, 0.9510565162951535312, 1.000000000000000000, 0.9510565162951535312, 1.000000000000000000, 0.9510565162951535312, 1.000000000000000000, 0.9510565162951535312, 1.000000000000000000, 0.9510565162951535312, 1.000000000000000000, 0.9510565162951535312, 1.000000000000000000, 0.9510565162951535312, 1.000000000000000000, 0.9510565162951535312, 1.000000000000000000, 0.9510565162951535312, 1.000000000000000000, 0.9510565162951535312, 1.000000000000000000, 0.9510565162951535312, 1.000000000000000000, 0.9510565162951535312, 1.000000000000000000, 0.9510565162951535312, 1.000000000000000000, 0.9510565162951535312, 1.000000000000000000, 0.9510565162951535312, 1.000000000000000000, 0.9510565162951535312, 1.000000000000000000, 0.9510565162951535312, 1.000000000000000000, 0.9510565162951535312, 1.000000000000000000, 0.9510565162951535312, 1.000000000000000000, 0.9510565162951535312, 1.000000000000000000, 0.9510565162951535312, 1.000000000000000000, 0.9510565162951535312, 1.000000000000000000, 0.9510565162951535312, 1.000000000000000000, 0.9510565162951535312, 1.000000000000000000, 0.9510565162951535312, 1.000000000000000000) ) ) 
 REPRESENTATION_ITEM ( '' )  SURFACE ( )  );
#13569=PLANE ( 'NONE',  #9453 ) ;
#13574=CARTESIAN_POINT ( 'NONE',  ( 0.7417250638684235176, 23.11142975074950101, -61.19295307432605568 ) ) ;
#13578=CARTESIAN_POINT ( 'NONE',  ( 0.5331684895902240040, 13.15756906230466328, -38.55704692567387326 ) ) ;
#13582=CARTESIAN_POINT ( 'NONE',  ( 0.8348115903393232839, 13.20534463599456387, -74.54295307432605000 ) ) ;
#13583=CARTESIAN_POINT ( 'NONE',  ( 3.043106805520193525, 20.33772366180932067, -67.50704692567386189 ) ) ;
#13591=CARTESIAN_POINT ( 'NONE',  ( -4.107178604518053611, 16.84948681541050775, -40.79999999999996874 ) ) ;
#13594=CARTESIAN_POINT ( 'NONE',  ( -1.028604700431329233, 11.93400751992799513, -29.70704692567387184 ) ) ;
#13596=CARTESIAN_POINT ( 'NONE',  ( 2.940415233664778416, 20.44041523366473712, -56.99999999999996447 ) ) ;
#13608=CARTESIAN_POINT ( 'NONE',  ( -2.564989113914250662, 12.12957133169093282, -32.84295307432606137 ) ) ;
#13628=CARTESIAN_POINT ( 'NONE',  ( 0.6839900399647733664, 13.18145684914961357, -46.04999999999996163 ) ) ;
#13638=CARTESIAN_POINT ( 'NONE',  ( -1.985016409143819605, 13.60418594181426855, -67.34999999999996589 ) ) ;
#13640=CARTESIAN_POINT ( 'NONE',  ( -4.099003336600151925, 21.81495595370741469, -57.75704692567386900 ) ) ;
#13641=CARTESIAN_POINT ( 'NONE',  ( -5.876318620034919782, 18.43071743580290089, -43.94999999999996021 ) ) ;
#13655=CARTESIAN_POINT ( 'NONE',  ( 0.7798958854283032371, 11.59979359312010772, -41.55704692567387326 ) ) ;
#13660=CARTESIAN_POINT ( 'NONE',  ( 1.081538986177402295, 11.64756916681001186, -62.54295307432605711 ) ) ;
#13677=CARTESIAN_POINT ( 'NONE',  ( 4.206979645153767322, 13.29302035484617051, -27.74999999999995381 ) ) ;
#13680=CARTESIAN_POINT ( 'NONE',  ( 0.7939530028709752552, 21.58445996917927445, -52.20704692567388605 ) ) ;
#13681=CARTESIAN_POINT ( 'NONE',  ( 2.940415233664778416, 20.44041523366473712, -41.99999999999996447 ) ) ;
#13682=FACE_OUTER_BOUND ( 'NONE', #25753, .T. ) ;
#13690=CARTESIAN_POINT ( 'NONE',  ( -4.107178604518053611, 16.84948681541050775, -52.79999999999996874 ) ) ;
#13692=CARTESIAN_POINT ( 'NONE',  ( 3.639207298612508801, 15.48273827966686866, -32.10704692567387042 ) ) ;
#13693=CARTESIAN_POINT ( 'NONE',  ( 5.301103610786608300, 20.20104720010254340, -72.14999999999996305 ) ) ;
#13697=CARTESIAN_POINT ( 'NONE',  ( 4.084459969179292216, 18.29395300287091430, -31.79295307432605355 ) ) ;
#13707=CARTESIAN_POINT ( 'NONE',  ( -3.965139115708213868, 15.65104167704456906, -24.15704692567387468 ) ) ;
#13713=CARTESIAN_POINT ( 'NONE',  ( 5.301103610786608300, 20.20104720010253985, -39.14999999999997016 ) ) ;
#13733=CARTESIAN_POINT ( 'NONE',  ( -5.301103610786608300, 14.79895279989743706, -61.64999999999995595 ) ) ;
#13739=CARTESIAN_POINT ( 'NONE',  ( 3.705139346311793869, 15.61213720913094960, -36.59999999999996589 ) ) ;
#13740=CARTESIAN_POINT ( 'NONE',  ( 3.895814058185739892, 19.48501640914376054, -63.14999999999997016 ) ) ;
#13753=CARTESIAN_POINT ( 'NONE',  ( 4.342430937695320736, 16.96683151040971538, -43.94295307432605568 ) ) ;
#13758=CARTESIAN_POINT ( 'NONE',  ( 0.5070733663080689846, 21.62989723985679902, -67.19295307432605568 ) ) ;
#13769=CARTESIAN_POINT ( 'NONE',  ( -4.318543150850367773, 18.18399003996480801, -28.94999999999996021 ) ) ;
#13776=CARTESIAN_POINT ( 'NONE',  ( 2.568848540478311460, 12.45835086740561692, -69.89999999999996305 ) ) ;
#13794=CARTESIAN_POINT ( 'NONE',  ( -1.081538986177402961, 23.35243083318996327, -64.04295307432605000 ) ) ;
#13803=CARTESIAN_POINT ( 'NONE',  ( -3.826489000663265472, 15.37892550466785480, -75.14295307432605853 ) ) ;
#13804=CARTESIAN_POINT ( 'NONE',  ( -2.121074495332175847, 13.67351099933674341, -68.85704692567387042 ) ) ;
#13815=CARTESIAN_POINT ( 'NONE',  ( 2.837105286290961370, 22.73177855326409613, -25.35704692567387042 ) ) ;
#13817=CARTESIAN_POINT ( 'NONE',  ( -3.895814058185739448, 15.51498359085620571, -55.64999999999994174 ) ) ;
#13829=CARTESIAN_POINT ( 'NONE',  ( 5.231778553264135212, 20.33710528629089254, -31.64295307432605853 ) ) ;
#13846=CARTESIAN_POINT ( 'NONE',  ( -4.107178604518053611, 16.84948681541050775, -43.79999999999996163 ) ) ;
#13856=CARTESIAN_POINT ( 'NONE',  ( 3.091735541773220852, 14.40826445822673563, -66.74999999999997158 ) ) ;
#13857=CARTESIAN_POINT ( 'NONE',  ( 2.439449611014226971, 12.39241881970633230, -59.40704692567388179 ) ) ;
#13858=CARTESIAN_POINT ( 'NONE',  ( -4.206979645153769098, 21.70697964515380107, -50.24999999999997158 ) ) ;
#13872=CARTESIAN_POINT ( 'NONE',  ( -4.103766977300021601, 13.60161616641083704, -42.00704692567387610 ) ) ;
#13877=CARTESIAN_POINT ( 'NONE',  ( 4.314955953707388936, 13.40099666339979123, -56.24295307432605995 ) ) ;
#13891=CARTESIAN_POINT ( 'NONE',  ( 2.568848540478311460, 12.45835086740561692, -30.89999999999996305 ) ) ;
#13894=CARTESIAN_POINT ( 'NONE',  ( 4.294655364005415699, 16.66518840966061887, -52.95704692567387895 ) ) ;
#13895=CARTESIAN_POINT ( 'NONE',  ( 4.318543150850367773, 16.81600996003516357, -72.44999999999994600 ) ) ;
#13904=CARTESIAN_POINT ( 'NONE',  ( 1.985016409143818272, 21.39581405818570303, -50.84999999999997300 ) ) ;
#13906=CARTESIAN_POINT ( 'NONE',  ( -3.639207298612509689, 19.51726172033310647, -39.60704692567387042 ) ) ;
#13907=CARTESIAN_POINT ( 'NONE',  ( 5.876318620034919782, 16.56928256419707068, -72.44999999999996021 ) ) ;
#13911=CARTESIAN_POINT ( 'NONE',  ( 4.342430937695320736, 16.96683151040971538, -31.94295307432605568 ) ) ;
#13918=CARTESIAN_POINT ( 'NONE',  ( -5.611429750749524992, 16.75827493613162034, -72.30704692567387326 ) ) ;
#13925=CARTESIAN_POINT ( 'NONE',  ( -2.701047200102606016, 12.19889638921340413, -37.34999999999994458 ) ) ;
#13941=ADVANCED_FACE ( 'NONE', ( #18849 ), #15886, .T. ) ;
#13946=CARTESIAN_POINT ( 'NONE',  ( 5.588711115410763597, 18.38516488214980882, -60.29999999999996163 ) ) ;
#13951=CARTESIAN_POINT ( 'NONE',  ( 2.940415233664778416, 20.44041523366473712, -29.99999999999996447 ) ) ;
#13952=CARTESIAN_POINT ( 'NONE',  ( 1.887862790868997109, 13.79486065368817194, -63.89999999999997016 ) ) ;
#13963=CARTESIAN_POINT ( 'NONE',  ( -0.8348115903393239501, 21.79465536400541126, -49.04295307432606421 ) ) ;
#13968=CARTESIAN_POINT ( 'NONE',  ( -0.8348115903393239501, 21.79465536400541126, -61.04295307432605711 ) ) ;
#13979=CARTESIAN_POINT ( 'NONE',  ( 3.091735541773220852, 14.40826445822673563, -30.74999999999995737 ) ) ;
#13989=CARTESIAN_POINT ( 'NONE',  ( 0.8851648821498760977, 23.08871111541074228, -71.69999999999997442 ) ) ;
#14012=CARTESIAN_POINT ( 'NONE',  ( 5.107581180293630396, 15.06055038898570686, -59.09295307432605426 ) ) ;
#14020=CARTESIAN_POINT ( 'NONE',  ( 2.698247469942395949, 12.52428291510489977, -29.39295307432606208 ) ) ;
#14022=CARTESIAN_POINT ( 'NONE',  ( 0.7939530028709752552, 21.58445996917927445, -67.20704692567387895 ) ) ;
#14034=CARTESIAN_POINT ( 'NONE',  ( 0.7798958854283032371, 11.59979359312010772, -26.55704692567386971 ) ) ;
#14036=CARTESIAN_POINT ( 'NONE',  ( -3.895814058185739448, 15.51498359085620571, -52.64999999999997016 ) ) ;
#14048=CARTESIAN_POINT ( 'NONE',  ( -5.565992480072003978, 16.47139529956871229, -30.29295307432605355 ) ) ;
#14066=CARTESIAN_POINT ( 'NONE',  ( 0.6505131845895220088, 21.60717860451803674, -44.69999999999996021 ) ) ;
#14075=CARTESIAN_POINT ( 'NONE',  ( 3.705139346311793869, 15.61213720913094960, -63.59999999999995879 ) ) ;
#14077=CARTESIAN_POINT ( 'NONE',  ( 2.439449611014226971, 12.39241881970633230, -53.40704692567386758 ) ) ;
#14078=CARTESIAN_POINT ( 'NONE',  ( 5.588711115410763597, 18.38516488214980882, -45.29999999999996874 ) ) ;
#14090=CARTESIAN_POINT ( 'NONE',  ( 2.837105286290961370, 22.73177855326409613, -34.35704692567387752 ) ) ;
#14093=CARTESIAN_POINT ( 'NONE',  ( -3.898383833589191827, 13.39623302270000771, -56.99295307432605995 ) ) ;
#14108=CARTESIAN_POINT ( 'NONE',  ( 5.588711115410763597, 18.38516488214980882, -30.29999999999996518 ) ) ;
#14111=CARTESIAN_POINT ( 'NONE',  ( -3.965139115708213868, 15.65104167704456906, -54.15704692567387468 ) ) ;
#14112=CARTESIAN_POINT ( 'NONE',  ( -1.887862790868997553, 21.20513934631180319, -71.39999999999996305 ) ) ;
#14118=CARTESIAN_POINT ( 'NONE',  ( 0.6505131845895220088, 21.60717860451803674, -56.69999999999997442 ) ) ;
#14120=CARTESIAN_POINT ( 'NONE',  ( 0.7939530028709752552, 21.58445996917927445, -40.20704692567387184 ) ) ;
#14130=CARTESIAN_POINT ( 'NONE',  ( -3.965139115708213868, 15.65104167704456906, -27.15704692567387823 ) ) ;
#14136=CARTESIAN_POINT ( 'NONE',  ( 0.9307174358028528216, 11.62368137996505801, -43.04999999999996163 ) ) ;
#14152=CARTESIAN_POINT ( 'NONE',  ( 0.8851648821498760977, 23.08871111541074228, -59.69999999999996732 ) ) ;
#14157=CARTESIAN_POINT ( 'NONE',  ( -4.318543150850367773, 18.18399003996480801, -34.94999999999996732 ) ) ;
#14158=CARTESIAN_POINT ( 'NONE',  ( -4.318543150850366885, 18.18399003996480801, -67.94999999999996021 ) ) ;
#14168=CARTESIAN_POINT ( 'NONE',  ( -3.826489000663265472, 15.37892550466785480, -45.14295307432605853 ) ) ;
#14174=CARTESIAN_POINT ( 'NONE',  ( 2.837723661809363307, 20.54310680552015356, -67.49295307432606705 ) ) ;
#14195=CARTESIAN_POINT ( 'NONE',  ( 0.8851648821498760977, 23.08871111541074228, -65.69999999999996021 ) ) ;
#14213=CARTESIAN_POINT ( 'NONE',  ( 3.898383833589191383, 21.60376697729997275, -55.49295307432605995 ) ) ;
#14223=CARTESIAN_POINT ( 'NONE',  ( 4.342430937695320736, 16.96683151040971538, -70.94295307432606990 ) ) ;
#14225=CARTESIAN_POINT ( 'NONE',  ( 0.5331684895902240040, 13.15756906230466328, -65.55704692567385905 ) ) ;
#14239=CARTESIAN_POINT ( 'NONE',  ( -1.887862790868997553, 21.20513934631180319, -56.39999999999996305 ) ) ;
#14252=CARTESIAN_POINT ( 'NONE',  ( 3.771071394011080269, 15.74153613859503764, -71.09295307432604716 ) ) ;
#14271=CARTESIAN_POINT ( 'NONE',  ( -1.985016409143819605, 13.60418594181426855, -46.34999999999997300 ) ) ;
#14281=CARTESIAN_POINT ( 'NONE',  ( -2.940415233664778860, 14.55958476633523802, -67.49999999999995737 ) ) ;
#14284=CARTESIAN_POINT ( 'NONE',  ( -5.370428668309080500, 14.93501088608579153, -57.15704692567387468 ) ) ;
#14285=CARTESIAN_POINT ( 'NONE',  ( -0.9307174358028534877, 23.37631862003491889, -47.54999999999996874 ) ) ;
#14299=CARTESIAN_POINT ( 'NONE',  ( 4.975717084895059372, 14.80175253005754143, -35.10704692567387752 ) ) ;
#14301=CARTESIAN_POINT ( 'NONE',  ( -0.7417250638684240727, 11.88857024925047057, -53.69295307432606279 ) ) ;
#14318=CARTESIAN_POINT ( 'NONE',  ( 5.876318620034919782, 16.56928256419707068, -30.44999999999995310 ) ) ;
#14321=CARTESIAN_POINT ( 'NONE',  ( -3.639207298612509689, 19.51726172033310647, -45.60704692567387752 ) ) ;
#14322=CARTESIAN_POINT ( 'NONE',  ( -3.705139346311794313, 19.38786279086902198, -71.09999999999996589 ) ) ;
#14329=CARTESIAN_POINT ( 'NONE',  ( -2.940415233664778860, 14.55958476633523802, -58.49999999999997158 ) ) ;
#14332=CARTESIAN_POINT ( 'NONE',  ( -3.965139115708213868, 15.65104167704456906, -39.15704692567386758 ) ) ;
#14333=CARTESIAN_POINT ( 'NONE',  ( 0.8851648821498760977, 23.08871111541074228, -74.69999999999997442 ) ) ;
#14344=CARTESIAN_POINT ( 'NONE',  ( 5.852430833189966819, 16.41846101382252243, -67.95704692567387895 ) ) ;
#14349=CARTESIAN_POINT ( 'NONE',  ( -0.9307174358028533767, 23.37631862003491889, -29.54999999999996518 ) ) ;
#14366=CARTESIAN_POINT ( 'NONE',  ( 5.301103610786608300, 20.20104720010253985, -63.14999999999997016 ) ) ;
#14370=CARTESIAN_POINT ( 'NONE',  ( 1.985016409143818272, 21.39581405818570303, -32.84999999999996589 ) ) ;
#14371=CARTESIAN_POINT ( 'NONE',  ( 0.6505131845895220088, 21.60717860451803674, -65.69999999999996021 ) ) ;
#14382=CARTESIAN_POINT ( 'NONE',  ( -3.771071394011080269, 19.25846386140493394, -36.59295307432605426 ) ) ;
#14387=CARTESIAN_POINT ( 'NONE',  ( 1.848958322955461808, 21.46513911570817612, -52.34295307432604716 ) ) ;
#14404=CARTESIAN_POINT ( 'NONE',  ( -2.568848540478311904, 22.54164913259435465, -65.39999999999997726 ) ) ;
#14426=CARTESIAN_POINT ( 'NONE',  ( -2.698247469942396837, 22.47571708489507358, -54.89295307432605853 ) ) ;
#14436=CARTESIAN_POINT ( 'NONE',  ( 1.848958322955461808, 21.46513911570817612, -61.34295307432606137 ) ) ;
#14438=CARTESIAN_POINT ( 'NONE',  ( 2.121074495332174958, 21.32648900066323350, -58.35704692567387752 ) ) ;
#14450=CARTESIAN_POINT ( 'NONE',  ( 1.887862790868997109, 13.79486065368817194, -51.89999999999997016 ) ) ;
#14463=CARTESIAN_POINT ( 'NONE',  ( -2.017261720333081598, 21.13920729861251857, -75.89295307432605853 ) ) ;
#14478=CARTESIAN_POINT ( 'NONE',  ( 3.091735541773220852, 14.40826445822673740, -39.74999999999996447 ) ) ;
#14484=CARTESIAN_POINT ( 'NONE',  ( 0.6839900399647733664, 13.18145684914961357, -31.04999999999995808 ) ) ;
#14494=CARTESIAN_POINT ( 'NONE',  ( -2.940415233664778860, 14.55958476633523802, -61.49999999999997158 ) ) ;
#14496=CARTESIAN_POINT ( 'NONE',  ( 4.099003336600150149, 13.18504404629255689, -53.25704692567386900 ) ) ;
#14497=CARTESIAN_POINT ( 'NONE',  ( -4.001075405444606936, 13.49892459455542060, -34.49999999999997158 ) ) ;
#14510=CARTESIAN_POINT ( 'NONE',  ( -1.028604700431329233, 11.93400751992799513, -38.70704692567387184 ) ) ;
#14515=CARTESIAN_POINT ( 'NONE',  ( -5.107581180293630396, 19.93944961101426827, -51.59295307432605426 ) ) ;
#14533=CARTESIAN_POINT ( 'NONE',  ( -5.900206406879871857, 18.27989588542834554, -75.44295307432606990 ) ) ;
#14536=CARTESIAN_POINT ( 'NONE',  ( -2.121074495332175847, 13.67351099933674341, -41.85704692567387752 ) ) ;
#14545=CARTESIAN_POINT ( 'NONE',  ( 3.091735541773220852, 14.40826445822673563, -48.74999999999997158 ) ) ;
#14548=CARTESIAN_POINT ( 'NONE',  ( -2.983759233219601903, 20.69971185032686023, -39.75704692567386900 ) ) ;
#14549=CARTESIAN_POINT ( 'NONE',  ( -5.301103610786608300, 14.79895279989743528, -70.64999999999996305 ) ) ;
#14559=CARTESIAN_POINT ( 'NONE',  ( -4.975717084895059372, 20.19824746994243370, -66.60704692567387042 ) ) ;
#14563=CARTESIAN_POINT ( 'NONE',  ( -5.588711115410763597, 16.61483511785016987, -28.79999999999996518 ) ) ;
#14581=CARTESIAN_POINT ( 'NONE',  ( 2.568848540478311460, 12.45835086740561692, -51.89999999999997016 ) ) ;
#14585=CARTESIAN_POINT ( 'NONE',  ( -3.091735541773221296, 20.59173554177323950, -26.24999999999996803 ) ) ;
#14586=CARTESIAN_POINT ( 'NONE',  ( 3.091735541773220852, 14.40826445822673740, -63.74999999999997158 ) ) ;
#14592=CARTESIAN_POINT ( 'NONE',  ( 4.318543150850367773, 16.81600996003516357, -69.44999999999997442 ) ) ;
#14596=CARTESIAN_POINT ( 'NONE',  ( 3.771071394011080269, 15.74153613859503764, -38.09295307432605426 ) ) ;
#14599=CARTESIAN_POINT ( 'NONE',  ( 3.826489000663266360, 19.62107449533211678, -52.64295307432606563 ) ) ;
#14617=CARTESIAN_POINT ( 'NONE',  ( -5.041649132594344884, 20.06884854047834921, -53.09999999999996589 ) ) ;
#14640=CARTESIAN_POINT ( 'NONE',  ( 5.231778553264135212, 20.33710528629089254, -52.64295307432606563 ) ) ;
#14650=CARTESIAN_POINT ( 'NONE',  ( 2.837723661809363307, 20.54310680552015356, -67.49295307432606705 ) ) ;
#14652=CARTESIAN_POINT ( 'NONE',  ( 0.7939530028709752552, 21.58445996917927445, -58.20704692567387184 ) ) ;
#14664=CARTESIAN_POINT ( 'NONE',  ( 4.107178604518054499, 18.15051318458946383, -45.29999999999996874 ) ) ;
#14675=CARTESIAN_POINT ( 'NONE',  ( 3.199711850326839357, 14.51624076678035635, -71.24295307432605284 ) ) ;
#14689=CARTESIAN_POINT ( 'NONE',  ( -3.091735541773221296, 20.59173554177323950, -41.24999999999995737 ) ) ;
#14694=CARTESIAN_POINT ( 'NONE',  ( -0.6839900399647736995, 21.81854315085035623, -38.54999999999996874 ) ) ;
#14703=CARTESIAN_POINT ( 'NONE',  ( -0.6505131845895224529, 13.39282139548194195, -52.19999999999996732 ) ) ;
#14705=CARTESIAN_POINT ( 'NONE',  ( -4.103766977300021601, 13.60161616641083704, -45.00704692567388321 ) ) ;
#14706=CARTESIAN_POINT ( 'NONE',  ( -5.876318620034919782, 18.43071743580290089, -40.94999999999996732 ) ) ;
#14709=CARTESIAN_POINT ( 'NONE',  ( 1.985016409143818272, 21.39581405818570303, -71.84999999999998010 ) ) ;
#14720=CARTESIAN_POINT ( 'NONE',  ( 5.611429750749524992, 18.24172506386835479, -34.80704692567387326 ) ) ;
#14725=CARTESIAN_POINT ( 'NONE',  ( 0.7417250638684235176, 23.11142975074950101, -55.19295307432606279 ) ) ;
#14742=CARTESIAN_POINT ( 'NONE',  ( -5.041649132594344884, 20.06884854047834921, -26.09999999999996234 ) ) ;
#14745=CARTESIAN_POINT ( 'NONE',  ( 3.639207298612508801, 15.48273827966686866, -41.10704692567387752 ) ) ;
#14746=CARTESIAN_POINT ( 'NONE',  ( -3.705139346311794313, 19.38786279086902198, -35.09999999999996589 ) ) ;
#14747=CARTESIAN_POINT ( 'NONE',  ( -3.091735541773221296, 20.59173554177323950, -68.24999999999995737 ) ) ;
#14758=CARTESIAN_POINT ( 'NONE',  ( 1.758463861404912620, 13.72892860598888731, -26.40704692567387823 ) ) ;
#14759=CARTESIAN_POINT ( 'NONE',  ( 5.876318620034919782, 16.56928256419707068, -69.44999999999998863 ) ) ;
#14768=CARTESIAN_POINT ( 'NONE',  ( -0.7798958854283041253, 23.40020640687986386, -61.05704692567386616 ) ) ;
#14772=CARTESIAN_POINT ( 'NONE',  ( -5.876318620034919782, 18.43071743580290089, -25.94999999999996732 ) ) ;
#14786=CARTESIAN_POINT ( 'NONE',  ( 5.301103610786608300, 20.20104720010253985, -51.14999999999994884 ) ) ;
#14790=CARTESIAN_POINT ( 'NONE',  ( -0.6839900399647736995, 21.81854315085035623, -26.54999999999996163 ) ) ;
#14791=CARTESIAN_POINT ( 'NONE',  ( -2.940415233664778860, 14.55958476633523802, -58.49999999999997158 ) ) ;
#14802=CARTESIAN_POINT ( 'NONE',  ( -1.848958322955462474, 13.53486088429179546, -35.84295307432606137 ) ) ;
#14805=CARTESIAN_POINT ( 'NONE',  ( -3.199711850326840246, 20.48375923321962233, -51.74295307432605995 ) ) ;
#14820=CARTESIAN_POINT ( 'NONE',  ( -0.8851648821498765418, 11.91128888458923285, -61.19999999999996732 ) ) ;
#14840=CARTESIAN_POINT ( 'NONE',  ( 3.898383833589191383, 21.60376697729997275, -52.49295307432605995 ) ) ;
#14848=CARTESIAN_POINT ( 'NONE',  ( -4.084459969179292216, 16.70604699712905372, -63.29295307432605000 ) ) ;
#14864=CARTESIAN_POINT ( 'NONE',  ( -1.985016409143819605, 13.60418594181426855, -49.34999999999996589 ) ) ;
#14874=CARTESIAN_POINT ( 'NONE',  ( -4.342430937695320736, 18.03316848959025620, -69.44295307432605568 ) ) ;
#14885=CARTESIAN_POINT ( 'NONE',  ( -1.985016409143819605, 13.60418594181426855, -34.34999999999996589 ) ) ;
#14889=CARTESIAN_POINT ( 'NONE',  ( 3.091735541773220852, 14.40826445822673563, -36.74999999999994316 ) ) ;
#14897=CARTESIAN_POINT ( 'NONE',  ( -1.985016409143819605, 13.60418594181426855, -55.34999999999997300 ) ) ;
#14899=CARTESIAN_POINT ( 'NONE',  ( -2.439449611014227859, 22.60758118029364283, -48.90704692567388179 ) ) ;
#14900=CARTESIAN_POINT ( 'NONE',  ( 5.588711115410763597, 18.38516488214980882, -39.29999999999996874 ) ) ;
#14903=CARTESIAN_POINT ( 'NONE',  ( -3.091735541773221296, 20.59173554177323950, -74.24999999999997158 ) ) ;
#14915=CARTESIAN_POINT ( 'NONE',  ( 4.103766977300021601, 21.39838383358913987, -31.50704692567387610 ) ) ;
#14922=CARTESIAN_POINT ( 'NONE',  ( 2.698247469942395949, 12.52428291510489977, -50.39295307432605853 ) ) ;
#14939=CARTESIAN_POINT ( 'NONE',  ( 5.588711115410763597, 18.38516488214980882, -27.29999999999996163 ) ) ;
#14943=CARTESIAN_POINT ( 'NONE',  ( -3.965139115708213868, 15.65104167704456906, -45.15704692567388179 ) ) ;
#14945=CARTESIAN_POINT ( 'NONE',  ( -2.940415233664778860, 14.55958476633523802, -31.49999999999996447 ) ) ;
#14946=CARTESIAN_POINT ( 'NONE',  ( 4.107178604518054499, 18.15051318458946383, -63.29999999999996874 ) ) ;
#14957=CARTESIAN_POINT ( 'NONE',  ( -2.983759233219601903, 20.69971185032686023, -24.75704692567387610 ) ) ;
#14958=CARTESIAN_POINT ( 'NONE',  ( 0.9307174358028527106, 11.62368137996505801, -61.04999999999996163 ) ) ;
#14969=CARTESIAN_POINT ( 'NONE',  ( 2.837105286290961370, 22.73177855326409613, -67.35704692567388463 ) ) ;
#14975=CARTESIAN_POINT ( 'NONE',  ( -5.588711115410763597, 16.61483511785016987, -25.79999999999996163 ) ) ;
#14991=CARTESIAN_POINT ( 'NONE',  ( -5.588711115410763597, 16.61483511785016987, -49.79999999999996874 ) ) ;
#14995=CARTESIAN_POINT ( 'NONE',  ( -3.895814058185739448, 15.51498359085620571, -25.64999999999996305 ) ) ;
#14996=CARTESIAN_POINT ( 'NONE',  ( 4.107178604518054499, 18.15051318458946383, -54.29999999999996874 ) ) ;
#15004=CARTESIAN_POINT ( 'NONE',  ( 3.705139346311793869, 15.61213720913094960, -72.59999999999996589 ) ) ;
#15008=CARTESIAN_POINT ( 'NONE',  ( -2.017261720333081598, 21.13920729861251857, -33.89295307432605142 ) ) ;
#15011=CARTESIAN_POINT ( 'NONE',  ( -2.017261720333081598, 21.13920729861251857, -54.89295307432605853 ) ) ;
#15027=CARTESIAN_POINT ( 'NONE',  ( 5.301103610786608300, 20.20104720010253985, -60.14999999999995595 ) ) ;
#15051=CARTESIAN_POINT ( 'NONE',  ( 5.565992480072003978, 18.52860470043125574, -46.79295307432605711 ) ) ;
#15059=CARTESIAN_POINT ( 'NONE',  ( 3.826489000663266360, 19.62107449533211678, -64.64295307432604432 ) ) ;
#15073=CARTESIAN_POINT ( 'NONE',  ( -3.705139346311794313, 19.38786279086902198, -47.09999999999996589 ) ) ;
#15076=CIRCLE ( 'NONE', #31366, 0.7500000000000012212 ) ;
#15100=CARTESIAN_POINT ( 'NONE',  ( 1.985016409143818272, 21.39581405818570659, -38.84999999999996589 ) ) ;
#15104=CARTESIAN_POINT ( 'NONE',  ( 0.6505131845895220088, 21.60717860451803674, -32.69999999999996732 ) ) ;
#15113=CARTESIAN_POINT ( 'NONE',  ( 4.107178604518054499, 18.15051318458946383, -54.29999999999996874 ) ) ;
#15115=CARTESIAN_POINT ( 'NONE',  ( -5.852430833189966819, 18.58153898617744915, -51.45704692567387895 ) ) ;
#15116=CARTESIAN_POINT ( 'NONE',  ( 5.876318620034919782, 16.56928256419707068, -33.44999999999996021 ) ) ;
#15119=CARTESIAN_POINT ( 'NONE',  ( 1.985016409143818272, 21.39581405818570303, -74.84999999999993747 ) ) ;
#15127=CARTESIAN_POINT ( 'NONE',  ( -5.900206406879871857, 18.27989588542834554, -39.44295307432604858 ) ) ;
#15130=CARTESIAN_POINT ( 'NONE',  ( 4.975717084895059372, 14.80175253005754143, -26.10704692567387397 ) ) ;
#15134=CARTESIAN_POINT ( 'NONE',  ( -0.7417250638684240727, 11.88857024925047057, -50.69295307432606279 ) ) ;
#15151=CARTESIAN_POINT ( 'NONE',  ( -5.301103610786608300, 14.79895279989743706, -25.64999999999996305 ) ) ;
#15155=CARTESIAN_POINT ( 'NONE',  ( 0.7939530028709752552, 21.58445996917927445, -43.20704692567387184 ) ) ;
#15156=CARTESIAN_POINT ( 'NONE',  ( -4.318543150850367773, 18.18399003996480801, -37.94999999999996021 ) ) ;
#15157=CARTESIAN_POINT ( 'NONE',  ( 3.895814058185739448, 19.48501640914375344, -63.14999999999997016 ) ) ;
#15167=CARTESIAN_POINT ( 'NONE',  ( -0.7939530028709754772, 13.41554003082070246, -26.70704692567387539 ) ) ;
#15168=CARTESIAN_POINT ( 'NONE',  ( -4.001075405444606936, 13.49892459455542060, -67.49999999999995737 ) ) ;
#15179=CARTESIAN_POINT ( 'NONE',  ( 5.611429750749524992, 18.24172506386835479, -61.80704692567387326 ) ) ;
#15184=CARTESIAN_POINT ( 'NONE',  ( 5.876318620034919782, 16.56928256419707068, -27.44999999999996021 ) ) ;
#15202=CARTESIAN_POINT ( 'NONE',  ( 5.301103610786608300, 20.20104720010253985, -48.14999999999997726 ) ) ;
#15206=CARTESIAN_POINT ( 'NONE',  ( -4.107178604518053611, 16.84948681541050775, -28.79999999999996518 ) ) ;
#15207=CARTESIAN_POINT ( 'NONE',  ( 0.6505131845895220088, 21.60717860451803674, -59.69999999999996732 ) ) ;
#15220=CARTESIAN_POINT ( 'NONE',  ( 3.771071394011080269, 15.74153613859503764, -35.09295307432605426 ) ) ;
#15223=CARTESIAN_POINT ( 'NONE',  ( -3.826489000663265472, 15.37892550466785480, -57.14295307432605142 ) ) ;
#15242=CARTESIAN_POINT ( 'NONE',  ( 2.701047200102605572, 22.80110361078655856, -53.84999999999995879 ) ) ;
#15265=CARTESIAN_POINT ( 'NONE',  ( 0.7417250638684235176, 23.11142975074950101, -43.19295307432606279 ) ) ;
#15273=CARTESIAN_POINT ( 'NONE',  ( -0.5070733663080690956, 13.37010276014318144, -65.69295307432605568 ) ) ;
#15291=CARTESIAN_POINT ( 'NONE',  ( 0.6839900399647733664, 13.18145684914961357, -49.04999999999994742 ) ) ;
#15317=CARTESIAN_POINT ( 'NONE',  ( 0.6505131845895220088, 21.60717860451803674, -32.69999999999996732 ) ) ;
#15322=CARTESIAN_POINT ( 'NONE',  ( 1.985016409143818272, 21.39581405818570303, -38.84999999999996589 ) ) ;
#15331=CARTESIAN_POINT ( 'NONE',  ( 0.6505131845895220088, 21.60717860451803674, -59.69999999999996732 ) ) ;
#15333=CARTESIAN_POINT ( 'NONE',  ( 5.852430833189966819, 16.41846101382252243, -46.95704692567387184 ) ) ;
#15334=CARTESIAN_POINT ( 'NONE',  ( 5.301103610786608300, 20.20104720010254340, -36.14999999999996305 ) ) ;
#15336=CARTESIAN_POINT ( 'NONE',  ( 3.091735541773220852, 14.40826445822673563, -69.74999999999997158 ) ) ;
#15352=CARTESIAN_POINT ( 'NONE',  ( -4.975717084895059372, 20.19824746994243370, -27.60704692567387397 ) ) ;
#15356=CARTESIAN_POINT ( 'NONE',  ( -3.898383833589191827, 13.39623302270000771, -41.99295307432605995 ) ) ;
#15374=( NAMED_UNIT ( * ) PLANE_ANGLE_UNIT ( ) SI_UNIT ( $, .RADIAN. ) );
#15375=CARTESIAN_POINT ( 'NONE',  ( 5.876318620034919782, 16.56928256419707068, -27.44999999999996021 ) ) ;
#15380=CARTESIAN_POINT ( 'NONE',  ( -4.107178604518053611, 16.84948681541050775, -34.79999999999996163 ) ) ;
#15381=CARTESIAN_POINT ( 'NONE',  ( -4.318543150850367773, 18.18399003996480801, -61.94999999999997442 ) ) ;
#15389=CARTESIAN_POINT ( 'NONE',  ( -0.7939530028709754772, 13.41554003082070246, -29.70704692567387184 ) ) ;
#15390=CARTESIAN_POINT ( 'NONE',  ( 0.8851648821498760977, 23.08871111541074228, -65.69999999999996021 ) ) ;
#15401=CARTESIAN_POINT ( 'NONE',  ( -5.852430833189966819, 18.58153898617744915, -54.45704692567387895 ) ) ;
#15404=CARTESIAN_POINT ( 'NONE',  ( -4.314955953707389824, 21.59900333660018390, -66.74295307432606705 ) ) ;
#15419=CARTESIAN_POINT ( 'NONE',  ( -5.041649132594344884, 20.06884854047834921, -50.09999999999996589 ) ) ;
#15423=CARTESIAN_POINT ( 'NONE',  ( -3.965139115708213868, 15.65104167704456906, -69.15704692567386758 ) ) ;
#15424=CARTESIAN_POINT ( 'NONE',  ( 3.091735541773220852, 14.40826445822673740, -60.74999999999996447 ) ) ;
#15430=CARTESIAN_POINT ( 'NONE',  ( -1.985016409143819605, 13.60418594181426855, -73.34999999999996589 ) ) ;
#15432=CARTESIAN_POINT ( 'NONE',  ( -0.5331684895902242260, 21.84243093769531185, -58.05704692567386616 ) ) ;
#15436=CARTESIAN_POINT ( 'NONE',  ( -0.6839900399647736995, 21.81854315085035623, -71.54999999999994031 ) ) ;
#15439=CARTESIAN_POINT ( 'NONE',  ( 3.771071394011080269, 15.74153613859503764, -44.09295307432605426 ) ) ;
#15453=CARTESIAN_POINT ( 'NONE',  ( 0.9307174358028528216, 11.62368137996505801, -61.04999999999995453 ) ) ;
#15460=CARTESIAN_POINT ( 'NONE',  ( 4.001075405444606048, 21.50107540544455276, -74.99999999999997158 ) ) ;
#15474=CARTESIAN_POINT ( 'NONE',  ( 1.081538986177402295, 11.64756916681001186, -41.54295307432605000 ) ) ;
#15483=CARTESIAN_POINT ( 'NONE',  ( -0.8348115903393239501, 21.79465536400541126, -58.04295307432605711 ) ) ;
#15499=CARTESIAN_POINT ( 'NONE',  ( -1.887862790868997553, 21.20513934631180319, -47.39999999999997016 ) ) ;
#15520=CARTESIAN_POINT ( 'NONE',  ( 4.107178604518054499, 18.15051318458946383, -33.29999999999996874 ) ) ;
#15526=CARTESIAN_POINT ( 'NONE',  ( 4.294655364005415699, 16.66518840966061887, -70.95704692567389316 ) ) ;
#15535=CARTESIAN_POINT ( 'NONE',  ( 1.985016409143818272, 21.39581405818570303, -59.84999999999996589 ) ) ;
#15538=CARTESIAN_POINT ( 'NONE',  ( -1.028604700431329233, 11.93400751992799513, -50.70704692567387184 ) ) ;
#15540=CARTESIAN_POINT ( 'NONE',  ( 3.771071394011080269, 15.74153613859503764, -29.09295307432605782 ) ) ;
#15551=CARTESIAN_POINT ( 'NONE',  ( -0.9307174358028533767, 23.37631862003491889, -74.54999999999994031 ) ) ;
#15557=CARTESIAN_POINT ( 'NONE',  ( 4.314955953707388936, 13.40099666339979123, -44.24295307432605995 ) ) ;
#15572=CARTESIAN_POINT ( 'NONE',  ( 5.107581180293630396, 15.06055038898570686, -65.09295307432604716 ) ) ;
#15577=CARTESIAN_POINT ( 'NONE',  ( -3.895814058185739448, 15.51498359085620571, -37.64999999999996305 ) ) ;
#15578=CARTESIAN_POINT ( 'NONE',  ( -0.6839900399647736995, 21.81854315085035623, -62.54999999999996874 ) ) ;
#15591=CARTESIAN_POINT ( 'NONE',  ( -2.983759233219601903, 20.69971185032686023, -27.75704692567387255 ) ) ;
#15592=CARTESIAN_POINT ( 'NONE',  ( 5.876318620034919782, 16.56928256419707068, -66.44999999999997442 ) ) ;
#15603=CARTESIAN_POINT ( 'NONE',  ( 4.975717084895059372, 14.80175253005754143, -56.10704692567387752 ) ) ;
#15607=CARTESIAN_POINT ( 'NONE',  ( 2.698247469942395949, 12.52428291510489977, -68.39295307432607274 ) ) ;
#15626=CARTESIAN_POINT ( 'NONE',  ( 4.206979645153767322, 13.29302035484617051, -39.74999999999996447 ) ) ;
#15631=CARTESIAN_POINT ( 'NONE',  ( -0.5331684895902242260, 21.84243093769531185, -67.05704692567387326 ) ) ;
#15632=CARTESIAN_POINT ( 'NONE',  ( 0.6839900399647732554, 13.18145684914961357, -61.04999999999996163 ) ) ;
#15639=CARTESIAN_POINT ( 'NONE',  ( -1.985016409143819605, 13.60418594181426855, -67.34999999999996589 ) ) ;
#15641=CARTESIAN_POINT ( 'NONE',  ( 3.043106805520193525, 20.33772366180932067, -58.50704692567387610 ) ) ;
#15643=CARTESIAN_POINT ( 'NONE',  ( -1.985016409143819605, 13.60418594181426855, -70.34999999999993747 ) ) ;
#15647=CARTESIAN_POINT ( 'NONE',  ( -3.771071394011080269, 19.25846386140493394, -42.59295307432605426 ) ) ;
#15663=CARTESIAN_POINT ( 'NONE',  ( -0.8851648821498765418, 11.91128888458923285, -52.19999999999996732 ) ) ;
#15682=CARTESIAN_POINT ( 'NONE',  ( 1.887862790868997109, 13.79486065368817194, -39.89999999999996305 ) ) ;
#15683=CARTESIAN_POINT ( 'NONE',  ( -2.698247469942396837, 22.47571708489507358, -42.89295307432605853 ) ) ;
#15693=CARTESIAN_POINT ( 'NONE',  ( 4.084459969179292216, 18.29395300287091430, -58.79295307432606421 ) ) ;
#15707=CARTESIAN_POINT ( 'NONE',  ( -3.705139346311794313, 19.38786279086902198, -38.09999999999996589 ) ) ;
#15731=CARTESIAN_POINT ( 'NONE',  ( -3.895814058185739892, 15.51498359085620748, -25.64999999999996305 ) ) ;
#15734=CARTESIAN_POINT ( 'NONE',  ( 5.900206406879871857, 16.72010411457162604, -37.94295307432606279 ) ) ;
#15736=CARTESIAN_POINT ( 'NONE',  ( 1.758463861404912620, 13.72892860598888731, -71.40704692567388179 ) ) ;
#15745=CARTESIAN_POINT ( 'NONE',  ( 1.887862790868997109, 13.79486065368817194, -48.89999999999997016 ) ) ;
#15748=CARTESIAN_POINT ( 'NONE',  ( 5.370428668309080500, 20.06498911391418360, -34.65704692567386758 ) ) ;
#15749=CARTESIAN_POINT ( 'NONE',  ( 2.701047200102605128, 22.80110361078656211, -26.84999999999996234 ) ) ;
#15750=CARTESIAN_POINT ( 'NONE',  ( -1.887862790868997553, 21.20513934631180319, -62.39999999999997016 ) ) ;
#15760=CARTESIAN_POINT ( 'NONE',  ( 5.041649132594343996, 14.93115145952162415, -72.59999999999996589 ) ) ;
#15765=CARTESIAN_POINT ( 'NONE',  ( 5.565992480072003978, 18.52860470043125574, -40.79295307432605711 ) ) ;
#15784=CARTESIAN_POINT ( 'NONE',  ( -3.898383833589191827, 13.39623302270000771, -65.99295307432606705 ) ) ;
#15790=CARTESIAN_POINT ( 'NONE',  ( 2.940415233664778416, 20.44041523366473712, -29.99999999999996447 ) ) ;
#15792=CARTESIAN_POINT ( 'NONE',  ( -3.705139346311794313, 19.38786279086902198, -56.09999999999996589 ) ) ;
#15803=CARTESIAN_POINT ( 'NONE',  ( 5.852430833189966819, 16.41846101382252243, -61.95704692567387895 ) ) ;
#15804=CARTESIAN_POINT ( 'NONE',  ( 5.301103610786608300, 20.20104720010254340, -54.14999999999997016 ) ) ;
#15818=CARTESIAN_POINT ( 'NONE',  ( -5.370428668309080500, 14.93501088608579153, -51.15704692567387468 ) ) ;
#15822=CARTESIAN_POINT ( 'NONE',  ( -5.231778553264134324, 14.66289471370907727, -72.14295307432605853 ) ) ;
#15841=CARTESIAN_POINT ( 'NONE',  ( -5.876318620034919782, 18.43071743580290089, -43.94999999999995310 ) ) ;
#15845=CARTESIAN_POINT ( 'NONE',  ( -2.983759233219601903, 20.69971185032686023, -63.75704692567388321 ) ) ;
#15846=CARTESIAN_POINT ( 'NONE',  ( -3.705139346311794313, 19.38786279086902198, -50.09999999999996589 ) ) ;
#15855=CARTESIAN_POINT ( 'NONE',  ( 3.705139346311793869, 15.61213720913094960, -63.59999999999995879 ) ) ;
#15858=CARTESIAN_POINT ( 'NONE',  ( -4.129897239856814117, 16.99292663369196177, -51.30704692567388037 ) ) ;
#15861=CARTESIAN_POINT ( 'NONE',  ( 3.091735541773220852, 14.40826445822673563, -72.74999999999995737 ) ) ;
#15864=CARTESIAN_POINT ( 'NONE',  ( 3.826489000663266360, 19.62107449533211678, -46.64295307432605853 ) ) ;
#15879=CARTESIAN_POINT ( 'NONE',  ( 2.701047200102605572, 22.80110361078655856, -50.84999999999997300 ) ) ;
#15886=PLANE ( 'NONE',  #25324 ) ;
#15896=CARTESIAN_POINT ( 'NONE',  ( 5.876318620034919782, 16.56928256419707068, -72.44999999999994600 ) ) ;
#15901=CARTESIAN_POINT ( 'NONE',  ( -3.705139346311794313, 19.38786279086902198, -44.09999999999996589 ) ) ;
#15909=CARTESIAN_POINT ( 'NONE',  ( 0.8348115903393232839, 13.20534463599456387, -56.54295307432606421 ) ) ;
#15925=CARTESIAN_POINT ( 'NONE',  ( 3.705139346311793869, 15.61213720913094960, -39.59999999999996589 ) ) ;
#15951=CARTESIAN_POINT ( 'NONE',  ( -4.294655364005415699, 18.33481159033935626, -30.45704692567387184 ) ) ;
#15952=CARTESIAN_POINT ( 'NONE',  ( -3.705139346311794313, 19.38786279086902198, -29.09999999999996589 ) ) ;
#15955=CARTESIAN_POINT ( 'NONE',  ( -4.314955953707389824, 21.59900333660018390, -30.74295307432605640 ) ) ;
#15956=CARTESIAN_POINT ( 'NONE',  ( -3.705139346311794313, 19.38786279086902198, -29.09999999999996589 ) ) ;
#15963=CARTESIAN_POINT ( 'NONE',  ( -0.6839900399647736995, 21.81854315085035623, -47.54999999999997584 ) ) ;
#15966=CARTESIAN_POINT ( 'NONE',  ( 1.028604700431328567, 23.06599248007198355, -37.20704692567387184 ) ) ;
#15967=CARTESIAN_POINT ( 'NONE',  ( -2.568848540478311904, 22.54164913259435465, -26.39999999999996660 ) ) ;
#15969=CARTESIAN_POINT ( 'NONE',  ( 3.895814058185739448, 19.48501640914375344, -66.14999999999997726 ) ) ;
#15979=CARTESIAN_POINT ( 'NONE',  ( -5.852430833189966819, 18.58153898617744915, -24.45704692567386829 ) ) ;
#15987=CARTESIAN_POINT ( 'NONE',  ( -5.900206406879871857, 18.27989588542834554, -39.44295307432604858 ) ) ;
#16002=CARTESIAN_POINT ( 'NONE',  ( 1.081538986177402295, 11.64756916681001186, -62.54295307432605711 ) ) ;
#16008=CARTESIAN_POINT ( 'NONE',  ( -2.940415233664778860, 14.55958476633523802, -52.49999999999996447 ) ) ;
#16020=CARTESIAN_POINT ( 'NONE',  ( -2.439449611014227859, 22.60758118029364283, -69.90704692567388179 ) ) ;
#16021=CARTESIAN_POINT ( 'NONE',  ( 5.041649132594343996, 14.93115145952162415, -57.59999999999997300 ) ) ;
#16035=CARTESIAN_POINT ( 'NONE',  ( -4.099003336600151925, 21.81495595370741469, -54.75704692567386900 ) ) ;
#16038=CARTESIAN_POINT ( 'NONE',  ( 2.564989113914249330, 22.87042866830903876, -70.34295307432606137 ) ) ;
#16054=CARTESIAN_POINT ( 'NONE',  ( -0.8851648821498765418, 11.91128888458923285, -46.19999999999996021 ) ) ;
#16060=CARTESIAN_POINT ( 'NONE',  ( 1.758463861404912620, 13.72892860598888731, -59.40704692567388179 ) ) ;
#16061=CARTESIAN_POINT ( 'NONE',  ( 1.887862790868997109, 13.79486065368817194, -51.89999999999997016 ) ) ;
#16070=CARTESIAN_POINT ( 'NONE',  ( 1.887862790868997109, 13.79486065368817194, -66.89999999999997726 ) ) ;
#16072=CARTESIAN_POINT ( 'NONE',  ( 4.129897239856814117, 18.00707336630801336, -46.80704692567388037 ) ) ;
#16078=CARTESIAN_POINT ( 'NONE',  ( 3.771071394011080269, 15.74153613859503764, -47.09295307432606137 ) ) ;
#16094=CARTESIAN_POINT ( 'NONE',  ( 5.588711115410763597, 18.38516488214980882, -45.29999999999996874 ) ) ;
#16107=CARTESIAN_POINT ( 'NONE',  ( -2.568848540478311904, 22.54164913259435465, -68.39999999999997726 ) ) ;
#16113=CARTESIAN_POINT ( 'NONE',  ( 3.091735541773220852, 14.40826445822673563, -42.74999999999996447 ) ) ;
#16125=CARTESIAN_POINT ( 'NONE',  ( -4.342430937695320736, 18.03316848959025620, -57.44295307432606990 ) ) ;
#16141=CARTESIAN_POINT ( 'NONE',  ( 0.6839900399647733664, 13.18145684914961357, -34.04999999999995453 ) ) ;
#16163=CARTESIAN_POINT ( 'NONE',  ( 3.043106805520193525, 20.33772366180932067, -37.50704692567386189 ) ) ;
#16164=CARTESIAN_POINT ( 'NONE',  ( 1.887862790868997109, 13.79486065368817194, -27.89999999999996660 ) ) ;
#16168=CARTESIAN_POINT ( 'NONE',  ( -2.698247469942396837, 22.47571708489507358, -36.89295307432605142 ) ) ;
#16169=CARTESIAN_POINT ( 'NONE',  ( 0.6505131845895220088, 21.60717860451803674, -26.69999999999996732 ) ) ;
#16175=CARTESIAN_POINT ( 'NONE',  ( 3.895814058185739448, 19.48501640914375344, -48.14999999999997726 ) ) ;
#16178=CARTESIAN_POINT ( 'NONE',  ( 5.852430833189966819, 16.41846101382252243, -34.95704692567387895 ) ) ;
#16179=CARTESIAN_POINT ( 'NONE',  ( 2.568848540478311460, 12.45835086740561692, -30.89999999999996305 ) ) ;
#16180=CARTESIAN_POINT ( 'NONE',  ( -3.091735541773221296, 20.59173554177323950, -68.24999999999995737 ) ) ;
#16192=CARTESIAN_POINT ( 'NONE',  ( -1.081538986177402961, 23.35243083318996327, -46.04295307432605711 ) ) ;
#16207=CARTESIAN_POINT ( 'NONE',  ( -0.6839900399647736995, 21.81854315085035623, -50.54999999999996163 ) ) ;
#16218=CARTESIAN_POINT ( 'NONE',  ( 4.975717084895059372, 14.80175253005754143, -68.10704692567387042 ) ) ;
#16219=CARTESIAN_POINT ( 'NONE',  ( -4.001075405444606936, 13.49892459455542060, -52.49999999999996447 ) ) ;
#16234=CARTESIAN_POINT ( 'NONE',  ( 4.099003336600150149, 13.18504404629255689, -50.25704692567386900 ) ) ;
#16237=CARTESIAN_POINT ( 'NONE',  ( -5.900206406879871857, 18.27989588542834554, -72.44295307432605568 ) ) ;
#16255=CARTESIAN_POINT ( 'NONE',  ( -5.041649132594344884, 20.06884854047834921, -44.09999999999996589 ) ) ;
#16258=CARTESIAN_POINT ( 'NONE',  ( -0.5331684895902242260, 21.84243093769531185, -64.05704692567387326 ) ) ;
#16260=CARTESIAN_POINT ( 'NONE',  ( -0.6839900399647738105, 21.81854315085035623, -50.54999999999996163 ) ) ;
#16269=CARTESIAN_POINT ( 'NONE',  ( 3.705139346311793869, 15.61213720913094960, -60.59999999999996589 ) ) ;
#16271=CARTESIAN_POINT ( 'NONE',  ( 3.965139115708213868, 19.34895832295540430, -49.65704692567388179 ) ) ;
#16275=CARTESIAN_POINT ( 'NONE',  ( 3.826489000663266360, 19.62107449533211678, -40.64295307432606563 ) ) ;
#16290=CARTESIAN_POINT ( 'NONE',  ( 5.041649132594343996, 14.93115145952162415, -51.59999999999996589 ) ) ;
#16308=CARTESIAN_POINT ( 'NONE',  ( 2.701047200102605572, 22.80110361078655856, -68.84999999999996589 ) ) ;
#16313=CARTESIAN_POINT ( 'NONE',  ( -2.940415233664778860, 14.55958476633523802, -46.49999999999997158 ) ) ;
#16324=CARTESIAN_POINT ( 'NONE',  ( 2.837723661809363307, 20.54310680552015356, -55.49295307432605995 ) ) ;
#16340=CARTESIAN_POINT ( 'NONE',  ( 4.318543150850367773, 16.81600996003516357, -36.44999999999996732 ) ) ;
#16366=CARTESIAN_POINT ( 'NONE',  ( -3.965139115708213868, 15.65104167704456906, -30.15704692567386758 ) ) ;
#16371=CARTESIAN_POINT ( 'NONE',  ( 2.698247469942395949, 12.52428291510489977, -32.39295307432605142 ) ) ;
#16372=CARTESIAN_POINT ( 'NONE',  ( 0.7939530028709752552, 21.58445996917927445, -70.20704692567387895 ) ) ;
#16380=CARTESIAN_POINT ( 'NONE',  ( -3.705139346311794313, 19.38786279086902198, -47.09999999999996589 ) ) ;
#16383=CARTESIAN_POINT ( 'NONE',  ( 5.370428668309080500, 20.06498911391418360, -37.65704692567386758 ) ) ;
#16385=CARTESIAN_POINT ( 'NONE',  ( -4.318543150850367773, 18.18399003996480801, -67.94999999999994600 ) ) ;
#16398=CARTESIAN_POINT ( 'NONE',  ( 5.107581180293630396, 15.06055038898570686, -32.09295307432605426 ) ) ;
#16417=CARTESIAN_POINT ( 'NONE',  ( -4.318543150850367773, 18.18399003996480801, -25.94999999999996732 ) ) ;
#16418=CARTESIAN_POINT ( 'NONE',  ( -0.6505131845895224529, 13.39282139548194195, -52.19999999999996732 ) ) ;
#16427=CARTESIAN_POINT ( 'NONE',  ( 2.439449611014226971, 12.39241881970633230, -62.40704692567388179 ) ) ;
#16428=CARTESIAN_POINT ( 'NONE',  ( 4.206979645153768210, 13.29302035484617406, -57.74999999999996447 ) ) ;
#16439=CARTESIAN_POINT ( 'NONE',  ( 4.099003336600150149, 13.18504404629255689, -47.25704692567386900 ) ) ;
#16444=CARTESIAN_POINT ( 'NONE',  ( 2.564989113914249330, 22.87042866830903876, -61.34295307432606137 ) ) ;
#16460=CARTESIAN_POINT ( 'NONE',  ( -4.001075405444606936, 13.49892459455542060, -46.49999999999997158 ) ) ;
#16463=CARTESIAN_POINT ( 'NONE',  ( 2.121074495332174958, 21.32648900066323350, -61.35704692567387752 ) ) ;
#16464=CARTESIAN_POINT ( 'NONE',  ( 0.6505131845895220088, 21.60717860451803674, -44.69999999999996021 ) ) ;
#16474=CARTESIAN_POINT ( 'NONE',  ( -0.6839900399647736995, 21.81854315085035623, -65.54999999999996874 ) ) ;
#16476=CARTESIAN_POINT ( 'NONE',  ( 3.043106805520193525, 20.33772366180932067, -49.50704692567387610 ) ) ;
#16480=CARTESIAN_POINT ( 'NONE',  ( -0.5070733663080690956, 13.37010276014318144, -38.69295307432606279 ) ) ;
#16487=CARTESIAN_POINT ( 'NONE',  ( -4.975717084895059372, 20.19824746994243370, -72.60704692567387042 ) ) ;
#16496=CARTESIAN_POINT ( 'NONE',  ( -5.041649132594344884, 20.06884854047834921, -47.09999999999996589 ) ) ;
#16513=CARTESIAN_POINT ( 'NONE',  ( -5.301103610786608300, 14.79895279989743706, -67.64999999999997726 ) ) ;
#16519=CARTESIAN_POINT ( 'NONE',  ( -0.6839900399647736995, 21.81854315085035623, -41.54999999999996874 ) ) ;
#16520=CARTESIAN_POINT ( 'NONE',  ( -3.705139346311794313, 19.38786279086902198, -74.09999999999996589 ) ) ;
#16531=CARTESIAN_POINT ( 'NONE',  ( -0.5070733663080690956, 13.37010276014318144, -44.69295307432606279 ) ) ;
#16536=CARTESIAN_POINT ( 'NONE',  ( -1.848958322955462474, 13.53486088429179546, -59.84295307432606137 ) ) ;
#16547=CARTESIAN_POINT ( 'NONE',  ( 3.895814058185739448, 19.48501640914375344, -33.14999999999996305 ) ) ;
#16574=CARTESIAN_POINT ( 'NONE',  ( -0.7939530028709754772, 13.41554003082070246, -35.70704692567387184 ) ) ;
#16579=CARTESIAN_POINT ( 'NONE',  ( -2.564989113914250662, 12.12957133169093282, -32.84295307432606137 ) ) ;
#16580=CARTESIAN_POINT ( 'NONE',  ( -4.129897239856814117, 16.99292663369196177, -60.30704692567387326 ) ) ;
#16587=CARTESIAN_POINT ( 'NONE',  ( 0.6505131845895220088, 21.60717860451803674, -47.69999999999996732 ) ) ;
#16591=CARTESIAN_POINT ( 'NONE',  ( 5.611429750749524992, 18.24172506386835479, -34.80704692567387326 ) ) ;
#16593=CARTESIAN_POINT ( 'NONE',  ( -3.705139346311794313, 19.38786279086902198, -65.09999999999996589 ) ) ;
#16605=CARTESIAN_POINT ( 'NONE',  ( -5.107581180293630396, 19.93944961101426827, -33.59295307432606137 ) ) ;
#16621=CARTESIAN_POINT ( 'NONE',  ( -1.887862790868997553, 21.20513934631180319, -44.39999999999997016 ) ) ;
#16630=CARTESIAN_POINT ( 'NONE',  ( 3.705139346311793869, 15.61213720913094960, -72.59999999999996589 ) ) ;
#16632=CARTESIAN_POINT ( 'NONE',  ( 4.103766977300021601, 21.39838383358913987, -70.50704692567386189 ) ) ;
#16633=CARTESIAN_POINT ( 'NONE',  ( 5.041649132594343996, 14.93115145952162415, -42.59999999999996589 ) ) ;
#16647=CARTESIAN_POINT ( 'NONE',  ( -2.439449611014227859, 22.60758118029364283, -48.90704692567388179 ) ) ;
#16651=CARTESIAN_POINT ( 'NONE',  ( -4.314955953707389824, 21.59900333660018390, -60.74295307432605995 ) ) ;
#16667=CARTESIAN_POINT ( 'NONE',  ( 5.041649132594343996, 14.93115145952162415, -33.59999999999996589 ) ) ;
#16670=CARTESIAN_POINT ( 'NONE',  ( 3.965139115708213868, 19.34895832295540430, -49.65704692567388179 ) ) ;
#16672=CARTESIAN_POINT ( 'NONE',  ( -4.318543150850366885, 18.18399003996480801, -43.94999999999996021 ) ) ;
#16682=CARTESIAN_POINT ( 'NONE',  ( -0.6839900399647736995, 21.81854315085035623, -53.54999999999996163 ) ) ;
#16685=CARTESIAN_POINT ( 'NONE',  ( -4.129897239856814117, 16.99292663369196177, -48.30704692567388037 ) ) ;
#16689=CARTESIAN_POINT ( 'NONE',  ( -2.837723661809363751, 14.45689319447982335, -35.99295307432605995 ) ) ;
#16695=CARTESIAN_POINT ( 'NONE',  ( -1.028604700431329233, 11.93400751992799513, -71.70704692567387895 ) ) ;
#16700=CARTESIAN_POINT ( 'NONE',  ( -2.701047200102606016, 12.19889638921340413, -34.34999999999995879 ) ) ;
#16717=CARTESIAN_POINT ( 'NONE',  ( -5.588711115410763597, 16.61483511785016987, -70.79999999999996874 ) ) ;
#16722=CARTESIAN_POINT ( 'NONE',  ( -4.318543150850367773, 18.18399003996480801, -28.94999999999996021 ) ) ;
#16734=CARTESIAN_POINT ( 'NONE',  ( 0.8348115903393232839, 13.20534463599456387, -44.54295307432605711 ) ) ;
#16739=CARTESIAN_POINT ( 'NONE',  ( -2.017261720333081598, 21.13920729861251857, -60.89295307432605853 ) ) ;
#16750=CARTESIAN_POINT ( 'NONE',  ( 3.895814058185739448, 19.48501640914375344, -27.14999999999995595 ) ) ;
#16760=CARTESIAN_POINT ( 'NONE',  ( -0.8851648821498765418, 11.91128888458923285, -70.19999999999997442 ) ) ;
#16776=CARTESIAN_POINT ( 'NONE',  ( -5.107581180293630396, 19.93944961101426827, -63.59295307432605426 ) ) ;
#16781=CARTESIAN_POINT ( 'NONE',  ( -2.121074495332175847, 13.67351099933674341, -35.85704692567387752 ) ) ;
#16785=CARTESIAN_POINT ( 'NONE',  ( -4.314955953707389824, 21.59900333660018390, -27.74295307432605995 ) ) ;
#16786=CARTESIAN_POINT ( 'NONE',  ( 2.121074495332174958, 21.32648900066323350, -67.35704692567388463 ) ) ;
#16793=CARTESIAN_POINT ( 'NONE',  ( -0.6505131845895224529, 13.39282139548194195, -40.19999999999996732 ) ) ;
#16796=CARTESIAN_POINT ( 'NONE',  ( 4.975717084895059372, 14.80175253005754143, -29.10704692567387752 ) ) ;
#16797=CARTESIAN_POINT ( 'NONE',  ( -3.091735541773221296, 20.59173554177323950, -53.24999999999996447 ) ) ;
#16809=CARTESIAN_POINT ( 'NONE',  ( 2.564989113914249330, 22.87042866830903876, -31.34295307432605782 ) ) ;
#16828=CARTESIAN_POINT ( 'NONE',  ( 0.6839900399647733664, 13.18145684914961357, -49.04999999999994742 ) ) ;
#16838=CARTESIAN_POINT ( 'NONE',  ( -4.318543150850367773, 18.18399003996480801, -73.94999999999997442 ) ) ;
#16840=CARTESIAN_POINT ( 'NONE',  ( 0.7798958854283032371, 11.59979359312010772, -53.55704692567387326 ) ) ;
#16841=CARTESIAN_POINT ( 'NONE',  ( 5.301103610786608300, 20.20104720010254340, -45.14999999999996305 ) ) ;
#16855=CARTESIAN_POINT ( 'NONE',  ( -2.837105286290963146, 12.26822144673588255, -47.85704692567386331 ) ) ;
#16860=CARTESIAN_POINT ( 'NONE',  ( -5.900206406879871857, 18.27989588542834554, -60.44295307432605568 ) ) ;
#16874=CARTESIAN_POINT ( 'NONE',  ( 5.301103610786608300, 20.20104720010253985, -36.14999999999994884 ) ) ;
#16877=CARTESIAN_POINT ( 'NONE',  ( -2.983759233219601903, 20.69971185032686023, -48.75704692567386189 ) ) ;
#16878=CARTESIAN_POINT ( 'NONE',  ( -4.318543150850366885, 18.18399003996480801, -40.94999999999996732 ) ) ;
#16879=CARTESIAN_POINT ( 'NONE',  ( -3.895814058185739448, 15.51498359085620571, -70.64999999999996305 ) ) ;
#16888=CARTESIAN_POINT ( 'NONE',  ( 4.318543150850367773, 16.81600996003516357, -57.44999999999996732 ) ) ;
#16890=CARTESIAN_POINT ( 'NONE',  ( 3.639207298612508801, 15.48273827966686866, -41.10704692567387752 ) ) ;
#16891=CARTESIAN_POINT ( 'NONE',  ( -0.9307174358028534877, 23.37631862003491889, -71.54999999999995453 ) ) ;
#16893=CARTESIAN_POINT ( 'NONE',  ( 2.017261720333081598, 13.86079270138745834, -32.39295307432605142 ) ) ;
#16900=CARTESIAN_POINT ( 'NONE',  ( -5.370428668309080500, 14.93501088608579153, -72.15704692567386758 ) ) ;
#16906=CARTESIAN_POINT ( 'NONE',  ( 2.568848540478311460, 12.45835086740561692, -42.89999999999996305 ) ) ;
#16924=CARTESIAN_POINT ( 'NONE',  ( 5.041649132594343996, 14.93115145952162415, -60.59999999999996589 ) ) ;
#16929=CARTESIAN_POINT ( 'NONE',  ( -4.107178604518053611, 16.84948681541050775, -34.79999999999996163 ) ) ;
#16930=CARTESIAN_POINT ( 'NONE',  ( -4.318543150850366885, 18.18399003996480801, -73.94999999999997442 ) ) ;
#16940=CARTESIAN_POINT ( 'NONE',  ( 2.017261720333081598, 13.86079270138745834, -44.39295307432605853 ) ) ;
#16945=MECHANICAL_DESIGN_GEOMETRIC_PRESENTATION_REPRESENTATION('',(#37321),#633);
#16946=CARTESIAN_POINT ( 'NONE',  ( -3.771071394011080269, 19.25846386140493394, -66.59295307432604716 ) ) ;
#16957=CARTESIAN_POINT ( 'NONE',  ( -3.895814058185739448, 15.51498359085620571, -25.64999999999996305 ) ) ;
#16966=CARTESIAN_POINT ( 'NONE',  ( -5.041649132594344884, 20.06884854047834921, -68.09999999999996589 ) ) ;
#16983=CARTESIAN_POINT ( 'NONE',  ( 5.565992480072003978, 18.52860470043125574, -67.79295307432606421 ) ) ;
#16993=CARTESIAN_POINT ( 'NONE',  ( -0.5070733663080690956, 13.37010276014318144, -74.69295307432606990 ) ) ;
#16994=CARTESIAN_POINT ( 'NONE',  ( 3.965139115708213868, 19.34895832295540430, -64.65704692567386758 ) ) ;
#17005=CARTESIAN_POINT ( 'NONE',  ( 5.370428668309080500, 20.06498911391418360, -25.65704692567387823 ) ) ;
#17007=CARTESIAN_POINT ( 'NONE',  ( 4.318543150850367773, 16.81600996003516357, -54.44999999999996021 ) ) ;
#17021=CARTESIAN_POINT ( 'NONE',  ( 5.900206406879871857, 16.72010411457162604, -28.94295307432605568 ) ) ;
#17040=CARTESIAN_POINT ( 'NONE',  ( 4.107178604518054499, 18.15051318458946383, -42.29999999999996874 ) ) ;
#17049=CARTESIAN_POINT ( 'NONE',  ( -4.318543150850367773, 18.18399003996480801, -67.94999999999994600 ) ) ;
#17051=CARTESIAN_POINT ( 'NONE',  ( 1.028604700431328567, 23.06599248007198355, -52.20704692567388605 ) ) ;
#17052=CARTESIAN_POINT ( 'NONE',  ( 0.8851648821498760977, 23.08871111541074228, -41.69999999999996732 ) ) ;
#17063=CARTESIAN_POINT ( 'NONE',  ( 1.028604700431328567, 23.06599248007198355, -46.20704692567387184 ) ) ;
#17070=CARTESIAN_POINT ( 'NONE',  ( -5.565992480072003978, 16.47139529956871229, -57.29295307432606421 ) ) ;
#17086=CARTESIAN_POINT ( 'NONE',  ( 4.206979645153767322, 13.29302035484617051, -36.74999999999994316 ) ) ;
#17089=CARTESIAN_POINT ( 'NONE',  ( -1.758463861404912842, 21.27107139401109137, -51.90704692567388179 ) ) ;
#17090=DIRECTION ( 'NONE',  ( -0.7071067811865510144, -0.7071067811865440200, 0.000000000000000000 ) ) ;
#17099=CARTESIAN_POINT ( 'NONE',  ( 4.107178604518054499, 18.15051318458946383, -54.29999999999996874 ) ) ;
#17102=CARTESIAN_POINT ( 'NONE',  ( 4.294655364005415699, 16.66518840966061887, -31.95704692567387184 ) ) ;
#17106=CARTESIAN_POINT ( 'NONE',  ( 1.848958322955461808, 21.46513911570817612, -31.34295307432605782 ) ) ;
#17114=CARTESIAN_POINT ( 'NONE',  ( 5.370428668309080500, 20.06498911391418360, -70.65704692567386758 ) ) ;
#17121=CARTESIAN_POINT ( 'NONE',  ( 0.9307174358028528216, 11.62368137996505801, -40.04999999999994742 ) ) ;
#17137=CARTESIAN_POINT ( 'NONE',  ( -5.301103610786608300, 14.79895279989743706, -64.64999999999994884 ) ) ;
#17142=CARTESIAN_POINT ( 'NONE',  ( 3.895814058185739448, 19.48501640914375344, -30.14999999999997016 ) ) ;
#17143=CARTESIAN_POINT ( 'NONE',  ( -4.107178604518053611, 16.84948681541050775, -70.79999999999996874 ) ) ;
#17155=CARTESIAN_POINT ( 'NONE',  ( 0.8348115903393232839, 13.20534463599456387, -41.54295307432605000 ) ) ;
#17162=CARTESIAN_POINT ( 'NONE',  ( 3.771071394011080269, 15.74153613859503764, -68.09295307432604716 ) ) ;
#17173=CARTESIAN_POINT ( 'NONE',  ( 0.6505131845895220088, 21.60717860451803674, -26.69999999999996732 ) ) ;
#17182=CARTESIAN_POINT ( 'NONE',  ( 0.9307174358028528216, 11.62368137996505801, -70.04999999999996874 ) ) ;
#17200=CARTESIAN_POINT ( 'NONE',  ( 2.564989113914249330, 22.87042866830903876, -58.34295307432606137 ) ) ;
#17208=CARTESIAN_POINT ( 'NONE',  ( -2.837723661809363751, 14.45689319447982335, -71.99295307432603863 ) ) ;
#17210=CARTESIAN_POINT ( 'NONE',  ( -1.758463861404912842, 21.27107139401109137, -66.90704692567388179 ) ) ;
#17224=CARTESIAN_POINT ( 'NONE',  ( 5.852430833189966819, 16.41846101382252243, -28.95704692567387184 ) ) ;
#17226=CARTESIAN_POINT ( 'NONE',  ( 0.6505131845895220088, 21.60717860451803674, -59.69999999999996732 ) ) ;
#17238=CARTESIAN_POINT ( 'NONE',  ( -5.107581180293630396, 19.93944961101426827, -30.59295307432605782 ) ) ;
#17257=CARTESIAN_POINT ( 'NONE',  ( -3.895814058185739448, 15.51498359085620571, -40.64999999999994174 ) ) ;
#17265=CARTESIAN_POINT ( 'NONE',  ( -1.985016409143819605, 13.60418594181426855, -64.34999999999996589 ) ) ;
#17267=CARTESIAN_POINT ( 'NONE',  ( -5.852430833189966819, 18.58153898617744915, -60.45704692567387895 ) ) ;
#17268=CARTESIAN_POINT ( 'NONE',  ( 0.9307174358028527106, 11.62368137996505801, -49.04999999999995453 ) ) ;
#17281=CARTESIAN_POINT ( 'NONE',  ( 0.7798958854283032371, 11.59979359312010772, -44.55704692567387326 ) ) ;
#17287=CARTESIAN_POINT ( 'NONE',  ( -0.7417250638684240727, 11.88857024925047057, -62.69295307432606279 ) ) ;
#17301=CARTESIAN_POINT ( 'NONE',  ( 0.8851648821498760977, 23.08871111541074228, -35.69999999999996732 ) ) ;
#17305=CARTESIAN_POINT ( 'NONE',  ( 3.639207298612508801, 15.48273827966686866, -56.10704692567387752 ) ) ;
#17307=CARTESIAN_POINT ( 'NONE',  ( 3.895814058185739448, 19.48501640914375344, -72.14999999999996305 ) ) ;
#17316=CARTESIAN_POINT ( 'NONE',  ( -3.895814058185739448, 15.51498359085620571, -55.64999999999994174 ) ) ;
#17318=CARTESIAN_POINT ( 'NONE',  ( 4.129897239856814117, 18.00707336630801336, -37.80704692567387326 ) ) ;
#17328=CARTESIAN_POINT ( 'NONE',  ( -1.758463861404912842, 21.27107139401109137, -24.90704692567387823 ) ) ;
#17334=CARTESIAN_POINT ( 'NONE',  ( 4.001075405444606048, 21.50107540544455276, -41.99999999999996447 ) ) ;
#17351=CARTESIAN_POINT ( 'NONE',  ( -2.568848540478311904, 22.54164913259435465, -62.39999999999997016 ) ) ;
#17356=CARTESIAN_POINT ( 'NONE',  ( 3.895814058185739448, 19.48501640914375344, -36.14999999999994884 ) ) ;
#17357=CARTESIAN_POINT ( 'NONE',  ( 2.940415233664778416, 20.44041523366473712, -68.99999999999995737 ) ) ;
#17369=CARTESIAN_POINT ( 'NONE',  ( -2.017261720333081598, 21.13920729861251857, -42.89295307432605853 ) ) ;
#17374=CARTESIAN_POINT ( 'NONE',  ( -3.199711850326840246, 20.48375923321962233, -66.74295307432606705 ) ) ;
#17384=CARTESIAN_POINT ( 'NONE',  ( 3.895814058185739448, 19.48501640914375344, -30.14999999999997016 ) ) ;
#17392=CARTESIAN_POINT ( 'NONE',  ( 5.876318620034919782, 16.56928256419707068, -63.44999999999996732 ) ) ;
#17416=CARTESIAN_POINT ( 'NONE',  ( -5.107581180293630396, 19.93944961101426827, -54.59295307432605426 ) ) ;
#17425=CARTESIAN_POINT ( 'NONE',  ( 0.8348115903393232839, 13.20534463599456387, -71.54295307432605000 ) ) ;
#17427=CARTESIAN_POINT ( 'NONE',  ( 4.129897239856814117, 18.00707336630801336, -64.80704692567387326 ) ) ;
#17439=CARTESIAN_POINT ( 'NONE',  ( -4.099003336600151925, 21.81495595370741469, -24.75704692567387610 ) ) ;
#17441=CARTESIAN_POINT ( 'NONE',  ( 1.985016409143818272, 21.39581405818570303, -50.84999999999997300 ) ) ;
#17453=CARTESIAN_POINT ( 'NONE',  ( -1.848958322955462474, 13.53486088429179546, -71.84295307432606137 ) ) ;
#17470=CARTESIAN_POINT ( 'NONE',  ( 3.895814058185739448, 19.48501640914375344, -42.14999999999996305 ) ) ;
#17479=CARTESIAN_POINT ( 'NONE',  ( -0.6839900399647736995, 21.81854315085035623, -62.54999999999996874 ) ) ;
#17480=CARTESIAN_POINT ( 'NONE',  ( -2.439449611014227859, 22.60758118029364283, -51.90704692567388179 ) ) ;
#17481=CARTESIAN_POINT ( 'NONE',  ( -5.876318620034919782, 18.43071743580290089, -49.94999999999995310 ) ) ;
#17494=CARTESIAN_POINT ( 'NONE',  ( -2.439449611014227859, 22.60758118029364283, -36.90704692567386758 ) ) ;
#17497=CARTESIAN_POINT ( 'NONE',  ( 2.564989113914249330, 22.87042866830903876, -49.34295307432604716 ) ) ;
#17510=CARTESIAN_POINT ( 'NONE',  ( 5.588711115410763597, 18.38516488214980882, -36.29999999999996163 ) ) ;
#17513=CARTESIAN_POINT ( 'NONE',  ( -3.965139115708213868, 15.65104167704456906, -48.15704692567388179 ) ) ;
#17522=CARTESIAN_POINT ( 'NONE',  ( -3.705139346311794313, 19.38786279086902198, -56.09999999999996589 ) ) ;
#17524=CARTESIAN_POINT ( 'NONE',  ( 0.7939530028709752552, 21.58445996917927445, -37.20704692567387184 ) ) ;
#17534=CARTESIAN_POINT ( 'NONE',  ( -1.028604700431329233, 11.93400751992799513, -62.70704692567387184 ) ) ;
#17539=CARTESIAN_POINT ( 'NONE',  ( 5.041649132594343996, 14.93115145952162415, -42.59999999999996589 ) ) ;
#17558=CARTESIAN_POINT ( 'NONE',  ( -2.701047200102606016, 12.19889638921340413, -64.34999999999996589 ) ) ;
#17563=CARTESIAN_POINT ( 'NONE',  ( -3.091735541773221296, 20.59173554177323950, -29.24999999999996447 ) ) ;
#17564=CARTESIAN_POINT ( 'NONE',  ( -0.6839900399647738105, 21.81854315085035623, -71.54999999999995453 ) ) ;
#17575=CARTESIAN_POINT ( 'NONE',  ( 0.5070733663080689846, 21.62989723985679902, -37.19295307432606279 ) ) ;
#17580=CARTESIAN_POINT ( 'NONE',  ( 0.5070733663080689846, 21.62989723985679902, -58.19295307432606279 ) ) ;
#17599=CARTESIAN_POINT ( 'NONE',  ( -5.041649132594344884, 20.06884854047834921, -71.09999999999996589 ) ) ;
#17619=CARTESIAN_POINT ( 'NONE',  ( 2.564989113914249330, 22.87042866830903876, -52.34295307432604716 ) ) ;
#17627=CARTESIAN_POINT ( 'NONE',  ( -3.898383833589191827, 13.39623302270000771, -26.99295307432605995 ) ) ;
#17629=CARTESIAN_POINT ( 'NONE',  ( 3.639207298612508801, 15.48273827966686866, -50.10704692567387752 ) ) ;
#17643=CARTESIAN_POINT ( 'NONE',  ( -2.940415233664778860, 14.55958476633523802, -52.49999999999996447 ) ) ;
#17654=CARTESIAN_POINT ( 'NONE',  ( 0.8348115903393232839, 13.20534463599456387, -74.54295307432605000 ) ) ;
#17668=CARTESIAN_POINT ( 'NONE',  ( 3.895814058185739892, 19.48501640914376054, -42.14999999999996305 ) ) ;
#17673=CARTESIAN_POINT ( 'NONE',  ( -3.091735541773221296, 20.59173554177323950, -32.24999999999996447 ) ) ;
#17682=CARTESIAN_POINT ( 'NONE',  ( -1.887862790868997553, 21.20513934631180319, -62.39999999999997016 ) ) ;
#17684=CARTESIAN_POINT ( 'NONE',  ( -5.611429750749524992, 16.75827493613162034, -54.30704692567388037 ) ) ;
#17685=CARTESIAN_POINT ( 'NONE',  ( -4.001075405444606936, 13.49892459455542060, -31.49999999999996447 ) ) ;
#17698=CARTESIAN_POINT ( 'NONE',  ( 2.439449611014226971, 12.39241881970633230, -35.40704692567386758 ) ) ;
#17701=CARTESIAN_POINT ( 'NONE',  ( 5.900206406879871857, 16.72010411457162604, -52.94295307432605568 ) ) ;
#17717=CARTESIAN_POINT ( 'NONE',  ( -5.900206406879871857, 18.27989588542834554, -69.44295307432605568 ) ) ;
#17720=CARTESIAN_POINT ( 'NONE',  ( 0.5331684895902240040, 13.15756906230466328, -47.55704692567388037 ) ) ;
#17728=CARTESIAN_POINT ( 'NONE',  ( -1.985016409143819605, 13.60418594181426855, -49.34999999999996589 ) ) ;
#17730=CARTESIAN_POINT ( 'NONE',  ( 3.043106805520193525, 20.33772366180932067, -37.50704692567386189 ) ) ;
#17731=CARTESIAN_POINT ( 'NONE',  ( -0.9307174358028534877, 23.37631862003491889, -74.54999999999995453 ) ) ;
#17743=CARTESIAN_POINT ( 'NONE',  ( 1.028604700431328567, 23.06599248007198355, -64.20704692567387895 ) ) ;
#17749=CARTESIAN_POINT ( 'NONE',  ( 5.301103610786608300, 20.20104720010253985, -33.14999999999996305 ) ) ;
#17765=CARTESIAN_POINT ( 'NONE',  ( 4.001075405444606048, 21.50107540544455276, -65.99999999999997158 ) ) ;
#17769=CARTESIAN_POINT ( 'NONE',  ( 4.294655364005415699, 16.66518840966061887, -67.95704692567387895 ) ) ;
#17771=CARTESIAN_POINT ( 'NONE',  ( 3.091735541773220852, 14.40826445822673740, -66.74999999999997158 ) ) ;
#17782=CARTESIAN_POINT ( 'NONE',  ( 3.826489000663266360, 19.62107449533211678, -31.64295307432605853 ) ) ;
#17785=CARTESIAN_POINT ( 'NONE',  ( -4.342430937695320736, 18.03316848959025620, -54.44295307432606990 ) ) ;
#17800=CARTESIAN_POINT ( 'NONE',  ( -4.206979645153768210, 21.70697964515380107, -56.24999999999995026 ) ) ;
#17822=CARTESIAN_POINT ( 'NONE',  ( -2.698247469942396837, 22.47571708489507358, -51.89295307432605853 ) ) ;
#17829=CARTESIAN_POINT ( 'NONE',  ( -2.017261720333081598, 21.13920729861251857, -66.89295307432607274 ) ) ;
#17831=CARTESIAN_POINT ( 'NONE',  ( 1.758463861404912620, 13.72892860598888731, -59.40704692567388179 ) ) ;
#17845=CARTESIAN_POINT ( 'NONE',  ( -0.6839900399647736995, 21.81854315085035623, -41.54999999999996874 ) ) ;
#17857=CARTESIAN_POINT ( 'NONE',  ( -4.084459969179292216, 16.70604699712905372, -75.29295307432605000 ) ) ;
#17871=CARTESIAN_POINT ( 'NONE',  ( 0.6839900399647732554, 13.18145684914961357, -37.04999999999996163 ) ) ;
#17878=CARTESIAN_POINT ( 'NONE',  ( -4.318543150850367773, 18.18399003996480801, -34.94999999999996732 ) ) ;
#17887=CARTESIAN_POINT ( 'NONE',  ( 1.887862790868997109, 13.79486065368817194, -60.89999999999997016 ) ) ;
#17889=CARTESIAN_POINT ( 'NONE',  ( -5.852430833189966819, 18.58153898617744915, -42.45704692567387184 ) ) ;
#17890=CARTESIAN_POINT ( 'NONE',  ( -2.701047200102606460, 12.19889638921340591, -40.34999999999996589 ) ) ;
#17893=CARTESIAN_POINT ( 'NONE',  ( 0.6505131845895220088, 21.60717860451803674, -71.69999999999997442 ) ) ;
#17903=CARTESIAN_POINT ( 'NONE',  ( -5.852430833189966819, 18.58153898617744915, -36.45704692567386473 ) ) ;
#17906=CARTESIAN_POINT ( 'NONE',  ( 2.564989113914249330, 22.87042866830903876, -52.34295307432604716 ) ) ;
#17924=CARTESIAN_POINT ( 'NONE',  ( -0.7417250638684240727, 11.88857024925047057, -74.69295307432606990 ) ) ;
#17928=CARTESIAN_POINT ( 'NONE',  ( -4.294655364005415699, 18.33481159033935626, -42.45704692567387184 ) ) ;
#17929=CARTESIAN_POINT ( 'NONE',  ( -1.887862790868997553, 21.20513934631180319, -32.39999999999996305 ) ) ;
#17930=CARTESIAN_POINT ( 'NONE',  ( -1.887862790868997553, 21.20513934631180319, -62.39999999999997016 ) ) ;
#17939=CARTESIAN_POINT ( 'NONE',  ( 1.758463861404912620, 13.72892860598888731, -29.40704692567386758 ) ) ;
#17940=CARTESIAN_POINT ( 'NONE',  ( 5.041649132594343996, 14.93115145952162415, -66.59999999999996589 ) ) ;
#17952=CARTESIAN_POINT ( 'NONE',  ( -4.103766977300021601, 13.60161616641083704, -66.00704692567386189 ) ) ;
#17955=CARTESIAN_POINT ( 'NONE',  ( 4.001075405444606048, 21.50107540544455276, -32.99999999999996447 ) ) ;
#17972=CARTESIAN_POINT ( 'NONE',  ( -4.001075405444606936, 13.49892459455542060, -55.49999999999996447 ) ) ;
#17977=CARTESIAN_POINT ( 'NONE',  ( -1.985016409143819605, 13.60418594181426855, -28.34999999999995524 ) ) ;
#17978=CARTESIAN_POINT ( 'NONE',  ( -1.887862790868997553, 21.20513934631180319, -56.39999999999996305 ) ) ;
#17984=CARTESIAN_POINT ( 'NONE',  ( -4.107178604518053611, 16.84948681541050775, -73.79999999999996874 ) ) ;
#17989=CARTESIAN_POINT ( 'NONE',  ( 3.771071394011080269, 15.74153613859503764, -41.09295307432606137 ) ) ;
#17992=CARTESIAN_POINT ( 'NONE',  ( 0.8348115903393232839, 13.20534463599456387, -53.54295307432606421 ) ) ;
#18007=CARTESIAN_POINT ( 'NONE',  ( -5.876318620034919782, 18.43071743580290089, -55.94999999999997442 ) ) ;
#18028=CARTESIAN_POINT ( 'NONE',  ( 4.314955953707388936, 13.40099666339979123, -53.24295307432605995 ) ) ;
#18038=CARTESIAN_POINT ( 'NONE',  ( 0.8348115903393232839, 13.20534463599456387, -65.54295307432606421 ) ) ;
#18041=CARTESIAN_POINT ( 'NONE',  ( 3.639207298612508801, 15.48273827966686866, -56.10704692567387752 ) ) ;
#18054=CARTESIAN_POINT ( 'NONE',  ( -0.6505131845895224529, 13.39282139548194195, -49.19999999999996732 ) ) ;
#18066=CARTESIAN_POINT ( 'NONE',  ( 2.017261720333081598, 13.86079270138745834, -71.39295307432605853 ) ) ;
#18079=CARTESIAN_POINT ( 'NONE',  ( -4.107178604518053611, 16.84948681541050775, -34.79999999999996163 ) ) ;
#18084=CARTESIAN_POINT ( 'NONE',  ( 0.6505131845895220088, 21.60717860451803674, -38.69999999999996021 ) ) ;
#18095=CARTESIAN_POINT ( 'NONE',  ( 3.091735541773220852, 14.40826445822673563, -54.74999999999997158 ) ) ;
#18097=CARTESIAN_POINT ( 'NONE',  ( 2.439449611014226971, 12.39241881970633230, -47.40704692567387468 ) ) ;
#18098=CARTESIAN_POINT ( 'NONE',  ( 4.001075405444606048, 21.50107540544455276, -35.99999999999996447 ) ) ;
#18101=CARTESIAN_POINT ( 'NONE',  ( -0.6839900399647736995, 21.81854315085035623, -74.54999999999994031 ) ) ;
#18112=CARTESIAN_POINT ( 'NONE',  ( -2.439449611014227859, 22.60758118029364283, -39.90704692567386758 ) ) ;
#18116=CARTESIAN_POINT ( 'NONE',  ( -5.565992480072003978, 16.47139529956871229, -54.29295307432607132 ) ) ;
#18133=CARTESIAN_POINT ( 'NONE',  ( 5.107581180293630396, 15.06055038898570686, -74.09295307432606137 ) ) ;
#18136=CARTESIAN_POINT ( 'NONE',  ( 2.983759233219601459, 14.30028814967311668, -47.25704692567386900 ) ) ;
#18137=CARTESIAN_POINT ( 'NONE',  ( 1.887862790868997109, 13.79486065368817194, -36.89999999999997016 ) ) ;
#18138=CARTESIAN_POINT ( 'NONE',  ( 0.6839900399647733664, 13.18145684914961357, -61.04999999999995453 ) ) ;
#18147=CARTESIAN_POINT ( 'NONE',  ( 3.965139115708213868, 19.34895832295540430, -28.65704692567387468 ) ) ;
#18148=CARTESIAN_POINT ( 'NONE',  ( -2.568848540478311904, 22.54164913259435465, -65.39999999999997726 ) ) ;
#18161=CARTESIAN_POINT ( 'NONE',  ( 2.439449611014226971, 12.39241881970633230, -62.40704692567388179 ) ) ;
#18165=CARTESIAN_POINT ( 'NONE',  ( 2.701047200102605572, 22.80110361078655856, -32.84999999999996589 ) ) ;
#18180=CARTESIAN_POINT ( 'NONE',  ( -2.701047200102606016, 12.19889638921340413, -55.34999999999997300 ) ) ;
#18184=CARTESIAN_POINT ( 'NONE',  ( 4.318543150850367773, 16.81600996003516357, -27.44999999999996021 ) ) ;
#18185=CARTESIAN_POINT ( 'NONE',  ( 3.895814058185739892, 19.48501640914376054, -57.14999999999995595 ) ) ;
#18191=CARTESIAN_POINT ( 'NONE',  ( -2.940415233664778860, 14.55958476633523802, -73.49999999999997158 ) ) ;
#18197=CARTESIAN_POINT ( 'NONE',  ( 4.084459969179292216, 18.29395300287091430, -40.79295307432605711 ) ) ;
#18200=CARTESIAN_POINT ( 'NONE',  ( 3.826489000663266360, 19.62107449533211678, -58.64295307432606563 ) ) ;
#18215=CARTESIAN_POINT ( 'NONE',  ( 5.876318620034919782, 16.56928256419707068, -54.44999999999996021 ) ) ;
#18235=CARTESIAN_POINT ( 'NONE',  ( -5.107581180293630396, 19.93944961101426827, -45.59295307432606137 ) ) ;
#18242=CARTESIAN_POINT ( 'NONE',  ( 4.342430937695320736, 16.96683151040971538, -64.94295307432605568 ) ) ;
#18257=CARTESIAN_POINT ( 'NONE',  ( -2.940415233664778860, 14.55958476633523802, -46.49999999999997158 ) ) ;
#18281=CARTESIAN_POINT ( 'NONE',  ( -3.705139346311794313, 19.38786279086902198, -38.09999999999996589 ) ) ;
#18285=CARTESIAN_POINT ( 'NONE',  ( 1.887862790868997109, 13.79486065368817194, -36.89999999999997016 ) ) ;
#18293=CARTESIAN_POINT ( 'NONE',  ( 3.705139346311793869, 15.61213720913094960, -57.59999999999997300 ) ) ;
#18295=CARTESIAN_POINT ( 'NONE',  ( 0.7798958854283032371, 11.59979359312010772, -44.55704692567387326 ) ) ;
#18296=CARTESIAN_POINT ( 'NONE',  ( 5.301103610786608300, 20.20104720010254340, -39.14999999999997016 ) ) ;
#18300=CARTESIAN_POINT ( 'NONE',  ( -4.107178604518053611, 16.84948681541050775, -73.79999999999996874 ) ) ;
#18310=CARTESIAN_POINT ( 'NONE',  ( 5.611429750749524992, 18.24172506386835479, -31.80704692567387326 ) ) ;
#18315=CARTESIAN_POINT ( 'NONE',  ( -5.107581180293630396, 19.93944961101426827, -54.59295307432605426 ) ) ;
#18335=CARTESIAN_POINT ( 'NONE',  ( -1.081538986177402961, 23.35243083318996327, -76.04295307432605000 ) ) ;
#18339=CARTESIAN_POINT ( 'NONE',  ( -3.639207298612509689, 19.51726172033310647, -39.60704692567387042 ) ) ;
#18340=CARTESIAN_POINT ( 'NONE',  ( -2.940415233664778860, 14.55958476633523802, -34.49999999999997158 ) ) ;
#18341=CARTESIAN_POINT ( 'NONE',  ( -1.887862790868997553, 21.20513934631180319, -65.39999999999997726 ) ) ;
#18352=CARTESIAN_POINT ( 'NONE',  ( 4.129897239856814117, 18.00707336630801336, -25.80704692567386971 ) ) ;
#18353=CARTESIAN_POINT ( 'NONE',  ( 5.588711115410763597, 18.38516488214980882, -63.29999999999996874 ) ) ;
#18367=CARTESIAN_POINT ( 'NONE',  ( -4.099003336600151925, 21.81495595370741469, -63.75704692567388321 ) ) ;
#18371=CARTESIAN_POINT ( 'NONE',  ( 5.588711115410763597, 18.38516488214980882, -33.29999999999996874 ) ) ;
#18389=CARTESIAN_POINT ( 'NONE',  ( -0.8851648821498765418, 11.91128888458923285, -55.19999999999997442 ) ) ;
#18393=CARTESIAN_POINT ( 'NONE',  ( -0.7939530028709754772, 13.41554003082070246, -68.70704692567387895 ) ) ;
#18394=CARTESIAN_POINT ( 'NONE',  ( 0.6505131845895220088, 21.60717860451803674, -62.69999999999996732 ) ) ;
#18405=CARTESIAN_POINT ( 'NONE',  ( -1.848958322955462474, 13.53486088429179546, -38.84295307432606137 ) ) ;
#18408=CARTESIAN_POINT ( 'NONE',  ( -3.199711850326840246, 20.48375923321962233, -54.74295307432605995 ) ) ;
#18412=CIRCLE ( 'NONE', #19114, 0.7500000000000009992 ) ;
#18424=CARTESIAN_POINT ( 'NONE',  ( 4.001075405444606048, 21.50107540544455276, -59.99999999999997158 ) ) ;
#18446=CARTESIAN_POINT ( 'NONE',  ( -2.698247469942396837, 22.47571708489507358, -48.89295307432605853 ) ) ;
#18455=CARTESIAN_POINT ( 'NONE',  ( 2.017261720333081598, 13.86079270138745834, -68.39295307432607274 ) ) ;
#18468=CARTESIAN_POINT ( 'NONE',  ( 3.091735541773220852, 14.40826445822673563, -48.74999999999997158 ) ) ;
#18492=CARTESIAN_POINT ( 'NONE',  ( 3.091735541773220852, 14.40826445822673740, -30.74999999999996092 ) ) ;
#18498=CARTESIAN_POINT ( 'NONE',  ( 2.940415233664778416, 20.44041523366473712, -38.99999999999996447 ) ) ;
#18507=CARTESIAN_POINT ( 'NONE',  ( 4.318543150850367773, 16.81600996003516357, -57.44999999999996732 ) ) ;
#18510=CARTESIAN_POINT ( 'NONE',  ( 1.028604700431328567, 23.06599248007198355, -43.20704692567387184 ) ) ;
#18511=CARTESIAN_POINT ( 'NONE',  ( 5.588711115410763597, 18.38516488214980882, -36.29999999999996163 ) ) ;
#18513=CARTESIAN_POINT ( 'NONE',  ( 0.6839900399647733664, 13.18145684914961357, -70.04999999999996874 ) ) ;
#18525=CARTESIAN_POINT ( 'NONE',  ( -5.370428668309080500, 14.93501088608579153, -27.15704692567387823 ) ) ;
#18530=CARTESIAN_POINT ( 'NONE',  ( -2.698247469942396837, 22.47571708489507358, -39.89295307432605853 ) ) ;
#18548=CARTESIAN_POINT ( 'NONE',  ( 2.564989113914249330, 22.87042866830903876, -76.34295307432604716 ) ) ;
#18552=CARTESIAN_POINT ( 'NONE',  ( 4.107178604518054499, 18.15051318458946383, -36.29999999999996163 ) ) ;
#18553=CARTESIAN_POINT ( 'NONE',  ( 0.6505131845895220088, 21.60717860451803674, -59.69999999999996732 ) ) ;
#18563=CARTESIAN_POINT ( 'NONE',  ( 3.965139115708213868, 19.34895832295540430, -25.65704692567387823 ) ) ;
#18564=CARTESIAN_POINT ( 'NONE',  ( -5.588711115410763597, 16.61483511785016987, -61.79999999999996874 ) ) ;
#18579=CARTESIAN_POINT ( 'NONE',  ( -5.611429750749524992, 16.75827493613162034, -51.30704692567388037 ) ) ;
#18584=CARTESIAN_POINT ( 'NONE',  ( 4.001075405444606048, 21.50107540544455276, -29.99999999999996447 ) ) ;
#18603=CARTESIAN_POINT ( 'NONE',  ( -5.301103610786608300, 14.79895279989743706, -55.64999999999994174 ) ) ;
#18607=CARTESIAN_POINT ( 'NONE',  ( -3.895814058185739448, 15.51498359085620571, -28.64999999999995950 ) ) ;
#18608=CARTESIAN_POINT ( 'NONE',  ( 3.895814058185739892, 19.48501640914376054, -60.14999999999996305 ) ) ;
#18615=FACE_OUTER_BOUND ( 'NONE', #3113, .T. ) ;
#18619=CARTESIAN_POINT ( 'NONE',  ( 1.985016409143818272, 21.39581405818570303, -71.84999999999998010 ) ) ;
#18622=CARTESIAN_POINT ( 'NONE',  ( 2.837723661809363307, 20.54310680552015356, -46.49295307432606705 ) ) ;
#18639=CARTESIAN_POINT ( 'NONE',  ( -0.8851648821498765418, 11.91128888458923285, -58.19999999999996732 ) ) ;
#18660=CARTESIAN_POINT ( 'NONE',  ( -0.7417250638684240727, 11.88857024925047057, -41.69295307432606279 ) ) ;
#18669=CARTESIAN_POINT ( 'NONE',  ( -3.826489000663265472, 15.37892550466785480, -57.14295307432605142 ) ) ;
#18683=CARTESIAN_POINT ( 'NONE',  ( -3.895814058185739448, 15.51498359085620571, -46.64999999999994884 ) ) ;
#18695=ORIENTED_EDGE ( 'NONE', *, *, #8142, .F. ) ;
#18710=CARTESIAN_POINT ( 'NONE',  ( -1.985016409143819605, 13.60418594181426855, -28.34999999999996234 ) ) ;
#18715=CARTESIAN_POINT ( 'NONE',  ( 1.887862790868997109, 13.79486065368817194, -27.89999999999996660 ) ) ;
#18724=CARTESIAN_POINT ( 'NONE',  ( -3.091735541773221296, 20.59173554177323950, -56.24999999999995026 ) ) ;
#18726=CARTESIAN_POINT ( 'NONE',  ( 1.028604700431328567, 23.06599248007198355, -49.20704692567387184 ) ) ;
#18727=CARTESIAN_POINT ( 'NONE',  ( -0.9307174358028534877, 23.37631862003491889, -29.54999999999996518 ) ) ;
#18728=CARTESIAN_POINT ( 'NONE',  ( -2.017261720333081598, 21.13920729861251857, -27.89295307432605853 ) ) ;
#18738=CARTESIAN_POINT ( 'NONE',  ( 5.611429750749524992, 18.24172506386835479, -28.80704692567387326 ) ) ;
#18742=CARTESIAN_POINT ( 'NONE',  ( 5.231778553264135212, 20.33710528629089254, -43.64295307432605853 ) ) ;
#18760=CARTESIAN_POINT ( 'NONE',  ( 5.231778553264135212, 20.33710528629089254, -61.64295307432606563 ) ) ;
#18766=CARTESIAN_POINT ( 'NONE',  ( 3.705139346311793869, 15.61213720913094960, -36.59999999999996589 ) ) ;
#18767=CARTESIAN_POINT ( 'NONE',  ( 3.895814058185739448, 19.48501640914375344, -66.14999999999997726 ) ) ;
#18776=CARTESIAN_POINT ( 'NONE',  ( 0.7939530028709752552, 21.58445996917927445, -25.20704692567387539 ) ) ;
#18777=CARTESIAN_POINT ( 'NONE',  ( -5.301103610786608300, 14.79895279989743528, -61.64999999999996305 ) ) ;
#18789=CARTESIAN_POINT ( 'NONE',  ( 2.439449611014226971, 12.39241881970633230, -56.40704692567388179 ) ) ;
#18792=CARTESIAN_POINT ( 'NONE',  ( 2.564989113914249330, 22.87042866830903876, -73.34295307432607558 ) ) ;
#18807=CARTESIAN_POINT ( 'NONE',  ( -2.701047200102606016, 12.19889638921340413, -52.34999999999994458 ) ) ;
#18811=CARTESIAN_POINT ( 'NONE',  ( 3.639207298612508801, 15.48273827966686866, -65.10704692567387042 ) ) ;
#18812=CARTESIAN_POINT ( 'NONE',  ( 1.887862790868997109, 13.79486065368817194, -54.89999999999996305 ) ) ;
#18819=CARTESIAN_POINT ( 'NONE',  ( -0.6839900399647736995, 21.81854315085035623, -59.54999999999994742 ) ) ;
#18821=CARTESIAN_POINT ( 'NONE',  ( -4.294655364005415699, 18.33481159033935626, -51.45704692567387895 ) ) ;
#18824=CARTESIAN_POINT ( 'NONE',  ( -4.107178604518053611, 16.84948681541050775, -70.79999999999996874 ) ) ;
#18827=CARTESIAN_POINT ( 'NONE',  ( 0.5070733663080689846, 21.62989723985679902, -43.19295307432606279 ) ) ;
#18843=CARTESIAN_POINT ( 'NONE',  ( -4.206979645153768210, 21.70697964515380107, -44.24999999999997868 ) ) ;
#18849=FACE_OUTER_BOUND ( 'NONE', #21052, .T. ) ;
#18863=CARTESIAN_POINT ( 'NONE',  ( -1.985016409143819605, 13.60418594181426855, -46.34999999999997300 ) ) ;
#18864=CARTESIAN_POINT ( 'NONE',  ( -4.314955953707389824, 21.59900333660018390, -48.74295307432605284 ) ) ;
#18873=CARTESIAN_POINT ( 'NONE',  ( 2.017261720333081598, 13.86079270138745834, -56.39295307432605853 ) ) ;
#18912=CARTESIAN_POINT ( 'NONE',  ( -4.318543150850366885, 18.18399003996480801, -28.94999999999996021 ) ) ;
#18915=CARTESIAN_POINT ( 'NONE',  ( -2.698247469942396837, 22.47571708489507358, -33.89295307432605142 ) ) ;
#18916=CARTESIAN_POINT ( 'NONE',  ( 3.043106805520193525, 20.33772366180932067, -73.50704692567386189 ) ) ;
#18924=CARTESIAN_POINT ( 'NONE',  ( -2.940415233664778860, 14.55958476633523802, -52.49999999999996447 ) ) ;
#18928=CARTESIAN_POINT ( 'NONE',  ( 0.7798958854283032371, 11.59979359312010772, -32.55704692567387326 ) ) ;
#18929=CARTESIAN_POINT ( 'NONE',  ( -0.8851648821498765418, 11.91128888458923285, -28.19999999999996732 ) ) ;
#18930=CARTESIAN_POINT ( 'NONE',  ( -2.940415233664778860, 14.55958476633523802, -61.49999999999997158 ) ) ;
#18941=CARTESIAN_POINT ( 'NONE',  ( 2.568848540478311460, 12.45835086740561692, -72.89999999999996305 ) ) ;
#18949=CARTESIAN_POINT ( 'NONE',  ( -4.314955953707389824, 21.59900333660018390, -45.74295307432605995 ) ) ;
#18964=CARTESIAN_POINT ( 'NONE',  ( 2.698247469942395949, 12.52428291510489977, -65.39295307432605853 ) ) ;
#18969=CARTESIAN_POINT ( 'NONE',  ( -4.107178604518053611, 16.84948681541050775, -28.79999999999996518 ) ) ;
#18970=CARTESIAN_POINT ( 'NONE',  ( 1.887862790868997109, 13.79486065368817194, -54.89999999999996305 ) ) ;
#18983=CARTESIAN_POINT ( 'NONE',  ( -0.7798958854283041253, 23.40020640687986386, -70.05704692567387326 ) ) ;
#18984=CARTESIAN_POINT ( 'NONE',  ( 0.8851648821498760977, 23.08871111541074228, -50.69999999999996732 ) ) ;
#18996=CARTESIAN_POINT ( 'NONE',  ( -2.439449611014227859, 22.60758118029364283, -54.90704692567386758 ) ) ;
#18999=CARTESIAN_POINT ( 'NONE',  ( -4.314955953707389824, 21.59900333660018390, -69.74295307432603863 ) ) ;
#19017=CARTESIAN_POINT ( 'NONE',  ( -2.701047200102606016, 12.19889638921340413, -43.34999999999994458 ) ) ;
#19021=CARTESIAN_POINT ( 'NONE',  ( -3.965139115708213868, 15.65104167704456906, -63.15704692567388179 ) ) ;
#19022=CARTESIAN_POINT ( 'NONE',  ( -1.887862790868997553, 21.20513934631180319, -47.39999999999997016 ) ) ;
#19030=CARTESIAN_POINT ( 'NONE',  ( 0.6839900399647733664, 13.18145684914961357, -64.04999999999994031 ) ) ;
#19033=CARTESIAN_POINT ( 'NONE',  ( 2.121074495332174958, 21.32648900066323350, -55.35704692567387752 ) ) ;
#19035=CARTESIAN_POINT ( 'NONE',  ( 1.985016409143818272, 21.39581405818570303, -74.84999999999993747 ) ) ;
#19039=CARTESIAN_POINT ( 'NONE',  ( -4.342430937695320736, 18.03316848959025620, -48.44295307432605568 ) ) ;
#19052=CARTESIAN_POINT ( 'NONE',  ( -2.701047200102606016, 12.19889638921340413, -46.34999999999997300 ) ) ;
#19067=CARTESIAN_POINT ( 'NONE',  ( 0.9307174358028528216, 11.62368137996505801, -73.04999999999998295 ) ) ;
#19072=CARTESIAN_POINT ( 'NONE',  ( -1.887862790868997553, 21.20513934631180319, -44.39999999999997016 ) ) ;
#19074=CARTESIAN_POINT ( 'NONE',  ( 5.231778553264135212, 20.33710528629089254, -46.64295307432605853 ) ) ;
#19084=CARTESIAN_POINT ( 'NONE',  ( 0.8348115903393232839, 13.20534463599456387, -53.54295307432606421 ) ) ;
#19099=CARTESIAN_POINT ( 'NONE',  ( -2.940415233664778860, 14.55958476633523802, -40.49999999999996447 ) ) ;
#19101=DIRECTION ( 'NONE',  ( 0.7071067811865513475, 0.7071067811865437980, 0.000000000000000000 ) ) ;
#19114=AXIS2_PLACEMENT_3D ( 'NONE', #36442, #7519, #17090 ) ;
#19128=CARTESIAN_POINT ( 'NONE',  ( 0.5331684895902240040, 13.15756906230466328, -29.55704692567387681 ) ) ;
#19129=CARTESIAN_POINT ( 'NONE',  ( 4.318543150850366885, 16.81600996003516713, -30.44999999999996021 ) ) ;
#19132=CARTESIAN_POINT ( 'NONE',  ( 5.565992480072003978, 18.52860470043125574, -34.79295307432605711 ) ) ;
#19133=CARTESIAN_POINT ( 'NONE',  ( 2.121074495332174958, 21.32648900066323350, -73.35704692567385621 ) ) ;
#19140=CARTESIAN_POINT ( 'NONE',  ( -1.887862790868997553, 21.20513934631180319, -50.39999999999996305 ) ) ;
#19143=CARTESIAN_POINT ( 'NONE',  ( 4.099003336600150149, 13.18504404629255689, -41.25704692567387610 ) ) ;
#19144=CARTESIAN_POINT ( 'NONE',  ( -5.588711115410763597, 16.61483511785016987, -28.79999999999996518 ) ) ;
#19145=CARTESIAN_POINT ( 'NONE',  ( 4.318543150850367773, 16.81600996003516357, -63.44999999999996732 ) ) ;
#19153=CARTESIAN_POINT ( 'NONE',  ( 5.876318620034919782, 16.56928256419707068, -72.44999999999994600 ) ) ;
#19158=CARTESIAN_POINT ( 'NONE',  ( -5.900206406879871857, 18.27989588542834554, -45.44295307432605568 ) ) ;
#19175=CARTESIAN_POINT ( 'NONE',  ( 3.898383833589191383, 21.60376697729997275, -67.49295307432606705 ) ) ;
#19180=CARTESIAN_POINT ( 'NONE',  ( 0.6505131845895220088, 21.60717860451803674, -29.69999999999996376 ) ) ;
#19181=CARTESIAN_POINT ( 'NONE',  ( -0.6505131845895224529, 13.39282139548194195, -58.19999999999996732 ) ) ;
#19192=CARTESIAN_POINT ( 'NONE',  ( -2.439449611014227859, 22.60758118029364283, -63.90704692567388179 ) ) ;
#19193=CARTESIAN_POINT ( 'NONE',  ( -4.206979645153769098, 21.70697964515380107, -59.24999999999997158 ) ) ;
#19205=CARTESIAN_POINT ( 'NONE',  ( -1.028604700431329233, 11.93400751992799513, -53.70704692567388605 ) ) ;
#19209=CARTESIAN_POINT ( 'NONE',  ( -5.231778553264134324, 14.66289471370907727, -69.14295307432605853 ) ) ;
#19227=CARTESIAN_POINT ( 'NONE',  ( 0.9307174358028528216, 11.62368137996505801, -40.04999999999994742 ) ) ;
#19231=CARTESIAN_POINT ( 'NONE',  ( 1.758463861404912620, 13.72892860598888731, -65.40704692567388179 ) ) ;
#19232=CARTESIAN_POINT ( 'NONE',  ( -4.318543150850366885, 18.18399003996480801, -46.94999999999996021 ) ) ;
#19241=CARTESIAN_POINT ( 'NONE',  ( -4.107178604518053611, 16.84948681541050775, -61.79999999999996874 ) ) ;
#19244=CARTESIAN_POINT ( 'NONE',  ( -2.983759233219601903, 20.69971185032686023, -48.75704692567386189 ) ) ;
#19249=CARTESIAN_POINT ( 'NONE',  ( -2.837723661809363751, 14.45689319447982335, -47.99295307432606705 ) ) ;
#19261=CARTESIAN_POINT ( 'NONE',  ( -0.9307174358028533767, 23.37631862003491889, -47.54999999999997584 ) ) ;
#19278=CARTESIAN_POINT ( 'NONE',  ( 5.301103610786608300, 20.20104720010253985, -66.14999999999997726 ) ) ;
#19283=CARTESIAN_POINT ( 'NONE',  ( 0.6839900399647733664, 13.18145684914961357, -46.04999999999996163 ) ) ;
#19293=CARTESIAN_POINT ( 'NONE',  ( -3.771071394011080269, 19.25846386140493394, -51.59295307432605426 ) ) ;
#19308=CARTESIAN_POINT ( 'NONE',  ( -1.887862790868997553, 21.20513934631180319, -38.39999999999997016 ) ) ;
#19334=CARTESIAN_POINT ( 'NONE',  ( 2.983759233219601459, 14.30028814967311668, -32.25704692567387610 ) ) ;
#19335=CARTESIAN_POINT ( 'NONE',  ( 1.985016409143818272, 21.39581405818570659, -32.84999999999996589 ) ) ;
#19338=CARTESIAN_POINT ( 'NONE',  ( 2.564989113914249330, 22.87042866830903876, -31.34295307432605782 ) ) ;
#19339=CARTESIAN_POINT ( 'NONE',  ( -0.5331684895902242260, 21.84243093769531185, -73.05704692567387326 ) ) ;
#19346=CARTESIAN_POINT ( 'NONE',  ( 2.940415233664778416, 20.44041523366473712, -44.99999999999997158 ) ) ;
#19349=CARTESIAN_POINT ( 'NONE',  ( 1.028604700431328567, 23.06599248007198355, -40.20704692567387184 ) ) ;
#19350=CARTESIAN_POINT ( 'NONE',  ( 4.206979645153768210, 13.29302035484617406, -27.74999999999995737 ) ) ;
#19351=CARTESIAN_POINT ( 'NONE',  ( 1.985016409143818272, 21.39581405818570303, -65.84999999999992326 ) ) ;
#19368=CARTESIAN_POINT ( 'NONE',  ( -5.107581180293630396, 19.93944961101426827, -42.59295307432605426 ) ) ;
#19388=CARTESIAN_POINT ( 'NONE',  ( 2.940415233664778416, 20.44041523366473712, -50.99999999999997158 ) ) ;
#19399=CARTESIAN_POINT ( 'NONE',  ( -4.103766977300021601, 13.60161616641083704, -63.00704692567389031 ) ) ;
#19400=CARTESIAN_POINT ( 'NONE',  ( 4.001075405444606048, 21.50107540544455276, -56.99999999999996447 ) ) ;
#19413=CARTESIAN_POINT ( 'NONE',  ( 0.7798958854283032371, 11.59979359312010772, -50.55704692567388747 ) ) ;
#19418=CARTESIAN_POINT ( 'NONE',  ( 5.107581180293630396, 15.06055038898570686, -71.09295307432604716 ) ) ;
#19433=CARTESIAN_POINT ( 'NONE',  ( 5.876318620034919782, 16.56928256419707068, -42.44999999999996732 ) ) ;
#19437=CARTESIAN_POINT ( 'NONE',  ( -1.758463861404912842, 21.27107139401109137, -60.90704692567388179 ) ) ;
#19438=CARTESIAN_POINT ( 'NONE',  ( 0.6505131845895220088, 21.60717860451803674, -50.69999999999996732 ) ) ;
#19442=EDGE_CURVE ( 'NONE', #3983, #21597, #18412, .T. ) ;
#19449=CARTESIAN_POINT ( 'NONE',  ( 2.940415233664778416, 20.44041523366473712, -68.99999999999995737 ) ) ;
#19450=ADVANCED_FACE ( 'NONE', ( #13682 ), #31982, .T. ) ;
#19452=CARTESIAN_POINT ( 'NONE',  ( -1.758463861404912842, 21.27107139401109137, -42.90704692567387468 ) ) ;
#19456=CARTESIAN_POINT ( 'NONE',  ( 4.342430937695320736, 16.96683151040971538, -40.94295307432605568 ) ) ;
#19471=CARTESIAN_POINT ( 'NONE',  ( 0.8851648821498760977, 23.08871111541074228, -44.69999999999996021 ) ) ;
#19476=ORIENTED_EDGE ( 'NONE', *, *, #19680, .T. ) ;
#19485=CARTESIAN_POINT ( 'NONE',  ( 0.8851648821498760977, 23.08871111541074228, -71.69999999999997442 ) ) ;
#19490=CARTESIAN_POINT ( 'NONE',  ( -4.318543150850367773, 18.18399003996480801, -46.94999999999996021 ) ) ;
#19491=CARTESIAN_POINT ( 'NONE',  ( -3.091735541773221296, 20.59173554177323950, -74.24999999999997158 ) ) ;
#19501=CARTESIAN_POINT ( 'NONE',  ( -1.848958322955462474, 13.53486088429179546, -53.84295307432606137 ) ) ;
#19506=PRODUCT_DEFINITION ( 'UNKNOWN', '', #37055, #36495 ) ;
#19518=CARTESIAN_POINT ( 'NONE',  ( 2.940415233664778416, 20.44041523366473712, -35.99999999999996447 ) ) ;
#19539=CARTESIAN_POINT ( 'NONE',  ( -2.983759233219601903, 20.69971185032686023, -33.75704692567387610 ) ) ;
#19543=CARTESIAN_POINT ( 'NONE',  ( -0.7417250638684240727, 11.88857024925047057, -38.69295307432606279 ) ) ;
#19544=CARTESIAN_POINT ( 'NONE',  ( -0.7939530028709754772, 13.41554003082070246, -71.70704692567387895 ) ) ;
#19551=CARTESIAN_POINT ( 'NONE',  ( 4.107178604518054499, 18.15051318458946383, -42.29999999999996874 ) ) ;
#19554=CARTESIAN_POINT ( 'NONE',  ( -2.439449611014227859, 22.60758118029364283, -33.90704692567386758 ) ) ;
#19555=CARTESIAN_POINT ( 'NONE',  ( -2.701047200102606460, 12.19889638921340591, -28.34999999999996234 ) ) ;
#19556=CARTESIAN_POINT ( 'NONE',  ( -4.107178604518053611, 16.84948681541050775, -67.79999999999996874 ) ) ;
#19568=CARTESIAN_POINT ( 'NONE',  ( -0.7417250638684240727, 11.88857024925047057, -32.69295307432605568 ) ) ;
#19585=CARTESIAN_POINT ( 'NONE',  ( -4.318543150850367773, 18.18399003996480801, -28.94999999999996021 ) ) ;
#19586=CARTESIAN_POINT ( 'NONE',  ( 0.6839900399647733664, 13.18145684914961357, -58.04999999999996874 ) ) ;
#19595=CARTESIAN_POINT ( 'NONE',  ( 4.099003336600150149, 13.18504404629255689, -68.25704692567387610 ) ) ;
#19596=CARTESIAN_POINT ( 'NONE',  ( -5.876318620034919782, 18.43071743580290089, -58.94999999999996021 ) ) ;
#19610=CARTESIAN_POINT ( 'NONE',  ( -2.837105286290963146, 12.26822144673588255, -41.85704692567387752 ) ) ;
#19616=CARTESIAN_POINT ( 'NONE',  ( 0.7417250638684235176, 23.11142975074950101, -67.19295307432605568 ) ) ;
#19632=CARTESIAN_POINT ( 'NONE',  ( 2.701047200102605572, 22.80110361078655856, -44.84999999999996589 ) ) ;
#19635=CARTESIAN_POINT ( 'NONE',  ( 2.121074495332174958, 21.32648900066323350, -58.35704692567387752 ) ) ;
#19637=CARTESIAN_POINT ( 'NONE',  ( 3.895814058185739892, 19.48501640914376054, -51.14999999999996305 ) ) ;
#19649=CARTESIAN_POINT ( 'NONE',  ( 3.895814058185739448, 19.48501640914375344, -60.14999999999995595 ) ) ;
#19651=CARTESIAN_POINT ( 'NONE',  ( -3.965139115708213868, 15.65104167704456906, -45.15704692567388179 ) ) ;
#19655=CARTESIAN_POINT ( 'NONE',  ( 0.5070733663080689846, 21.62989723985679902, -40.19295307432605568 ) ) ;
#19661=CARTESIAN_POINT ( 'NONE',  ( -4.294655364005415699, 18.33481159033935626, -24.45704692567386829 ) ) ;
#19668=CARTESIAN_POINT ( 'NONE',  ( 5.041649132594343996, 14.93115145952162415, -45.59999999999996589 ) ) ;
#19680=EDGE_CURVE ( 'NONE', #4513, #2773, #15076, .T. ) ;
#19686=CARTESIAN_POINT ( 'NONE',  ( -4.103766977300021601, 13.60161616641083704, -24.00704692567387610 ) ) ;
#19692=CARTESIAN_POINT ( 'NONE',  ( 3.895814058185739448, 19.48501640914375344, -39.14999999999997016 ) ) ;
#19706=CARTESIAN_POINT ( 'NONE',  ( 3.199711850326839357, 14.51624076678035635, -50.24295307432605284 ) ) ;
#19711=CARTESIAN_POINT ( 'NONE',  ( 0.8348115903393232839, 13.20534463599456387, -62.54295307432605711 ) ) ;
#19723=CARTESIAN_POINT ( 'NONE',  ( -0.6839900399647736995, 21.81854315085035623, -35.54999999999994742 ) ) ;
#19749=CARTESIAN_POINT ( 'NONE',  ( 3.965139115708213868, 19.34895832295540430, -31.65704692567386402 ) ) ;
#19754=CARTESIAN_POINT ( 'NONE',  ( -5.107581180293630396, 19.93944961101426827, -36.59295307432605426 ) ) ;
#19755=CARTESIAN_POINT ( 'NONE',  ( -3.639207298612509689, 19.51726172033310647, -60.60704692567387752 ) ) ;
#19763=CARTESIAN_POINT ( 'NONE',  ( 3.091735541773220852, 14.40826445822673563, -45.74999999999995737 ) ) ;
#19765=CARTESIAN_POINT ( 'NONE',  ( -2.439449611014227859, 22.60758118029364283, -39.90704692567386758 ) ) ;
#19767=CARTESIAN_POINT ( 'NONE',  ( 1.887862790868997109, 13.79486065368817194, -60.89999999999997016 ) ) ;
#19780=CARTESIAN_POINT ( 'NONE',  ( 2.564989113914249330, 22.87042866830903876, -28.34295307432605426 ) ) ;
#19797=CARTESIAN_POINT ( 'NONE',  ( -4.318543150850367773, 18.18399003996480801, -55.94999999999997442 ) ) ;
#19806=CARTESIAN_POINT ( 'NONE',  ( -4.084459969179292216, 16.70604699712905372, -27.29295307432605355 ) ) ;
#19808=CARTESIAN_POINT ( 'NONE',  ( -4.975717084895059372, 20.19824746994243370, -69.60704692567387042 ) ) ;
#19809=CARTESIAN_POINT ( 'NONE',  ( -0.9307174358028534877, 23.37631862003491889, -53.54999999999996163 ) ) ;
#19822=CARTESIAN_POINT ( 'NONE',  ( -5.611429750749524992, 16.75827493613162034, -48.30704692567388037 ) ) ;
#19827=CARTESIAN_POINT ( 'NONE',  ( 5.565992480072003978, 18.52860470043125574, -64.79295307432606421 ) ) ;
#19843=CARTESIAN_POINT ( 'NONE',  ( 2.701047200102605572, 22.80110361078655856, -38.84999999999996589 ) ) ;
#19846=CARTESIAN_POINT ( 'NONE',  ( -2.983759233219601903, 20.69971185032686023, -51.75704692567388321 ) ) ;
#19847=CARTESIAN_POINT ( 'NONE',  ( -1.887862790868997553, 21.20513934631180319, -44.39999999999997016 ) ) ;
#19858=CARTESIAN_POINT ( 'NONE',  ( 4.318543150850367773, 16.81600996003516357, -51.44999999999997442 ) ) ;
#19860=CARTESIAN_POINT ( 'NONE',  ( 1.758463861404912620, 13.72892860598888731, -41.40704692567386758 ) ) ;
#19864=CARTESIAN_POINT ( 'NONE',  ( 4.084459969179292216, 18.29395300287091430, -34.79295307432605711 ) ) ;
#19872=CARTESIAN_POINT ( 'NONE',  ( -2.439449611014227859, 22.60758118029364283, -72.90704692567388179 ) ) ;
#19880=CARTESIAN_POINT ( 'NONE',  ( -5.301103610786608300, 14.79895279989743706, -34.64999999999997016 ) ) ;
#19901=CARTESIAN_POINT ( 'NONE',  ( 0.8851648821498760977, 23.08871111541074228, -74.69999999999997442 ) ) ;
#19906=CARTESIAN_POINT ( 'NONE',  ( 4.318543150850367773, 16.81600996003516357, -36.44999999999996732 ) ) ;
#19919=CARTESIAN_POINT ( 'NONE',  ( 0.5070733663080689846, 21.62989723985679902, -49.19295307432605568 ) ) ;
#19924=CARTESIAN_POINT ( 'NONE',  ( 0.8348115903393232839, 13.20534463599456387, -59.54295307432605711 ) ) ;
#19936=CARTESIAN_POINT ( 'NONE',  ( -0.6839900399647736995, 21.81854315085035623, -29.54999999999996518 ) ) ;
#19944=CARTESIAN_POINT ( 'NONE',  ( -0.8851648821498765418, 11.91128888458923285, -64.19999999999996021 ) ) ;
#19962=CARTESIAN_POINT ( 'NONE',  ( -2.564989113914250662, 12.12957133169093282, -68.84295307432606137 ) ) ;
#19966=CARTESIAN_POINT ( 'NONE',  ( 3.639207298612508801, 15.48273827966686866, -38.10704692567387752 ) ) ;
#19970=CARTESIAN_POINT ( 'NONE',  ( 3.771071394011080269, 15.74153613859503764, -71.09295307432604716 ) ) ;
#19971=CARTESIAN_POINT ( 'NONE',  ( -2.121074495332175847, 13.67351099933674341, -59.85704692567387752 ) ) ;
#19981=CARTESIAN_POINT ( 'NONE',  ( -3.705139346311794313, 19.38786279086902198, -41.09999999999996589 ) ) ;
#19984=CARTESIAN_POINT ( 'NONE',  ( 2.439449611014226971, 12.39241881970633230, -29.40704692567386758 ) ) ;
#19986=CARTESIAN_POINT ( 'NONE',  ( -2.940415233664778860, 14.55958476633523802, -58.49999999999997158 ) ) ;
#19999=CARTESIAN_POINT ( 'NONE',  ( -5.107581180293630396, 19.93944961101426827, -36.59295307432605426 ) ) ;
#20017=CARTESIAN_POINT ( 'NONE',  ( -1.985016409143819605, 13.60418594181426855, -49.34999999999996589 ) ) ;
#20027=CARTESIAN_POINT ( 'NONE',  ( -3.771071394011080269, 19.25846386140493394, -30.59295307432605782 ) ) ;
#20029=CARTESIAN_POINT ( 'NONE',  ( 4.099003336600150149, 13.18504404629255689, -59.25704692567388321 ) ) ;
#20030=CARTESIAN_POINT ( 'NONE',  ( 4.206979645153768210, 13.29302035484617406, -42.74999999999997158 ) ) ;
#20045=CARTESIAN_POINT ( 'NONE',  ( 2.439449611014226971, 12.39241881970633230, -44.40704692567387468 ) ) ;
#20049=CARTESIAN_POINT ( 'NONE',  ( 5.107581180293630396, 15.06055038898570686, -65.09295307432604716 ) ) ;
#20065=CARTESIAN_POINT ( 'NONE',  ( 0.8851648821498760977, 23.08871111541074228, -29.69999999999996376 ) ) ;
#20068=CARTESIAN_POINT ( 'NONE',  ( -4.129897239856814117, 16.99292663369196177, -51.30704692567388037 ) ) ;
#20069=CARTESIAN_POINT ( 'NONE',  ( -2.940415233664778860, 14.55958476633523802, -34.49999999999997158 ) ) ;
#20070=CARTESIAN_POINT ( 'NONE',  ( -0.6505131845895224529, 13.39282139548194195, -73.19999999999997442 ) ) ;
#20077=CARTESIAN_POINT ( 'NONE',  ( 0.6505131845895220088, 21.60717860451803674, -50.69999999999996732 ) ) ;
#20079=CARTESIAN_POINT ( 'NONE',  ( 2.983759233219601459, 14.30028814967311668, -41.25704692567387610 ) ) ;
#20080=CARTESIAN_POINT ( 'NONE',  ( -5.041649132594344884, 20.06884854047834921, -74.09999999999996589 ) ) ;
#20083=CARTESIAN_POINT ( 'NONE',  ( -4.084459969179292216, 16.70604699712905372, -39.29295307432605711 ) ) ;
#20089=CARTESIAN_POINT ( 'NONE',  ( 1.028604700431328567, 23.06599248007198355, -73.20704692567387895 ) ) ;
#20096=CARTESIAN_POINT ( 'NONE',  ( 5.301103610786608300, 20.20104720010253985, -42.14999999999996305 ) ) ;
#20114=CARTESIAN_POINT ( 'NONE',  ( -0.9307174358028533767, 23.37631862003491889, -56.54999999999996874 ) ) ;
#20119=CARTESIAN_POINT ( 'NONE',  ( 0.6505131845895220088, 21.60717860451803674, -32.69999999999996732 ) ) ;
#20132=CARTESIAN_POINT ( 'NONE',  ( -2.017261720333081598, 21.13920729861251857, -48.89295307432605853 ) ) ;
#20138=CARTESIAN_POINT ( 'NONE',  ( 3.771071394011080269, 15.74153613859503764, -62.09295307432606847 ) ) ;
#20150=CARTESIAN_POINT ( 'NONE',  ( -3.091735541773221296, 20.59173554177323950, -26.24999999999996803 ) ) ;
#20159=CARTESIAN_POINT ( 'NONE',  ( 4.001075405444606048, 21.50107540544455276, -71.99999999999997158 ) ) ;
#20176=CARTESIAN_POINT ( 'NONE',  ( 4.314955953707388936, 13.40099666339979123, -65.24295307432606705 ) ) ;
#20184=CARTESIAN_POINT ( 'NONE',  ( 4.084459969179292216, 18.29395300287091430, -73.79295307432605000 ) ) ;
#20186=CARTESIAN_POINT ( 'NONE',  ( -1.758463861404912842, 21.27107139401109137, -60.90704692567388179 ) ) ;
#20198=CARTESIAN_POINT ( 'NONE',  ( -5.852430833189966819, 18.58153898617744915, -30.45704692567387184 ) ) ;
#20199=CARTESIAN_POINT ( 'NONE',  ( -1.985016409143819605, 13.60418594181426855, -55.34999999999997300 ) ) ;
#20210=CARTESIAN_POINT ( 'NONE',  ( -5.565992480072003978, 16.47139529956871229, -36.29295307432605000 ) ) ;
#20229=CARTESIAN_POINT ( 'NONE',  ( -3.895814058185739448, 15.51498359085620571, -49.64999999999995595 ) ) ;
#20239=CARTESIAN_POINT ( 'NONE',  ( 0.6505131845895220088, 21.60717860451803674, -68.69999999999997442 ) ) ;
#20241=CARTESIAN_POINT ( 'NONE',  ( 4.975717084895059372, 14.80175253005754143, -56.10704692567387752 ) ) ;
#20242=CARTESIAN_POINT ( 'NONE',  ( 2.701047200102605128, 22.80110361078656211, -41.84999999999996589 ) ) ;
#20253=CARTESIAN_POINT ( 'NONE',  ( -5.370428668309080500, 14.93501088608579153, -45.15704692567388179 ) ) ;
#20257=CARTESIAN_POINT ( 'NONE',  ( -5.107581180293630396, 19.93944961101426827, -57.59295307432605426 ) ) ;
#20271=CARTESIAN_POINT ( 'NONE',  ( 5.301103610786608300, 20.20104720010253985, -30.14999999999997016 ) ) ;
#20275=CARTESIAN_POINT ( 'NONE',  ( 0.7939530028709752552, 21.58445996917927445, -55.20704692567388605 ) ) ;
#20284=CARTESIAN_POINT ( 'NONE',  ( 1.887862790868997109, 13.79486065368817194, -51.89999999999997016 ) ) ;
#20286=CARTESIAN_POINT ( 'NONE',  ( -1.758463861404912842, 21.27107139401109137, -30.90704692567387113 ) ) ;
#20290=CARTESIAN_POINT ( 'NONE',  ( -4.342430937695320736, 18.03316848959025620, -39.44295307432604858 ) ) ;
#20297=CARTESIAN_POINT ( 'NONE',  ( 4.294655364005415699, 16.66518840966061887, -28.95704692567387184 ) ) ;
#20303=CARTESIAN_POINT ( 'NONE',  ( 5.876318620034919782, 16.56928256419707068, -39.44999999999994600 ) ) ;
#20321=CARTESIAN_POINT ( 'NONE',  ( -4.001075405444606936, 13.49892459455542060, -64.49999999999997158 ) ) ;
#20327=CARTESIAN_POINT ( 'NONE',  ( 2.940415233664778416, 20.44041523366473712, -35.99999999999996447 ) ) ;
#20328=CARTESIAN_POINT ( 'NONE',  ( -1.887862790868997553, 21.20513934631180319, -68.39999999999997726 ) ) ;
#20339=CARTESIAN_POINT ( 'NONE',  ( -4.342430937695320736, 18.03316848959025620, -48.44295307432605568 ) ) ;
#20345=CARTESIAN_POINT ( 'NONE',  ( -0.5070733663080690956, 13.37010276014318144, -65.69295307432605568 ) ) ;
#20356=CARTESIAN_POINT ( 'NONE',  ( -2.940415233664778860, 14.55958476633523802, -31.49999999999996447 ) ) ;
#20365=CARTESIAN_POINT ( 'NONE',  ( 5.301103610786608300, 20.20104720010253985, -69.14999999999994884 ) ) ;
#20383=CARTESIAN_POINT ( 'NONE',  ( -0.7417250638684240727, 11.88857024925047057, -53.69295307432606279 ) ) ;
#20394=CARTESIAN_POINT ( 'NONE',  ( -3.199711850326840246, 20.48375923321962233, -72.74295307432603863 ) ) ;
#20396=CARTESIAN_POINT ( 'NONE',  ( -2.983759233219601903, 20.69971185032686023, -63.75704692567388321 ) ) ;
#20408=CARTESIAN_POINT ( 'NONE',  ( 1.028604700431328567, 23.06599248007198355, -31.20704692567387539 ) ) ;
#20410=CARTESIAN_POINT ( 'NONE',  ( -4.318543150850367773, 18.18399003996480801, -55.94999999999997442 ) ) ;
#20424=CARTESIAN_POINT ( 'NONE',  ( 2.564989113914249330, 22.87042866830903876, -34.34295307432605426 ) ) ;
#20441=CARTESIAN_POINT ( 'NONE',  ( 3.091735541773220852, 14.40826445822673563, -48.74999999999997158 ) ) ;
#20452=CARTESIAN_POINT ( 'NONE',  ( 0.6839900399647733664, 13.18145684914961357, -67.04999999999994031 ) ) ;
#20454=CARTESIAN_POINT ( 'NONE',  ( -1.028604700431329233, 11.93400751992799513, -56.70704692567387184 ) ) ;
#20455=CARTESIAN_POINT ( 'NONE',  ( 2.701047200102605128, 22.80110361078656211, -44.84999999999996589 ) ) ;
#20469=CARTESIAN_POINT ( 'NONE',  ( 1.028604700431328567, 23.06599248007198355, -49.20704692567387184 ) ) ;
#20474=CARTESIAN_POINT ( 'NONE',  ( 5.231778553264135212, 20.33710528629089254, -61.64295307432606563 ) ) ;
#20489=CARTESIAN_POINT ( 'NONE',  ( -5.876318620034919782, 18.43071743580290089, -28.94999999999996021 ) ) ;
#20492=CARTESIAN_POINT ( 'NONE',  ( -3.043106805520194413, 14.66227633819065623, -57.00704692567387610 ) ) ;
#20493=CARTESIAN_POINT ( 'NONE',  ( -3.895814058185739448, 15.51498359085620571, -73.64999999999993463 ) ) ;
#20499=CARTESIAN_POINT ( 'NONE',  ( 1.985016409143818272, 21.39581405818570303, -53.84999999999995879 ) ) ;
#20501=CARTESIAN_POINT ( 'NONE',  ( -0.7939530028709754772, 13.41554003082070246, -38.70704692567387184 ) ) ;
#20502=CARTESIAN_POINT ( 'NONE',  ( 0.9307174358028527106, 11.62368137996505801, -73.04999999999998295 ) ) ;
#20506=CARTESIAN_POINT ( 'NONE',  ( -4.342430937695320736, 18.03316848959025620, -33.44295307432605568 ) ) ;
#20513=CARTESIAN_POINT ( 'NONE',  ( 5.611429750749524992, 18.24172506386835479, -70.80704692567387326 ) ) ;
#20518=CARTESIAN_POINT ( 'NONE',  ( -0.8851648821498765418, 11.91128888458923285, -43.19999999999996732 ) ) ;
#20535=CARTESIAN_POINT ( 'NONE',  ( -5.588711115410763597, 16.61483511785016987, -61.79999999999996874 ) ) ;
#20540=CARTESIAN_POINT ( 'NONE',  ( 1.887862790868997109, 13.79486065368817194, -30.89999999999996305 ) ) ;
#20541=CARTESIAN_POINT ( 'NONE',  ( -3.895814058185739892, 15.51498359085620748, -70.64999999999996305 ) ) ;
#20553=CARTESIAN_POINT ( 'NONE',  ( -1.848958322955462474, 13.53486088429179546, -47.84295307432606137 ) ) ;
#20559=CARTESIAN_POINT ( 'NONE',  ( 4.084459969179292216, 18.29395300287091430, -64.79295307432606421 ) ) ;
#20578=CARTESIAN_POINT ( 'NONE',  ( 4.001075405444606048, 21.50107540544455276, -68.99999999999995737 ) ) ;
#20598=CARTESIAN_POINT ( 'NONE',  ( -5.231778553264134324, 14.66289471370907727, -51.14295307432606563 ) ) ;
#20605=CARTESIAN_POINT ( 'NONE',  ( 3.826489000663266360, 19.62107449533211678, -70.64295307432605853 ) ) ;
#20607=CARTESIAN_POINT ( 'NONE',  ( -3.639207298612509689, 19.51726172033310647, -66.60704692567387042 ) ) ;
#20620=CARTESIAN_POINT ( 'NONE',  ( 5.370428668309080500, 20.06498911391418360, -28.65704692567387468 ) ) ;
#20622=CARTESIAN_POINT ( 'NONE',  ( 4.107178604518054499, 18.15051318458946383, -51.29999999999996874 ) ) ;
#20634=CARTESIAN_POINT ( 'NONE',  ( 3.771071394011080269, 15.74153613859503764, -74.09295307432606137 ) ) ;
#20654=CARTESIAN_POINT ( 'NONE',  ( -3.470745319554693342, 14.02925468044533019, -25.49999999999996803 ) ) ;
#20655=CARTESIAN_POINT ( 'NONE',  ( 1.887862790868997109, 13.79486065368817194, -48.89999999999997016 ) ) ;
#20664=CARTESIAN_POINT ( 'NONE',  ( 0.6839900399647733664, 13.18145684914961357, -64.04999999999994031 ) ) ;
#20666=CARTESIAN_POINT ( 'NONE',  ( 5.370428668309080500, 20.06498911391418360, -55.65704692567387468 ) ) ;
#20667=CARTESIAN_POINT ( 'NONE',  ( 4.001075405444606048, 21.50107540544455276, -47.99999999999996447 ) ) ;
#20682=CARTESIAN_POINT ( 'NONE',  ( -5.611429750749524992, 16.75827493613162034, -39.30704692567388037 ) ) ;
#20686=CARTESIAN_POINT ( 'NONE',  ( 1.081538986177402295, 11.64756916681001186, -47.54295307432606421 ) ) ;
#20703=CARTESIAN_POINT ( 'NONE',  ( -2.701047200102606016, 12.19889638921340413, -34.34999999999995879 ) ) ;
#20706=CARTESIAN_POINT ( 'NONE',  ( -0.5331684895902242260, 21.84243093769531185, -49.05704692567388037 ) ) ;
#20707=CARTESIAN_POINT ( 'NONE',  ( -2.940415233664778860, 14.55958476633523802, -73.49999999999997158 ) ) ;
#20716=CARTESIAN_POINT ( 'NONE',  ( 0.6839900399647733664, 13.18145684914961357, -58.04999999999996874 ) ) ;
#20718=CARTESIAN_POINT ( 'NONE',  ( -4.129897239856814117, 16.99292663369196177, -33.30704692567387326 ) ) ;
#20719=CARTESIAN_POINT ( 'NONE',  ( 0.8851648821498760977, 23.08871111541074228, -71.69999999999997442 ) ) ;
#20730=CARTESIAN_POINT ( 'NONE',  ( 5.370428668309080500, 20.06498911391418360, -67.65704692567386758 ) ) ;
#20736=CARTESIAN_POINT ( 'NONE',  ( -4.001075405444606936, 13.49892459455542060, -40.49999999999996447 ) ) ;
#20754=CARTESIAN_POINT ( 'NONE',  ( 0.9307174358028528216, 11.62368137996505801, -64.04999999999994031 ) ) ;
#20760=CARTESIAN_POINT ( 'NONE',  ( -3.895814058185739448, 15.51498359085620571, -34.64999999999997016 ) ) ;
#20761=CARTESIAN_POINT ( 'NONE',  ( -0.6505131845895224529, 13.39282139548194195, -70.19999999999997442 ) ) ;
#20772=CARTESIAN_POINT ( 'NONE',  ( -3.826489000663265472, 15.37892550466785480, -33.14295307432605853 ) ) ;
#20777=CARTESIAN_POINT ( 'NONE',  ( -0.5070733663080690956, 13.37010276014318144, -53.69295307432606279 ) ) ;
#20794=CARTESIAN_POINT ( 'NONE',  ( -5.876318620034919782, 18.43071743580290089, -67.94999999999994600 ) ) ;
#20798=ORIENTED_EDGE ( 'NONE', *, *, #12300, .T. ) ;
#20812=CARTESIAN_POINT ( 'NONE',  ( -5.107581180293630396, 19.93944961101426827, -57.59295307432605426 ) ) ;
#20821=CARTESIAN_POINT ( 'NONE',  ( -4.342430937695320736, 18.03316848959025620, -72.44295307432605568 ) ) ;
#20823=CARTESIAN_POINT ( 'NONE',  ( -2.121074495332175847, 13.67351099933674341, -56.85704692567387042 ) ) ;
#20835=CARTESIAN_POINT ( 'NONE',  ( -0.6839900399647736995, 21.81854315085035623, -56.54999999999996874 ) ) ;
#20844=CARTESIAN_POINT ( 'NONE',  ( 3.826489000663266360, 19.62107449533211678, -73.64295307432605853 ) ) ;
#20856=CARTESIAN_POINT ( 'NONE',  ( -0.6839900399647738105, 21.81854315085035623, -35.54999999999995453 ) ) ;
#20862=CARTESIAN_POINT ( 'NONE',  ( 3.091735541773220852, 14.40826445822673563, -42.74999999999996447 ) ) ;
#20872=CARTESIAN_POINT ( 'NONE',  ( -3.091735541773221296, 20.59173554177323950, -62.24999999999995737 ) ) ;
#20873=CARTESIAN_POINT ( 'NONE',  ( -5.611429750749524992, 16.75827493613162034, -57.30704692567387326 ) ) ;
#20874=CARTESIAN_POINT ( 'NONE',  ( -2.701047200102606460, 12.19889638921340591, -46.34999999999997300 ) ) ;
#20887=CARTESIAN_POINT ( 'NONE',  ( -4.103766977300021601, 13.60161616641083704, -36.00704692567386189 ) ) ;
#20890=CARTESIAN_POINT ( 'NONE',  ( -1.081538986177402961, 23.35243083318996327, -52.04295307432606421 ) ) ;
#20906=CARTESIAN_POINT ( 'NONE',  ( -5.107581180293630396, 19.93944961101426827, -69.59295307432604716 ) ) ;
#20909=CARTESIAN_POINT ( 'NONE',  ( 4.294655364005415699, 16.66518840966061887, -46.95704692567387184 ) ) ;
#20910=CARTESIAN_POINT ( 'NONE',  ( -0.6839900399647736995, 21.81854315085035623, -71.54999999999994031 ) ) ;
#20917=CARTESIAN_POINT ( 'NONE',  ( 4.318543150850367773, 16.81600996003516357, -48.44999999999994600 ) ) ;
#20920=CARTESIAN_POINT ( 'NONE',  ( -2.983759233219601903, 20.69971185032686023, -33.75704692567387610 ) ) ;
#20921=CARTESIAN_POINT ( 'NONE',  ( -5.588711115410763597, 16.61483511785016987, -70.79999999999996874 ) ) ;
#20933=CARTESIAN_POINT ( 'NONE',  ( 2.837105286290961370, 22.73177855326409613, -64.35704692567387042 ) ) ;
#20937=CARTESIAN_POINT ( 'NONE',  ( 0.9307174358028528216, 11.62368137996505801, -31.04999999999995808 ) ) ;
#20956=CARTESIAN_POINT ( 'NONE',  ( -5.876318620034919782, 18.43071743580290089, -61.94999999999997442 ) ) ;
#20960=CARTESIAN_POINT ( 'NONE',  ( 1.758463861404912620, 13.72892860598888731, -68.40704692567388179 ) ) ;
#20961=CARTESIAN_POINT ( 'NONE',  ( -3.895814058185739892, 15.51498359085620748, -64.64999999999996305 ) ) ;
#20971=CARTESIAN_POINT ( 'NONE',  ( 3.199711850326839357, 14.51624076678035635, -38.24295307432604574 ) ) ;
#20975=CARTESIAN_POINT ( 'NONE',  ( 4.084459969179292216, 18.29395300287091430, -55.79295307432606421 ) ) ;
#20993=CARTESIAN_POINT ( 'NONE',  ( 5.301103610786608300, 20.20104720010253985, -54.14999999999997726 ) ) ;
#21007=ADVANCED_FACE ( 'NONE', ( #18615 ), #13561, .T. ) ;
#21012=CARTESIAN_POINT ( 'NONE',  ( -5.565992480072003978, 16.47139529956871229, -57.29295307432606421 ) ) ;
#21021=CARTESIAN_POINT ( 'NONE',  ( 4.342430937695320736, 16.96683151040971538, -61.94295307432605568 ) ) ;
#21023=CARTESIAN_POINT ( 'NONE',  ( 1.758463861404912620, 13.72892860598888731, -53.40704692567386758 ) ) ;
#21036=CARTESIAN_POINT ( 'NONE',  ( 4.318543150850367773, 16.81600996003516357, -42.44999999999996732 ) ) ;
#21048=CARTESIAN_POINT ( 'NONE',  ( -0.8348115903393239501, 21.79465536400541126, -73.04295307432606421 ) ) ;
#21052=EDGE_LOOP ( 'NONE', ( #36800, #6815 ) ) ;
#21062=CARTESIAN_POINT ( 'NONE',  ( 3.895814058185739892, 19.48501640914376054, -39.14999999999997016 ) ) ;
#21067=CARTESIAN_POINT ( 'NONE',  ( 1.887862790868997109, 13.79486065368817194, -39.89999999999996305 ) ) ;
#21077=CARTESIAN_POINT ( 'NONE',  ( 4.107178604518054499, 18.15051318458946383, -63.29999999999996874 ) ) ;
#21079=CARTESIAN_POINT ( 'NONE',  ( -2.439449611014227859, 22.60758118029364283, -42.90704692567387468 ) ) ;
#21080=CARTESIAN_POINT ( 'NONE',  ( -0.8851648821498765418, 11.91128888458923285, -37.19999999999996732 ) ) ;
#21093=CARTESIAN_POINT ( 'NONE',  ( -4.103766977300021601, 13.60161616641083704, -33.00704692567387610 ) ) ;
#21097=CARTESIAN_POINT ( 'NONE',  ( -2.564989113914250662, 12.12957133169093282, -53.84295307432606137 ) ) ;
#21115=CARTESIAN_POINT ( 'NONE',  ( 5.565992480072003978, 18.52860470043125574, -73.79295307432605000 ) ) ;
#21118=CARTESIAN_POINT ( 'NONE',  ( 3.639207298612508801, 15.48273827966686866, -44.10704692567387752 ) ) ;
#21119=CARTESIAN_POINT ( 'NONE',  ( 2.940415233664778416, 20.44041523366473712, -62.99999999999997158 ) ) ;
#21128=CARTESIAN_POINT ( 'NONE',  ( -4.294655364005415699, 18.33481159033935626, -33.45704692567387895 ) ) ;
#21129=CARTESIAN_POINT ( 'NONE',  ( 2.568848540478311460, 12.45835086740561692, -63.89999999999997016 ) ) ;
#21140=CARTESIAN_POINT ( 'NONE',  ( -2.439449611014227859, 22.60758118029364283, -66.90704692567388179 ) ) ;
#21143=CARTESIAN_POINT ( 'NONE',  ( -2.568848540478311904, 22.54164913259435465, -32.39999999999996305 ) ) ;
#21159=CARTESIAN_POINT ( 'NONE',  ( -2.568848540478311904, 22.54164913259435465, -53.39999999999997016 ) ) ;
#21163=CARTESIAN_POINT ( 'NONE',  ( 3.965139115708213868, 19.34895832295540430, -67.65704692567386758 ) ) ;
#21164=CARTESIAN_POINT ( 'NONE',  ( -1.887862790868997553, 21.20513934631180319, -65.39999999999997726 ) ) ;
#21170=CARTESIAN_POINT ( 'NONE',  ( -0.6505131845895224529, 13.39282139548194195, -70.19999999999997442 ) ) ;
#21174=CARTESIAN_POINT ( 'NONE',  ( -1.848958322955462474, 13.53486088429179546, -32.84295307432606137 ) ) ;
#21177=CARTESIAN_POINT ( 'NONE',  ( -2.837723661809363751, 14.45689319447982335, -53.99295307432605995 ) ) ;
#21196=APPLICATION_CONTEXT ( 'automotive_design' ) ;
#21197=CARTESIAN_POINT ( 'NONE',  ( -2.701047200102606016, 12.19889638921340413, -58.34999999999995879 ) ) ;
#21220=CARTESIAN_POINT ( 'NONE',  ( 2.564989113914249330, 22.87042866830903876, -55.34295307432606137 ) ) ;
#21228=CARTESIAN_POINT ( 'NONE',  ( -2.017261720333081598, 21.13920729861251857, -69.89295307432607274 ) ) ;
#21230=CARTESIAN_POINT ( 'NONE',  ( 4.129897239856814117, 18.00707336630801336, -55.80704692567388037 ) ) ;
#21242=CARTESIAN_POINT ( 'NONE',  ( -3.091735541773221296, 20.59173554177323950, -41.24999999999995026 ) ) ;
#21256=CARTESIAN_POINT ( 'NONE',  ( -3.199711850326840246, 20.48375923321962233, -69.74295307432603863 ) ) ;
#21269=CARTESIAN_POINT ( 'NONE',  ( -4.318543150850366885, 18.18399003996480801, -34.94999999999996732 ) ) ;
#21276=CARTESIAN_POINT ( 'NONE',  ( -4.107178604518053611, 16.84948681541050775, -34.79999999999996163 ) ) ;
#21285=CARTESIAN_POINT ( 'NONE',  ( 0.6505131845895220088, 21.60717860451803674, -56.69999999999997442 ) ) ;
#21288=CARTESIAN_POINT ( 'NONE',  ( -4.975717084895059372, 20.19824746994243370, -45.60704692567387752 ) ) ;
#21289=CARTESIAN_POINT ( 'NONE',  ( 5.301103610786608300, 20.20104720010254340, -33.14999999999996305 ) ) ;
#21292=CARTESIAN_POINT ( 'NONE',  ( 0.8348115903393232839, 13.20534463599456387, -29.54295307432605355 ) ) ;
#21302=CARTESIAN_POINT ( 'NONE',  ( 2.439449611014226971, 12.39241881970633230, -32.40704692567386758 ) ) ;
#21304=CARTESIAN_POINT ( 'NONE',  ( -2.564989113914250662, 12.12957133169093282, -47.84295307432606137 ) ) ;
#21322=CARTESIAN_POINT ( 'NONE',  ( -5.107581180293630396, 19.93944961101426827, -75.59295307432606137 ) ) ;
#21325=CARTESIAN_POINT ( 'NONE',  ( -0.5331684895902242260, 21.84243093769531185, -43.05704692567387326 ) ) ;
#21326=CARTESIAN_POINT ( 'NONE',  ( -2.940415233664778860, 14.55958476633523802, -37.49999999999996447 ) ) ;
#21327=CARTESIAN_POINT ( 'NONE',  ( 1.985016409143818272, 21.39581405818570303, -65.84999999999992326 ) ) ;
#21338=CARTESIAN_POINT ( 'NONE',  ( -0.5331684895902242260, 21.84243093769531185, -25.05704692567386971 ) ) ;
#21339=CARTESIAN_POINT ( 'NONE',  ( 5.041649132594343996, 14.93115145952162415, -63.59999999999995879 ) ) ;
#21341=DIRECTION ( 'NONE',  ( -0.7037848285661852943, 0.7037848285661921777, 0.09681854243955874406 ) ) ;
#21351=CARTESIAN_POINT ( 'NONE',  ( -2.837105286290963146, 12.26822144673588255, -59.85704692567387752 ) ) ;
#21355=CARTESIAN_POINT ( 'NONE',  ( -2.568848540478311904, 22.54164913259435465, -26.39999999999996660 ) ) ;
#21368=CARTESIAN_POINT ( 'NONE',  ( 4.206979645153767322, 13.29302035484617051, -54.74999999999997158 ) ) ;
#21372=CARTESIAN_POINT ( 'NONE',  ( 3.895814058185739448, 19.48501640914375344, -27.14999999999995595 ) ) ;
#21373=CARTESIAN_POINT ( 'NONE',  ( -1.887862790868997553, 21.20513934631180319, -53.39999999999997016 ) ) ;
#21384=CARTESIAN_POINT ( 'NONE',  ( 2.017261720333081598, 13.86079270138745834, -35.39295307432605142 ) ) ;
#21386=CARTESIAN_POINT ( 'NONE',  ( 3.771071394011080269, 15.74153613859503764, -50.09295307432605426 ) ) ;
#21403=CARTESIAN_POINT ( 'NONE',  ( 5.876318620034919782, 16.56928256419707068, -57.44999999999996732 ) ) ;
#21424=CARTESIAN_POINT ( 'NONE',  ( 2.698247469942395949, 12.52428291510489977, -41.39295307432605853 ) ) ;
#21436=CARTESIAN_POINT ( 'NONE',  ( 3.826489000663266360, 19.62107449533211678, -67.64295307432605853 ) ) ;
#21449=CARTESIAN_POINT ( 'NONE',  ( 4.107178604518054499, 18.15051318458946383, -42.29999999999996874 ) ) ;
#21475=CARTESIAN_POINT ( 'NONE',  ( 4.107178604518054499, 18.15051318458946383, -39.29999999999996874 ) ) ;
#21479=CARTESIAN_POINT ( 'NONE',  ( 0.6505131845895220088, 21.60717860451803674, -35.69999999999996732 ) ) ;
#21488=CARTESIAN_POINT ( 'NONE',  ( -0.6505131845895224529, 13.39282139548194195, -58.19999999999996732 ) ) ;
#21490=CARTESIAN_POINT ( 'NONE',  ( 5.370428668309080500, 20.06498911391418360, -49.65704692567388179 ) ) ;
#21491=CARTESIAN_POINT ( 'NONE',  ( -0.8851648821498765418, 11.91128888458923285, -34.19999999999996732 ) ) ;
#21492=CARTESIAN_POINT ( 'NONE',  ( 3.898383833589191383, 21.60376697729997275, -40.49295307432605995 ) ) ;
#21495=CARTESIAN_POINT ( 'NONE',  ( 1.848958322955461808, 21.46513911570817612, -28.34295307432605426 ) ) ;
#21505=CARTESIAN_POINT ( 'NONE',  ( -0.7798958854283041253, 23.40020640687986386, -31.05704692567387681 ) ) ;
#21512=CARTESIAN_POINT ( 'NONE',  ( 5.231778553264135212, 20.33710528629089254, -46.64295307432605853 ) ) ;
#21531=CARTESIAN_POINT ( 'NONE',  ( -3.898383833589191827, 13.39623302270000771, -71.99295307432603863 ) ) ;
#21535=CARTESIAN_POINT ( 'NONE',  ( 0.7939530028709752552, 21.58445996917927445, -40.20704692567387184 ) ) ;
#21536=CARTESIAN_POINT ( 'NONE',  ( 3.091735541773220852, 14.40826445822673563, -30.74999999999995737 ) ) ;
#21537=CARTESIAN_POINT ( 'NONE',  ( -3.895814058185739448, 15.51498359085620571, -61.64999999999995595 ) ) ;
#21545=CARTESIAN_POINT ( 'NONE',  ( -4.129897239856814117, 16.99292663369196177, -27.30704692567386971 ) ) ;
#21546=CARTESIAN_POINT ( 'NONE',  ( -5.041649132594344884, 20.06884854047834921, -62.09999999999996589 ) ) ;
#21556=CARTESIAN_POINT ( 'NONE',  ( 4.975717084895059372, 14.80175253005754143, -62.10704692567388463 ) ) ;
#21560=CARTESIAN_POINT ( 'NONE',  ( -4.001075405444606936, 13.49892459455542060, -31.49999999999996447 ) ) ;
#21576=CARTESIAN_POINT ( 'NONE',  ( 4.206979645153767322, 13.29302035484617051, -48.74999999999997158 ) ) ;
#21580=CARTESIAN_POINT ( 'NONE',  ( -4.129897239856814117, 16.99292663369196177, -69.30704692567387326 ) ) ;
#21581=CARTESIAN_POINT ( 'NONE',  ( 4.318543150850366885, 16.81600996003516713, -60.44999999999996732 ) ) ;
#21587=CARTESIAN_POINT ( 'NONE',  ( 2.940415233664778416, 20.44041523366473712, -71.99999999999997158 ) ) ;
#21591=CARTESIAN_POINT ( 'NONE',  ( -3.199711850326840246, 20.48375923321962233, -39.74295307432605995 ) ) ;
#21594=CARTESIAN_POINT ( 'NONE',  ( -2.017261720333081598, 21.13920729861251857, -51.89295307432605853 ) ) ;
#21597=VERTEX_POINT ( 'NONE', #3887 ) ;
#21609=CARTESIAN_POINT ( 'NONE',  ( -4.001075405444606936, 13.49892459455542060, -58.49999999999997158 ) ) ;
#21628=CARTESIAN_POINT ( 'NONE',  ( -5.107581180293630396, 19.93944961101426827, -48.59295307432606847 ) ) ;
#21636=CARTESIAN_POINT ( 'NONE',  ( -3.771071394011080269, 19.25846386140493394, -69.59295307432604716 ) ) ;
#21651=CARTESIAN_POINT ( 'NONE',  ( 3.705139346311793869, 15.61213720913094960, -45.59999999999996589 ) ) ;
#21680=CARTESIAN_POINT ( 'NONE',  ( 2.940415233664778416, 20.44041523366473712, -32.99999999999996447 ) ) ;
#21684=CARTESIAN_POINT ( 'NONE',  ( 4.318543150850367773, 16.81600996003516357, -33.44999999999994600 ) ) ;
#21692=CARTESIAN_POINT ( 'NONE',  ( -3.705139346311794313, 19.38786279086902198, -53.09999999999996589 ) ) ;
#21693=CARTESIAN_POINT ( 'NONE',  ( 0.7798958854283032371, 11.59979359312010772, -50.55704692567388747 ) ) ;
#21694=CARTESIAN_POINT ( 'NONE',  ( -2.701047200102606460, 12.19889638921340591, -34.34999999999996589 ) ) ;
#21696=CARTESIAN_POINT ( 'NONE',  ( -4.107178604518053611, 16.84948681541050775, -70.79999999999996874 ) ) ;
#21710=CARTESIAN_POINT ( 'NONE',  ( 2.439449611014226971, 12.39241881970633230, -29.40704692567386758 ) ) ;
#21717=CARTESIAN_POINT ( 'NONE',  ( -3.898383833589191827, 13.39623302270000771, -38.99295307432604574 ) ) ;
#21734=CARTESIAN_POINT ( 'NONE',  ( -2.698247469942396837, 22.47571708489507358, -69.89295307432607274 ) ) ;
#21738=CARTESIAN_POINT ( 'NONE',  ( 4.318543150850367773, 16.81600996003516357, -36.44999999999996732 ) ) ;
#21739=CARTESIAN_POINT ( 'NONE',  ( 3.091735541773220852, 14.40826445822673563, -66.74999999999997158 ) ) ;
#21751=CARTESIAN_POINT ( 'NONE',  ( -4.294655364005415699, 18.33481159033935626, -24.45704692567386829 ) ) ;
#21752=CARTESIAN_POINT ( 'NONE',  ( 0.9307174358028527106, 11.62368137996505801, -64.04999999999995453 ) ) ;
#21764=CARTESIAN_POINT ( 'NONE',  ( -4.975717084895059372, 20.19824746994243370, -57.60704692567387752 ) ) ;
#21769=CARTESIAN_POINT ( 'NONE',  ( 5.041649132594343996, 14.93115145952162415, -27.59999999999996589 ) ) ;
#21785=CARTESIAN_POINT ( 'NONE',  ( 2.701047200102605572, 22.80110361078655856, -53.84999999999995879 ) ) ;
#21789=CARTESIAN_POINT ( 'NONE',  ( 4.294655364005415699, 16.66518840966061887, -70.95704692567389316 ) ) ;
#21790=CARTESIAN_POINT ( 'NONE',  ( 2.940415233664778416, 20.44041523366473712, -59.99999999999997158 ) ) ;
#21804=CARTESIAN_POINT ( 'NONE',  ( -2.837723661809363751, 14.45689319447982335, -26.99295307432605995 ) ) ;
#21807=CARTESIAN_POINT ( 'NONE',  ( -4.084459969179292216, 16.70604699712905372, -45.29295307432605711 ) ) ;
#21823=CARTESIAN_POINT ( 'NONE',  ( -0.9307174358028533767, 23.37631862003491889, -59.54999999999994742 ) ) ;
#21844=CARTESIAN_POINT ( 'NONE',  ( 5.565992480072003978, 18.52860470043125574, -43.79295307432606421 ) ) ;
#21850=CARTESIAN_POINT ( 'NONE',  ( 4.342430937695320736, 16.96683151040971538, -67.94295307432605568 ) ) ;
#21865=CARTESIAN_POINT ( 'NONE',  ( 4.318543150850367773, 16.81600996003516357, -48.44999999999994600 ) ) ;
#21887=CARTESIAN_POINT ( 'NONE',  ( -4.318543150850366885, 18.18399003996480801, -25.94999999999996732 ) ) ;
#21892=CARTESIAN_POINT ( 'NONE',  ( 4.107178604518054499, 18.15051318458946383, -33.29999999999996874 ) ) ;
#21900=CARTESIAN_POINT ( 'NONE',  ( -0.6839900399647736995, 21.81854315085035623, -53.54999999999996163 ) ) ;
#21903=CARTESIAN_POINT ( 'NONE',  ( -4.975717084895059372, 20.19824746994243370, -48.60704692567386331 ) ) ;
#21904=CARTESIAN_POINT ( 'NONE',  ( 2.568848540478311460, 12.45835086740561692, -33.89999999999996305 ) ) ;
#21905=CARTESIAN_POINT ( 'NONE',  ( -1.985016409143819605, 13.60418594181426855, -73.34999999999996589 ) ) ;
#21916=CARTESIAN_POINT ( 'NONE',  ( 2.701047200102605572, 22.80110361078655856, -74.84999999999993747 ) ) ;
#21923=CARTESIAN_POINT ( 'NONE',  ( -4.314955953707389824, 21.59900333660018390, -39.74295307432605995 ) ) ;
#21941=CARTESIAN_POINT ( 'NONE',  ( -4.314955953707389824, 21.59900333660018390, -60.74295307432605995 ) ) ;
#21947=CARTESIAN_POINT ( 'NONE',  ( -0.6505131845895224529, 13.39282139548194195, -31.19999999999996376 ) ) ;
#21948=CARTESIAN_POINT ( 'NONE',  ( -3.895814058185739448, 15.51498359085620571, -64.64999999999994884 ) ) ;
#21959=CARTESIAN_POINT ( 'NONE',  ( -3.639207298612509689, 19.51726172033310647, -27.60704692567387397 ) ) ;
#21960=CARTESIAN_POINT ( 'NONE',  ( 4.206979645153768210, 13.29302035484617406, -60.74999999999996447 ) ) ;
#21974=CARTESIAN_POINT ( 'NONE',  ( 1.028604700431328567, 23.06599248007198355, -52.20704692567388605 ) ) ;
#21979=ADVANCED_FACE ( 'NONE', ( #22147 ), #13569, .F. ) ;
#21981=CARTESIAN_POINT ( 'NONE',  ( -5.107581180293630396, 19.93944961101426827, -72.59295307432606137 ) ) ;
#21997=CARTESIAN_POINT ( 'NONE',  ( -5.876318620034919782, 18.43071743580290089, -49.94999999999994600 ) ) ;
#22001=CARTESIAN_POINT ( 'NONE',  ( 0.7939530028709752552, 21.58445996917927445, -61.20704692567387184 ) ) ;
#22002=CARTESIAN_POINT ( 'NONE',  ( -1.985016409143819605, 13.60418594181426855, -55.34999999999996589 ) ) ;
#22012=CARTESIAN_POINT ( 'NONE',  ( 4.107178604518054499, 18.15051318458946383, -72.29999999999996874 ) ) ;
#22014=CARTESIAN_POINT ( 'NONE',  ( -3.965139115708213868, 15.65104167704456906, -51.15704692567387468 ) ) ;
#22017=CARTESIAN_POINT ( 'NONE',  ( -3.705139346311794313, 19.38786279086902198, -71.09999999999996589 ) ) ;
#22020=CARTESIAN_POINT ( 'NONE',  ( -2.837723661809363751, 14.45689319447982335, -44.99295307432606705 ) ) ;
#22034=CARTESIAN_POINT ( 'NONE',  ( 2.568848540478311460, 12.45835086740561692, -51.89999999999997016 ) ) ;
#22055=CARTESIAN_POINT ( 'NONE',  ( 5.900206406879871857, 16.72010411457162604, -49.94295307432606279 ) ) ;
#22067=CARTESIAN_POINT ( 'NONE',  ( -1.848958322955462474, 13.53486088429179546, -50.84295307432606137 ) ) ;
#22083=CARTESIAN_POINT ( 'NONE',  ( 3.705139346311793869, 15.61213720913094960, -36.59999999999996589 ) ) ;
#22107=CARTESIAN_POINT ( 'NONE',  ( 1.887862790868997109, 13.79486065368817194, -30.89999999999996305 ) ) ;
#22109=CARTESIAN_POINT ( 'NONE',  ( -5.900206406879871857, 18.27989588542834554, -30.44295307432605213 ) ) ;
#22110=CARTESIAN_POINT ( 'NONE',  ( 3.705139346311793869, 15.61213720913094960, -27.59999999999996589 ) ) ;
#22118=CARTESIAN_POINT ( 'NONE',  ( 0.6839900399647733664, 13.18145684914961357, -55.04999999999995453 ) ) ;
#22121=CARTESIAN_POINT ( 'NONE',  ( -2.837105286290963146, 12.26822144673588255, -32.85704692567387752 ) ) ;
#22122=CARTESIAN_POINT ( 'NONE',  ( 0.9307174358028527106, 11.62368137996505801, -31.04999999999996163 ) ) ;
#22123=CARTESIAN_POINT ( 'NONE',  ( 3.705139346311793869, 15.61213720913094960, -72.59999999999996589 ) ) ;
#22134=CARTESIAN_POINT ( 'NONE',  ( -4.975717084895059372, 20.19824746994243370, -30.60704692567387752 ) ) ;
#22139=CARTESIAN_POINT ( 'NONE',  ( 2.564989113914249330, 22.87042866830903876, -43.34295307432605426 ) ) ;
#22147=FACE_OUTER_BOUND ( 'NONE', #38753, .T. ) ;
#22158=CARTESIAN_POINT ( 'NONE',  ( 5.565992480072003978, 18.52860470043125574, -64.79295307432606421 ) ) ;
#22163=CARTESIAN_POINT ( 'NONE',  ( 3.705139346311793869, 15.61213720913094960, -33.59999999999996589 ) ) ;
#22164=CARTESIAN_POINT ( 'NONE',  ( 0.6505131845895220088, 21.60717860451803674, -50.69999999999996732 ) ) ;
#22174=CARTESIAN_POINT ( 'NONE',  ( -4.099003336600151925, 21.81495595370741469, -72.75704692567386189 ) ) ;
#22175=CARTESIAN_POINT ( 'NONE',  ( 4.001075405444606048, 21.50107540544455276, -50.99999999999997158 ) ) ;
#22187=CARTESIAN_POINT ( 'NONE',  ( -4.099003336600151925, 21.81495595370741469, -51.75704692567388321 ) ) ;
#22190=CARTESIAN_POINT ( 'NONE',  ( 5.231778553264135212, 20.33710528629089254, -70.64295307432605853 ) ) ;
#22205=CARTESIAN_POINT ( 'NONE',  ( -5.301103610786608300, 14.79895279989743706, -46.64999999999994884 ) ) ;
#22209=CARTESIAN_POINT ( 'NONE',  ( -2.121074495332175847, 13.67351099933674341, -59.85704692567387752 ) ) ;
#22210=CARTESIAN_POINT ( 'NONE',  ( -3.895814058185739892, 15.51498359085620748, -58.64999999999996305 ) ) ;
#22219=CARTESIAN_POINT ( 'NONE',  ( -3.705139346311794313, 19.38786279086902198, -65.09999999999996589 ) ) ;
#22221=CARTESIAN_POINT ( 'NONE',  ( -2.121074495332175847, 13.67351099933674341, -53.85704692567387042 ) ) ;
#22226=CARTESIAN_POINT ( 'NONE',  ( -3.826489000663265472, 15.37892550466785480, -48.14295307432606563 ) ) ;
#22239=CARTESIAN_POINT ( 'NONE',  ( -0.9307174358028533767, 23.37631862003491889, -50.54999999999996163 ) ) ;
#22255=CARTESIAN_POINT ( 'NONE',  ( 2.568848540478311460, 12.45835086740561692, -66.89999999999997726 ) ) ;
#22260=CARTESIAN_POINT ( 'NONE',  ( 0.6505131845895220088, 21.60717860451803674, -44.69999999999996021 ) ) ;
#22261=CARTESIAN_POINT ( 'NONE',  ( 2.564989113914249330, 22.87042866830903876, -43.34295307432605426 ) ) ;
#22269=CARTESIAN_POINT ( 'NONE',  ( 4.084459969179292216, 18.29395300287091430, -55.79295307432606421 ) ) ;
#22286=CARTESIAN_POINT ( 'NONE',  ( -1.985016409143819605, 13.60418594181426855, -37.34999999999994458 ) ) ;
#22310=CARTESIAN_POINT ( 'NONE',  ( -0.7939530028709754772, 13.41554003082070246, -38.70704692567387184 ) ) ;
#22314=CARTESIAN_POINT ( 'NONE',  ( 0.7417250638684235176, 23.11142975074950101, -34.19295307432605568 ) ) ;
#22315=CARTESIAN_POINT ( 'NONE',  ( -3.639207298612509689, 19.51726172033310647, -72.60704692567387042 ) ) ;
#22323=CARTESIAN_POINT ( 'NONE',  ( -1.985016409143819605, 13.60418594181426855, -43.34999999999994458 ) ) ;
#22326=CARTESIAN_POINT ( 'NONE',  ( -4.103766977300021601, 13.60161616641083704, -36.00704692567386189 ) ) ;
#22328=CARTESIAN_POINT ( 'NONE',  ( 0.6839900399647733664, 13.18145684914961357, -64.04999999999994031 ) ) ;
#22338=CARTESIAN_POINT ( 'NONE',  ( 0.8851648821498760977, 23.08871111541074228, -74.69999999999997442 ) ) ;
#22342=CARTESIAN_POINT ( 'NONE',  ( -5.565992480072003978, 16.47139529956871229, -45.29295307432605711 ) ) ;
#22357=CARTESIAN_POINT ( 'NONE',  ( -1.081538986177402961, 23.35243083318996327, -61.04295307432605711 ) ) ;
#22363=CARTESIAN_POINT ( 'NONE',  ( 4.107178604518054499, 18.15051318458946383, -27.29999999999996163 ) ) ;
#22364=CARTESIAN_POINT ( 'NONE',  ( 1.887862790868997109, 13.79486065368817194, -57.89999999999996305 ) ) ;
#22376=CARTESIAN_POINT ( 'NONE',  ( -5.611429750749524992, 16.75827493613162034, -63.30704692567387326 ) ) ;
#22377=CARTESIAN_POINT ( 'NONE',  ( -5.041649132594344884, 20.06884854047834921, -59.09999999999997300 ) ) ;
#22390=CARTESIAN_POINT ( 'NONE',  ( -5.611429750749524992, 16.75827493613162034, -57.30704692567387326 ) ) ;
#22393=CARTESIAN_POINT ( 'NONE',  ( 1.081538986177402295, 11.64756916681001186, -68.54295307432605000 ) ) ;
#22410=CARTESIAN_POINT ( 'NONE',  ( 5.876318620034919782, 16.56928256419707068, -39.44999999999994600 ) ) ;
#22414=CARTESIAN_POINT ( 'NONE',  ( 0.7939530028709752552, 21.58445996917927445, -64.20704692567387895 ) ) ;
#22415=CARTESIAN_POINT ( 'NONE',  ( 2.940415233664778416, 20.44041523366473712, -47.99999999999996447 ) ) ;
#22425=CARTESIAN_POINT ( 'NONE',  ( 2.940415233664778416, 20.44041523366473712, -65.99999999999997158 ) ) ;
#22427=CARTESIAN_POINT ( 'NONE',  ( 2.121074495332174958, 21.32648900066323350, -49.35704692567387042 ) ) ;
#22445=CARTESIAN_POINT ( 'NONE',  ( 5.301103610786608300, 20.20104720010253985, -51.14999999999994884 ) ) ;
#22460=CARTESIAN_POINT ( 'NONE',  ( -5.041649132594344884, 20.06884854047834921, -74.09999999999996589 ) ) ;
#22465=CARTESIAN_POINT ( 'NONE',  ( -4.107178604518053611, 16.84948681541050775, -40.79999999999996874 ) ) ;
#22476=CARTESIAN_POINT ( 'NONE',  ( 0.5070733663080689846, 21.62989723985679902, -52.19295307432606279 ) ) ;
#22492=CARTESIAN_POINT ( 'NONE',  ( 4.318543150850367773, 16.81600996003516357, -33.44999999999994600 ) ) ;
#22516=CARTESIAN_POINT ( 'NONE',  ( 1.758463861404912620, 13.72892860598888731, -32.40704692567386758 ) ) ;
#22517=CARTESIAN_POINT ( 'NONE',  ( 0.6505131845895220088, 21.60717860451803674, -29.69999999999996376 ) ) ;
#22521=CARTESIAN_POINT ( 'NONE',  ( -5.565992480072003978, 16.47139529956871229, -36.29295307432605000 ) ) ;
#22522=CARTESIAN_POINT ( 'NONE',  ( 3.639207298612508801, 15.48273827966686866, -71.10704692567387042 ) ) ;
#22531=CARTESIAN_POINT ( 'NONE',  ( -4.107178604518053611, 16.84948681541050775, -46.79999999999996874 ) ) ;
#22534=CARTESIAN_POINT ( 'NONE',  ( 4.103766977300021601, 21.39838383358913987, -34.50704692567386900 ) ) ;
#22536=CARTESIAN_POINT ( 'NONE',  ( -0.6839900399647736995, 21.81854315085035623, -62.54999999999996874 ) ) ;
#22541=( NAMED_UNIT ( * ) SI_UNIT ( $, .STERADIAN. ) SOLID_ANGLE_UNIT ( ) );
#22552=CARTESIAN_POINT ( 'NONE',  ( 5.900206406879871857, 16.72010411457162604, -37.94295307432606279 ) ) ;
#22570=CARTESIAN_POINT ( 'NONE',  ( -1.081538986177402961, 23.35243083318996327, -67.04295307432605000 ) ) ;
#22579=CARTESIAN_POINT ( 'NONE',  ( -3.705139346311794313, 19.38786279086902198, -53.09999999999996589 ) ) ;
#22589=CARTESIAN_POINT ( 'NONE',  ( -5.370428668309080500, 14.93501088608579153, -66.15704692567388179 ) ) ;
#22590=CARTESIAN_POINT ( 'NONE',  ( 0.9307174358028527106, 11.62368137996505801, -55.04999999999996163 ) ) ;
#22602=CARTESIAN_POINT ( 'NONE',  ( -5.852430833189966819, 18.58153898617744915, -57.45704692567387895 ) ) ;
#22605=CARTESIAN_POINT ( 'NONE',  ( -5.107581180293630396, 19.93944961101426827, -66.59295307432604716 ) ) ;
#22624=CARTESIAN_POINT ( 'NONE',  ( -4.001075405444606936, 13.49892459455542060, -40.49999999999996447 ) ) ;
#22630=CARTESIAN_POINT ( 'NONE',  ( -1.758463861404912842, 21.27107139401109137, -57.90704692567388179 ) ) ;
#22631=CARTESIAN_POINT ( 'NONE',  ( -4.107178604518053611, 16.84948681541050775, -52.79999999999996874 ) ) ;
#22640=CARTESIAN_POINT ( 'NONE',  ( -4.107178604518053611, 16.84948681541050775, -64.79999999999996874 ) ) ;
#22642=CARTESIAN_POINT ( 'NONE',  ( -0.7939530028709754772, 13.41554003082070246, -41.70704692567387184 ) ) ;
#22648=CARTESIAN_POINT ( 'NONE',  ( -3.826489000663265472, 15.37892550466785480, -45.14295307432605853 ) ) ;
#22662=CARTESIAN_POINT ( 'NONE',  ( -5.588711115410763597, 16.61483511785016987, -43.79999999999996163 ) ) ;
#22678=CARTESIAN_POINT ( 'NONE',  ( 5.876318620034919782, 16.56928256419707068, -69.44999999999997442 ) ) ;
#22683=CARTESIAN_POINT ( 'NONE',  ( 0.6839900399647733664, 13.18145684914961357, -40.04999999999994742 ) ) ;
#22694=CARTESIAN_POINT ( 'NONE',  ( 3.826489000663266360, 19.62107449533211678, -55.64295307432606563 ) ) ;
#22710=CARTESIAN_POINT ( 'NONE',  ( 0.6505131845895220088, 21.60717860451803674, -32.69999999999996732 ) ) ;
#22736=CARTESIAN_POINT ( 'NONE',  ( -2.983759233219601903, 20.69971185032686023, -30.75704692567387610 ) ) ;
#22741=CARTESIAN_POINT ( 'NONE',  ( -3.965139115708213868, 15.65104167704456906, -72.15704692567386758 ) ) ;
#22749=CARTESIAN_POINT ( 'NONE',  ( -0.6839900399647736995, 21.81854315085035623, -44.54999999999994742 ) ) ;
#22752=CARTESIAN_POINT ( 'NONE',  ( 2.837105286290961370, 22.73177855326409613, -34.35704692567387752 ) ) ;
#22754=CARTESIAN_POINT ( 'NONE',  ( 3.705139346311793869, 15.61213720913094960, -66.59999999999996589 ) ) ;
#22767=CARTESIAN_POINT ( 'NONE',  ( -2.698247469942396837, 22.47571708489507358, -27.89295307432605853 ) ) ;
#22789=CARTESIAN_POINT ( 'NONE',  ( -3.091735541773221296, 20.59173554177323950, -59.24999999999997158 ) ) ;
#22800=CARTESIAN_POINT ( 'NONE',  ( -4.103766977300021601, 13.60161616641083704, -66.00704692567386189 ) ) ;
#22801=CARTESIAN_POINT ( 'NONE',  ( -5.301103610786608300, 14.79895279989743528, -58.64999999999996305 ) ) ;
#22815=CARTESIAN_POINT ( 'NONE',  ( 2.837105286290961370, 22.73177855326409613, -46.35704692567385621 ) ) ;
#22818=CARTESIAN_POINT ( 'NONE',  ( -0.7417250638684240727, 11.88857024925047057, -68.69295307432605568 ) ) ;
#22834=CARTESIAN_POINT ( 'NONE',  ( -5.876318620034919782, 18.43071743580290089, -37.94999999999996021 ) ) ;
#22837=CARTESIAN_POINT ( 'NONE',  ( 3.965139115708213868, 19.34895832295540430, -58.65704692567388179 ) ) ;
#22838=CARTESIAN_POINT ( 'NONE',  ( 4.107178604518054499, 18.15051318458946383, -45.29999999999996874 ) ) ;
#22847=CARTESIAN_POINT ( 'NONE',  ( -3.705139346311794313, 19.38786279086902198, -68.09999999999996589 ) ) ;
#22849=CARTESIAN_POINT ( 'NONE',  ( -3.043106805520194413, 14.66227633819065623, -48.00704692567387610 ) ) ;
#22853=CARTESIAN_POINT ( 'NONE',  ( -0.8348115903393239501, 21.79465536400541126, -37.04295307432605711 ) ) ;
#22869=CARTESIAN_POINT ( 'NONE',  ( 0.8851648821498760977, 23.08871111541074228, -50.69999999999996732 ) ) ;
#22885=CARTESIAN_POINT ( 'NONE',  ( -4.206979645153768210, 21.70697964515380107, -71.24999999999994316 ) ) ;
#22890=CARTESIAN_POINT ( 'NONE',  ( 1.985016409143818272, 21.39581405818570303, -41.84999999999995879 ) ) ;
#22903=CARTESIAN_POINT ( 'NONE',  ( -3.771071394011080269, 19.25846386140493394, -57.59295307432605426 ) ) ;
#22909=CARTESIAN_POINT ( 'NONE',  ( -4.342430937695320736, 18.03316848959025620, -60.44295307432605568 ) ) ;
#22920=CARTESIAN_POINT ( 'NONE',  ( 3.895814058185739448, 19.48501640914375344, -39.14999999999997016 ) ) ;
#22942=CARTESIAN_POINT ( 'NONE',  ( 3.965139115708213868, 19.34895832295540430, -34.65704692567386758 ) ) ;
#22946=CARTESIAN_POINT ( 'NONE',  ( 2.698247469942395949, 12.52428291510489977, -35.39295307432605142 ) ) ;
#22947=CARTESIAN_POINT ( 'NONE',  ( 4.129897239856814117, 18.00707336630801336, -61.80704692567387326 ) ) ;
#22954=CARTESIAN_POINT ( 'NONE',  ( 2.940415233664778416, 20.44041523366473712, -50.99999999999997158 ) ) ;
#22957=CARTESIAN_POINT ( 'NONE',  ( 4.975717084895059372, 14.80175253005754143, -35.10704692567387752 ) ) ;
#22960=CARTESIAN_POINT ( 'NONE',  ( 0.6839900399647733664, 13.18145684914961357, -67.04999999999994031 ) ) ;
#22971=CARTESIAN_POINT ( 'NONE',  ( -4.314955953707389824, 21.59900333660018390, -33.74295307432605995 ) ) ;
#22991=CARTESIAN_POINT ( 'NONE',  ( -3.895814058185739448, 15.51498359085620571, -52.64999999999997016 ) ) ;
#23000=CARTESIAN_POINT ( 'NONE',  ( -3.199711850326840246, 20.48375923321962233, -30.74295307432605640 ) ) ;
#23002=CARTESIAN_POINT ( 'NONE',  ( 5.611429750749524992, 18.24172506386835479, -64.80704692567387326 ) ) ;
#23003=CARTESIAN_POINT ( 'NONE',  ( -5.588711115410763597, 16.61483511785016987, -55.79999999999996874 ) ) ;
#23017=CARTESIAN_POINT ( 'NONE',  ( 5.852430833189966819, 16.41846101382252243, -46.95704692567387184 ) ) ;
#23021=CARTESIAN_POINT ( 'NONE',  ( -2.564989113914250662, 12.12957133169093282, -59.84295307432606137 ) ) ;
#23036=CARTESIAN_POINT ( 'NONE',  ( -5.301103610786608300, 14.79895279989743706, -40.64999999999994174 ) ) ;
#23040=CARTESIAN_POINT ( 'NONE',  ( 0.5331684895902240040, 13.15756906230466328, -50.55704692567388747 ) ) ;
#23042=CARTESIAN_POINT ( 'NONE',  ( 0.6839900399647732554, 13.18145684914961357, -49.04999999999995453 ) ) ;
#23051=CARTESIAN_POINT ( 'NONE',  ( -4.318543150850367773, 18.18399003996480801, -61.94999999999997442 ) ) ;
#23053=CARTESIAN_POINT ( 'NONE',  ( -0.5331684895902242260, 21.84243093769531185, -46.05704692567387326 ) ) ;
#23058=CARTESIAN_POINT ( 'NONE',  ( 3.771071394011080269, 15.74153613859503764, -35.09295307432605426 ) ) ;
#23065=CARTESIAN_POINT ( 'NONE',  ( -2.983759233219601903, 20.69971185032686023, -27.75704692567387255 ) ) ;
#23072=CARTESIAN_POINT ( 'NONE',  ( -2.568848540478311904, 22.54164913259435465, -35.39999999999996305 ) ) ;
#23089=CARTESIAN_POINT ( 'NONE',  ( 2.701047200102605572, 22.80110361078655856, -71.84999999999998010 ) ) ;
#23095=CARTESIAN_POINT ( 'NONE',  ( 3.705139346311793869, 15.61213720913094960, -30.59999999999996589 ) ) ;
#23107=CARTESIAN_POINT ( 'NONE',  ( 3.826489000663266360, 19.62107449533211678, -49.64295307432606563 ) ) ;
#23112=CARTESIAN_POINT ( 'NONE',  ( -1.848958322955462474, 13.53486088429179546, -62.84295307432604716 ) ) ;
#23123=CARTESIAN_POINT ( 'NONE',  ( -1.985016409143819605, 13.60418594181426855, -28.34999999999995524 ) ) ;
#23131=CARTESIAN_POINT ( 'NONE',  ( 5.852430833189966819, 16.41846101382252243, -25.95704692567387184 ) ) ;
#23150=CARTESIAN_POINT ( 'NONE',  ( -3.639207298612509689, 19.51726172033310647, -36.60704692567387752 ) ) ;
#23155=CARTESIAN_POINT ( 'NONE',  ( 2.837723661809363307, 20.54310680552015356, -73.49295307432603863 ) ) ;
#23157=CARTESIAN_POINT ( 'NONE',  ( -3.043106805520194413, 14.66227633819065623, -60.00704692567389031 ) ) ;
#23165=CARTESIAN_POINT ( 'NONE',  ( -3.091735541773221296, 20.59173554177323950, -50.24999999999997158 ) ) ;
#23168=CARTESIAN_POINT ( 'NONE',  ( 5.852430833189966819, 16.41846101382252243, -25.95704692567387184 ) ) ;
#23170=CARTESIAN_POINT ( 'NONE',  ( 3.895814058185739448, 19.48501640914375344, -60.14999999999995595 ) ) ;
#23183=CARTESIAN_POINT ( 'NONE',  ( 2.698247469942395949, 12.52428291510489977, -29.39295307432606208 ) ) ;
#23200=CARTESIAN_POINT ( 'NONE',  ( -0.6839900399647736995, 21.81854315085035623, -26.54999999999996163 ) ) ;
#23201=CARTESIAN_POINT ( 'NONE',  ( 1.887862790868997109, 13.79486065368817194, -45.89999999999997016 ) ) ;
#23209=CARTESIAN_POINT ( 'NONE',  ( 2.940415233664778416, 20.44041523366473712, -74.99999999999997158 ) ) ;
#23211=CARTESIAN_POINT ( 'NONE',  ( -4.975717084895059372, 20.19824746994243370, -63.60704692567387752 ) ) ;
#23212=CARTESIAN_POINT ( 'NONE',  ( 0.9307174358028527106, 11.62368137996505801, -43.04999999999996163 ) ) ;
#23225=CARTESIAN_POINT ( 'NONE',  ( 4.975717084895059372, 14.80175253005754143, -41.10704692567387752 ) ) ;
#23230=CARTESIAN_POINT ( 'NONE',  ( 5.231778553264135212, 20.33710528629089254, -64.64295307432604432 ) ) ;
#23248=CARTESIAN_POINT ( 'NONE',  ( 2.568848540478311460, 12.45835086740561692, -27.89999999999996660 ) ) ;
#23251=CARTESIAN_POINT ( 'NONE',  ( -4.294655364005415699, 18.33481159033935626, -57.45704692567387895 ) ) ;
#23252=CARTESIAN_POINT ( 'NONE',  ( -3.895814058185739892, 15.51498359085620748, -43.64999999999996305 ) ) ;
#23253=CARTESIAN_POINT ( 'NONE',  ( 1.985016409143818272, 21.39581405818570303, -74.84999999999993747 ) ) ;
#23261=CARTESIAN_POINT ( 'NONE',  ( 3.895814058185739448, 19.48501640914375344, -51.14999999999994884 ) ) ;
#23263=CARTESIAN_POINT ( 'NONE',  ( -0.5331684895902242260, 21.84243093769531185, -43.05704692567387326 ) ) ;
#23264=CARTESIAN_POINT ( 'NONE',  ( -4.206979645153769098, 21.70697964515380107, -71.24999999999995737 ) ) ;
#23268=CARTESIAN_POINT ( 'NONE',  ( 0.8348115903393232839, 13.20534463599456387, -38.54295307432605000 ) ) ;
#23277=CARTESIAN_POINT ( 'NONE',  ( 2.121074495332174958, 21.32648900066323350, -25.35704692567387042 ) ) ;
#23285=CARTESIAN_POINT ( 'NONE',  ( 0.9307174358028528216, 11.62368137996505801, -34.04999999999995453 ) ) ;
#23307=CARTESIAN_POINT ( 'NONE',  ( 5.301103610786608300, 20.20104720010253985, -57.14999999999995595 ) ) ;
#23314=CARTESIAN_POINT ( 'NONE',  ( 3.895814058185739448, 19.48501640914375344, -33.14999999999996305 ) ) ;
#23327=CARTESIAN_POINT ( 'NONE',  ( -3.199711850326840246, 20.48375923321962233, -45.74295307432605995 ) ) ;
#23332=CARTESIAN_POINT ( 'NONE',  ( -3.826489000663265472, 15.37892550466785480, -63.14295307432606563 ) ) ;
#23342=CARTESIAN_POINT ( 'NONE',  ( 0.6839900399647733664, 13.18145684914961357, -28.04999999999995453 ) ) ;
#23352=CARTESIAN_POINT ( 'NONE',  ( -2.568848540478311904, 22.54164913259435465, -68.39999999999997726 ) ) ;
#23368=CARTESIAN_POINT ( 'NONE',  ( -5.565992480072003978, 16.47139529956871229, -60.29295307432605000 ) ) ;
#23373=CARTESIAN_POINT ( 'NONE',  ( 3.639207298612508801, 15.48273827966686866, -29.10704692567387752 ) ) ;
#23378=CARTESIAN_POINT ( 'NONE',  ( 3.771071394011080269, 15.74153613859503764, -74.09295307432606137 ) ) ;
#23379=CARTESIAN_POINT ( 'NONE',  ( 0.7939530028709752552, 21.58445996917927445, -61.20704692567387184 ) ) ;
#23389=CARTESIAN_POINT ( 'NONE',  ( -3.091735541773221296, 20.59173554177323950, -41.24999999999995026 ) ) ;
#23392=CARTESIAN_POINT ( 'NONE',  ( -4.103766977300021601, 13.60161616641083704, -27.00704692567387610 ) ) ;
#23394=CARTESIAN_POINT ( 'NONE',  ( -0.6505131845895224529, 13.39282139548194195, -58.19999999999996732 ) ) ;
#23406=CARTESIAN_POINT ( 'NONE',  ( -2.698247469942396837, 22.47571708489507358, -30.89295307432606208 ) ) ;
#23424=CARTESIAN_POINT ( 'NONE',  ( -2.940415233664778860, 14.55958476633523802, -46.49999999999997158 ) ) ;
#23435=CARTESIAN_POINT ( 'NONE',  ( 1.887862790868997109, 13.79486065368817194, -66.89999999999997726 ) ) ;
#23437=CARTESIAN_POINT ( 'NONE',  ( 5.852430833189966819, 16.41846101382252243, -58.95704692567386473 ) ) ;
#23438=CARTESIAN_POINT ( 'NONE',  ( -2.568848540478311904, 22.54164913259435465, -44.39999999999997016 ) ) ;
#23451=CARTESIAN_POINT ( 'NONE',  ( -1.081538986177402961, 23.35243083318996327, -40.04295307432605000 ) ) ;
#23453=CARTESIAN_POINT ( 'NONE',  ( -5.852430833189966819, 18.58153898617744915, -42.45704692567387184 ) ) ;
#23457=CARTESIAN_POINT ( 'NONE',  ( -2.698247469942396837, 22.47571708489507358, -57.89295307432605853 ) ) ;
#23474=CARTESIAN_POINT ( 'NONE',  ( -4.206979645153768210, 21.70697964515380107, -35.24999999999997158 ) ) ;
#23477=CARTESIAN_POINT ( 'NONE',  ( 0.5331684895902240040, 13.15756906230466328, -53.55704692567387326 ) ) ;
#23478=CARTESIAN_POINT ( 'NONE',  ( -1.985016409143819605, 13.60418594181426855, -37.34999999999995879 ) ) ;
#23487=CARTESIAN_POINT ( 'NONE',  ( -3.705139346311794313, 19.38786279086902198, -50.09999999999996589 ) ) ;
#23490=CARTESIAN_POINT ( 'NONE',  ( 0.7939530028709752552, 21.58445996917927445, -31.20704692567387539 ) ) ;
#23491=CARTESIAN_POINT ( 'NONE',  ( -5.876318620034919782, 18.43071743580290089, -73.94999999999997442 ) ) ;
#23493=CARTESIAN_POINT ( 'NONE',  ( 2.837723661809363307, 20.54310680552015356, -37.49295307432604574 ) ) ;
#23500=CARTESIAN_POINT ( 'NONE',  ( -2.837105286290963146, 12.26822144673588255, -71.85704692567388463 ) ) ;
#23508=CARTESIAN_POINT ( 'NONE',  ( -4.206979645153768210, 21.70697964515380107, -35.24999999999997158 ) ) ;
#23527=CARTESIAN_POINT ( 'NONE',  ( -2.568848540478311904, 22.54164913259435465, -65.39999999999997726 ) ) ;
#23532=CARTESIAN_POINT ( 'NONE',  ( 4.318543150850367773, 16.81600996003516357, -30.44999999999995310 ) ) ;
#23533=CARTESIAN_POINT ( 'NONE',  ( 2.940415233664778416, 20.44041523366473712, -62.99999999999997158 ) ) ;
#23545=CARTESIAN_POINT ( 'NONE',  ( -3.826489000663265472, 15.37892550466785480, -42.14295307432605142 ) ) ;
#23550=CARTESIAN_POINT ( 'NONE',  ( 1.848958322955461808, 21.46513911570817612, -64.34295307432606137 ) ) ;
#23560=CARTESIAN_POINT ( 'NONE',  ( -0.6505131845895224529, 13.39282139548194195, -31.19999999999996376 ) ) ;
#23571=CARTESIAN_POINT ( 'NONE',  ( 0.8851648821498760977, 23.08871111541074228, -68.69999999999997442 ) ) ;
#23586=CARTESIAN_POINT ( 'NONE',  ( -5.900206406879871857, 18.27989588542834554, -51.44295307432605568 ) ) ;
#23595=CARTESIAN_POINT ( 'NONE',  ( -2.017261720333081598, 21.13920729861251857, -75.89295307432605853 ) ) ;
#23596=CARTESIAN_POINT ( 'NONE',  ( 0.5331684895902240040, 13.15756906230466328, -62.55704692567387326 ) ) ;
#23607=CARTESIAN_POINT ( 'NONE',  ( -5.370428668309080500, 14.93501088608579153, -27.15704692567387823 ) ) ;
#23609=CARTESIAN_POINT ( 'NONE',  ( 3.705139346311793869, 15.61213720913094960, -54.59999999999996589 ) ) ;
#23621=CARTESIAN_POINT ( 'NONE',  ( 4.314955953707388936, 13.40099666339979123, -35.24295307432605995 ) ) ;
#23641=CARTESIAN_POINT ( 'NONE',  ( -3.091735541773221296, 20.59173554177323950, -41.24999999999995026 ) ) ;
#23651=CARTESIAN_POINT ( 'NONE',  ( -3.895814058185739448, 15.51498359085620571, -67.64999999999997726 ) ) ;
#23654=CARTESIAN_POINT ( 'NONE',  ( 2.837105286290961370, 22.73177855326409613, -55.35704692567387752 ) ) ;
#23655=CARTESIAN_POINT ( 'NONE',  ( 4.001075405444606048, 21.50107540544455276, -44.99999999999997158 ) ) ;
#23668=CARTESIAN_POINT ( 'NONE',  ( 4.103766977300021601, 21.39838383358913987, -46.50704692567387610 ) ) ;
#23672=CARTESIAN_POINT ( 'NONE',  ( -3.898383833589191827, 13.39623302270000771, -62.99295307432606705 ) ) ;
#23687=CARTESIAN_POINT ( 'NONE',  ( -4.001075405444606936, 13.49892459455542060, -31.49999999999996447 ) ) ;
#23690=CARTESIAN_POINT ( 'NONE',  ( -3.965139115708213868, 15.65104167704456906, -51.15704692567387468 ) ) ;
#23699=CARTESIAN_POINT ( 'NONE',  ( -3.705139346311794313, 19.38786279086902198, -59.09999999999997300 ) ) ;
#23702=CARTESIAN_POINT ( 'NONE',  ( -3.639207298612509689, 19.51726172033310647, -33.60704692567387042 ) ) ;
#23703=CARTESIAN_POINT ( 'NONE',  ( -2.701047200102606460, 12.19889638921340591, -70.34999999999995168 ) ) ;
#23706=CARTESIAN_POINT ( 'NONE',  ( -0.8348115903393239501, 21.79465536400541126, -34.04295307432605711 ) ) ;
#23712=CARTESIAN_POINT ( 'NONE',  ( 4.975717084895059372, 14.80175253005754143, -71.10704692567387042 ) ) ;
#23717=CARTESIAN_POINT ( 'NONE',  ( -0.9307174358028533767, 23.37631862003491889, -38.54999999999996874 ) ) ;
#23733=CARTESIAN_POINT ( 'NONE',  ( 0.9307174358028528216, 11.62368137996505801, -58.04999999999996874 ) ) ;
#23738=CARTESIAN_POINT ( 'NONE',  ( -3.091735541773221296, 20.59173554177323950, -38.24999999999996447 ) ) ;
#23739=CARTESIAN_POINT ( 'NONE',  ( 1.985016409143818272, 21.39581405818570659, -71.84999999999996589 ) ) ;
#23749=CARTESIAN_POINT ( 'NONE',  ( -4.084459969179292216, 16.70604699712905372, -45.29295307432605711 ) ) ;
#23755=CARTESIAN_POINT ( 'NONE',  ( 1.848958322955461808, 21.46513911570817612, -67.34295307432606137 ) ) ;
#23774=CARTESIAN_POINT ( 'NONE',  ( -5.588711115410763597, 16.61483511785016987, -67.79999999999996874 ) ) ;
#23794=CARTESIAN_POINT ( 'NONE',  ( -4.314955953707389824, 21.59900333660018390, -54.74295307432605995 ) ) ;
#23804=CARTESIAN_POINT ( 'NONE',  ( 3.898383833589191383, 21.60376697729997275, -28.49295307432605995 ) ) ;
#23806=CARTESIAN_POINT ( 'NONE',  ( 1.758463861404912620, 13.72892860598888731, -65.40704692567388179 ) ) ;
#23819=CARTESIAN_POINT ( 'NONE',  ( 5.611429750749524992, 18.24172506386835479, -31.80704692567387326 ) ) ;
#23821=CARTESIAN_POINT ( 'NONE',  ( 4.318543150850367773, 16.81600996003516357, -51.44999999999997442 ) ) ;
#23832=ORIENTED_EDGE ( 'NONE', *, *, #19442, .T. ) ;
#23835=CARTESIAN_POINT ( 'NONE',  ( -2.837723661809363751, 14.45689319447982335, -68.99295307432605284 ) ) ;
#23846=AXIS2_PLACEMENT_3D ( 'NONE', #37922, #21341, #34936 ) ;
#23856=CARTESIAN_POINT ( 'NONE',  ( 2.940415233664778416, 20.44041523366473712, -44.99999999999997158 ) ) ;
#23866=CARTESIAN_POINT ( 'NONE',  ( 2.940415233664778416, 20.44041523366473712, -68.99999999999995737 ) ) ;
#23868=CARTESIAN_POINT ( 'NONE',  ( 4.103766977300021601, 21.39838383358913987, -52.50704692567387610 ) ) ;
#23869=CARTESIAN_POINT ( 'NONE',  ( -0.8851648821498765418, 11.91128888458923285, -43.19999999999996732 ) ) ;
#23880=CARTESIAN_POINT ( 'NONE',  ( 4.975717084895059372, 14.80175253005754143, -38.10704692567387752 ) ) ;
#23885=CARTESIAN_POINT ( 'NONE',  ( -2.698247469942396837, 22.47571708489507358, -60.89295307432605853 ) ) ;
#23901=CARTESIAN_POINT ( 'NONE',  ( 5.588711115410763597, 18.38516488214980882, -33.29999999999996874 ) ) ;
#23904=CARTESIAN_POINT ( 'NONE',  ( 4.294655364005415699, 16.66518840966061887, -49.95704692567387184 ) ) ;
#23905=CARTESIAN_POINT ( 'NONE',  ( 2.940415233664778416, 20.44041523366473712, -74.99999999999997158 ) ) ;
#23912=CARTESIAN_POINT ( 'NONE',  ( -0.6839900399647736995, 21.81854315085035623, -56.54999999999996874 ) ) ;
#23914=CARTESIAN_POINT ( 'NONE',  ( 4.129897239856814117, 18.00707336630801336, -34.80704692567387326 ) ) ;
#23925=CARTESIAN_POINT ( 'NONE',  ( -3.043106805520194413, 14.66227633819065623, -27.00704692567387610 ) ) ;
#23931=CARTESIAN_POINT ( 'NONE',  ( -0.8851648821498765418, 11.91128888458923285, -40.19999999999996732 ) ) ;
#23950=CARTESIAN_POINT ( 'NONE',  ( 2.568848540478311460, 12.45835086740561692, -60.89999999999997016 ) ) ;
#23955=CARTESIAN_POINT ( 'NONE',  ( -1.887862790868997553, 21.20513934631180319, -29.39999999999996660 ) ) ;
#23956=CARTESIAN_POINT ( 'NONE',  ( -0.6505131845895224529, 13.39282139548194195, -67.19999999999997442 ) ) ;
#23968=CARTESIAN_POINT ( 'NONE',  ( -3.826489000663265472, 15.37892550466785480, -48.14295307432606563 ) ) ;
#23974=CARTESIAN_POINT ( 'NONE',  ( -4.084459969179292216, 16.70604699712905372, -54.29295307432607132 ) ) ;
#23983=CARTESIAN_POINT ( 'NONE',  ( 1.985016409143818272, 21.39581405818570303, -26.84999999999995524 ) ) ;
#23991=CARTESIAN_POINT ( 'NONE',  ( -5.876318620034919782, 18.43071743580290089, -70.94999999999997442 ) ) ;
#24012=CARTESIAN_POINT ( 'NONE',  ( -2.564989113914250662, 12.12957133169093282, -50.84295307432606137 ) ) ;
#24018=CARTESIAN_POINT ( 'NONE',  ( 3.826489000663266360, 19.62107449533211678, -73.64295307432605853 ) ) ;
#24019=CARTESIAN_POINT ( 'NONE',  ( -1.758463861404912842, 21.27107139401109137, -57.90704692567388179 ) ) ;
#24034=CARTESIAN_POINT ( 'NONE',  ( 2.940415233664778416, 20.44041523366473712, -53.99999999999996447 ) ) ;
#24047=CARTESIAN_POINT ( 'NONE',  ( 2.017261720333081598, 13.86079270138745834, -74.39295307432605853 ) ) ;
#24068=CARTESIAN_POINT ( 'NONE',  ( -4.107178604518053611, 16.84948681541050775, -49.79999999999996874 ) ) ;
#24077=CARTESIAN_POINT ( 'NONE',  ( -1.887862790868997553, 21.20513934631180319, -65.39999999999997726 ) ) ;
#24079=CARTESIAN_POINT ( 'NONE',  ( -0.7798958854283041253, 23.40020640687986386, -55.05704692567387326 ) ) ;
#24080=CARTESIAN_POINT ( 'NONE',  ( 5.876318620034919782, 16.56928256419707068, -48.44999999999996732 ) ) ;
#24093=CARTESIAN_POINT ( 'NONE',  ( 5.611429750749524992, 18.24172506386835479, -37.80704692567387326 ) ) ;
#24098=CARTESIAN_POINT ( 'NONE',  ( 3.898383833589191383, 21.60376697729997275, -52.49295307432605995 ) ) ;
#24112=DIRECTION ( 'NONE',  ( 0.000000000000000000, 0.000000000000000000, 1.000000000000000000 ) ) ;
#24113=CARTESIAN_POINT ( 'NONE',  ( 0.9307174358028528216, 11.62368137996505801, -37.04999999999996163 ) ) ;
#24116=CARTESIAN_POINT ( 'NONE',  ( 3.639207298612508801, 15.48273827966686866, -47.10704692567387042 ) ) ;
#24126=CARTESIAN_POINT ( 'NONE',  ( 3.705139346311793869, 15.61213720913094960, -54.59999999999996589 ) ) ;
#24130=CARTESIAN_POINT ( 'NONE',  ( 4.294655364005415699, 16.66518840966061887, -34.95704692567387895 ) ) ;
#24141=CARTESIAN_POINT ( 'NONE',  ( -2.439449611014227859, 22.60758118029364283, -63.90704692567388179 ) ) ;
#24147=CARTESIAN_POINT ( 'NONE',  ( 5.301103610786608300, 20.20104720010253985, -27.14999999999995595 ) ) ;
#24153=CARTESIAN_POINT ( 'NONE',  ( -4.107178604518053611, 16.84948681541050775, -64.79999999999996874 ) ) ;
#24162=CARTESIAN_POINT ( 'NONE',  ( 4.001075405444606048, 21.50107540544455276, -59.99999999999997158 ) ) ;
#24166=CARTESIAN_POINT ( 'NONE',  ( -0.6505131845895224529, 13.39282139548194195, -28.19999999999996732 ) ) ;
#24167=CARTESIAN_POINT ( 'NONE',  ( -4.107178604518053611, 16.84948681541050775, -67.79999999999996874 ) ) ;
#24178=CARTESIAN_POINT ( 'NONE',  ( 3.826489000663266360, 19.62107449533211678, -37.64295307432604432 ) ) ;
#24183=CARTESIAN_POINT ( 'NONE',  ( 4.084459969179292216, 18.29395300287091430, -58.79295307432606421 ) ) ;
#24200=CARTESIAN_POINT ( 'NONE',  ( -4.001075405444606936, 13.49892459455542060, -64.49999999999997158 ) ) ;
#24223=CARTESIAN_POINT ( 'NONE',  ( -0.8348115903393239501, 21.79465536400541126, -61.04295307432605711 ) ) ;
#24225=CARTESIAN_POINT ( 'NONE',  ( -0.7939530028709754772, 13.41554003082070246, -56.70704692567387184 ) ) ;
#24238=CARTESIAN_POINT ( 'NONE',  ( -3.895814058185739448, 15.51498359085620571, -43.64999999999996305 ) ) ;
#24247=CARTESIAN_POINT ( 'NONE',  ( -0.8348115903393239501, 21.79465536400541126, -76.04295307432605000 ) ) ;
#24260=CARTESIAN_POINT ( 'NONE',  ( 1.887862790868997109, 13.79486065368817194, -39.89999999999996305 ) ) ;
#24266=CARTESIAN_POINT ( 'NONE',  ( 3.895814058185739448, 19.48501640914375344, -39.14999999999997016 ) ) ;
#24275=CARTESIAN_POINT ( 'NONE',  ( -3.091735541773221296, 20.59173554177323950, -68.24999999999995737 ) ) ;
#24276=CARTESIAN_POINT ( 'NONE',  ( 4.975717084895059372, 14.80175253005754143, -44.10704692567387752 ) ) ;
#24277=CARTESIAN_POINT ( 'NONE',  ( -4.001075405444606936, 13.49892459455542060, -40.49999999999996447 ) ) ;
#24290=CARTESIAN_POINT ( 'NONE',  ( -5.370428668309080500, 14.93501088608579153, -36.15704692567386758 ) ) ;
#24297=CARTESIAN_POINT ( 'NONE',  ( 3.898383833589191383, 21.60376697729997275, -55.49295307432605995 ) ) ;
#24314=CARTESIAN_POINT ( 'NONE',  ( -5.588711115410763597, 16.61483511785016987, -25.79999999999996163 ) ) ;
#24317=CARTESIAN_POINT ( 'NONE',  ( 3.043106805520193525, 20.33772366180932067, -43.50704692567387610 ) ) ;
#24319=CARTESIAN_POINT ( 'NONE',  ( 4.107178604518054499, 18.15051318458946383, -66.29999999999996874 ) ) ;
#24329=CARTESIAN_POINT ( 'NONE',  ( -3.043106805520194413, 14.66227633819065623, -39.00704692567386900 ) ) ;
#24330=CARTESIAN_POINT ( 'NONE',  ( -5.041649132594344884, 20.06884854047834921, -68.09999999999996589 ) ) ;
#24341=CARTESIAN_POINT ( 'NONE',  ( 4.099003336600150149, 13.18504404629255689, -65.25704692567387610 ) ) ;
#24346=CARTESIAN_POINT ( 'NONE',  ( -5.301103610786608300, 14.79895279989743706, -28.64999999999995950 ) ) ;
#24361=CARTESIAN_POINT ( 'NONE',  ( -4.001075405444606936, 13.49892459455542060, -49.49999999999996447 ) ) ;
#24365=CARTESIAN_POINT ( 'NONE',  ( -0.5331684895902242260, 21.84243093769531185, -70.05704692567387326 ) ) ;
#24366=CARTESIAN_POINT ( 'NONE',  ( -0.6839900399647738105, 21.81854315085035623, -68.54999999999996874 ) ) ;
#24374=CARTESIAN_POINT ( 'NONE',  ( 3.895814058185739448, 19.48501640914375344, -69.14999999999994884 ) ) ;
#24378=CARTESIAN_POINT ( 'NONE',  ( -4.084459969179292216, 16.70604699712905372, -36.29295307432605000 ) ) ;
#24381=CARTESIAN_POINT ( 'NONE',  ( 2.837723661809363307, 20.54310680552015356, -58.49295307432606705 ) ) ;
#24397=CARTESIAN_POINT ( 'NONE',  ( 4.206979645153767322, 13.29302035484617051, -57.74999999999995737 ) ) ;
#24407=MANIFOLD_SOLID_BREP ( 'Sweep1', #8388 ) ;
#24419=CARTESIAN_POINT ( 'NONE',  ( -5.900206406879871857, 18.27989588542834554, -57.44295307432606990 ) ) ;
#24428=CARTESIAN_POINT ( 'NONE',  ( -3.199711850326840246, 20.48375923321962233, -69.74295307432603863 ) ) ;
#24430=CARTESIAN_POINT ( 'NONE',  ( 0.7939530028709752552, 21.58445996917927445, -55.20704692567388605 ) ) ;
#24443=CARTESIAN_POINT ( 'NONE',  ( 3.091735541773220852, 14.40826445822673563, -42.74999999999996447 ) ) ;
#24454=CARTESIAN_POINT ( 'NONE',  ( -0.5070733663080690956, 13.37010276014318144, -74.69295307432606990 ) ) ;
#24467=CARTESIAN_POINT ( 'NONE',  ( 2.940415233664778416, 20.44041523366473712, -35.99999999999996447 ) ) ;
#24472=CARTESIAN_POINT ( 'NONE',  ( -1.887862790868997553, 21.20513934631180319, -35.39999999999996305 ) ) ;
#24482=CARTESIAN_POINT ( 'NONE',  ( 4.107178604518054499, 18.15051318458946383, -57.29999999999996874 ) ) ;
#24484=CARTESIAN_POINT ( 'NONE',  ( 4.103766977300021601, 21.39838383358913987, -49.50704692567387610 ) ) ;
#24485=CARTESIAN_POINT ( 'NONE',  ( 5.041649132594343996, 14.93115145952162415, -33.59999999999996589 ) ) ;
#24488=CARTESIAN_POINT ( 'NONE',  ( -2.940415233664778860, 14.55958476633523802, -70.49999999999997158 ) ) ;
#24499=CARTESIAN_POINT ( 'NONE',  ( -5.611429750749524992, 16.75827493613162034, -33.30704692567387326 ) ) ;
#24504=CARTESIAN_POINT ( 'NONE',  ( -5.900206406879871857, 18.27989588542834554, -54.44295307432606990 ) ) ;
#24520=CARTESIAN_POINT ( 'NONE',  ( -4.314955953707389824, 21.59900333660018390, -75.74295307432603863 ) ) ;
#24523=CARTESIAN_POINT ( 'NONE',  ( 4.129897239856814117, 18.00707336630801336, -43.80704692567387326 ) ) ;
#24524=CARTESIAN_POINT ( 'NONE',  ( 4.318543150850367773, 16.81600996003516357, -33.44999999999994600 ) ) ;
#24526=CARTESIAN_POINT ( 'NONE',  ( 0.6505131845895220088, 21.60717860451803674, -68.69999999999997442 ) ) ;
#24535=CARTESIAN_POINT ( 'NONE',  ( 5.852430833189966819, 16.41846101382252243, -70.95704692567389316 ) ) ;
#24536=CARTESIAN_POINT ( 'NONE',  ( -0.8851648821498765418, 11.91128888458923285, -64.19999999999996021 ) ) ;
#24547=CARTESIAN_POINT ( 'NONE',  ( -5.370428668309080500, 14.93501088608579153, -60.15704692567387468 ) ) ;
#24552=CARTESIAN_POINT ( 'NONE',  ( 2.701047200102605572, 22.80110361078655856, -26.84999999999995524 ) ) ;
#24569=CARTESIAN_POINT ( 'NONE',  ( -2.701047200102606016, 12.19889638921340413, -49.34999999999996589 ) ) ;
#24573=CARTESIAN_POINT ( 'NONE',  ( 3.043106805520193525, 20.33772366180932067, -70.50704692567386189 ) ) ;
#24574=CARTESIAN_POINT ( 'NONE',  ( 0.6505131845895220088, 21.60717860451803674, -53.69999999999996732 ) ) ;
#24588=CARTESIAN_POINT ( 'NONE',  ( -0.5070733663080690956, 13.37010276014318144, -35.69295307432606279 ) ) ;
#24591=CARTESIAN_POINT ( 'NONE',  ( -0.8348115903393239501, 21.79465536400541126, -58.04295307432605711 ) ) ;
#24605=CARTESIAN_POINT ( 'NONE',  ( 5.041649132594343996, 14.93115145952162415, -60.59999999999996589 ) ) ;
#24630=CARTESIAN_POINT ( 'NONE',  ( 5.231778553264135212, 20.33710528629089254, -49.64295307432606563 ) ) ;
#24639=CARTESIAN_POINT ( 'NONE',  ( -0.8348115903393239501, 21.79465536400541126, -67.04295307432605000 ) ) ;
#24654=CARTESIAN_POINT ( 'NONE',  ( 0.6839900399647733664, 13.18145684914961357, -43.04999999999996163 ) ) ;
#24680=CARTESIAN_POINT ( 'NONE',  ( -3.895814058185739892, 15.51498359085620748, -37.64999999999997016 ) ) ;
#24685=CARTESIAN_POINT ( 'NONE',  ( 3.895814058185739448, 19.48501640914375344, -33.14999999999996305 ) ) ;
#24693=CARTESIAN_POINT ( 'NONE',  ( 3.895814058185739448, 19.48501640914375344, -51.14999999999994884 ) ) ;
#24695=CARTESIAN_POINT ( 'NONE',  ( 5.370428668309080500, 20.06498911391418360, -46.65704692567388179 ) ) ;
#24696=CARTESIAN_POINT ( 'NONE',  ( 5.876318620034919782, 16.56928256419707068, -39.44999999999996021 ) ) ;
#24699=CARTESIAN_POINT ( 'NONE',  ( 3.199711850326839357, 14.51624076678035635, -29.24295307432605640 ) ) ;
#24710=CARTESIAN_POINT ( 'NONE',  ( -4.975717084895059372, 20.19824746994243370, -36.60704692567387752 ) ) ;
#24716=CARTESIAN_POINT ( 'NONE',  ( -2.564989113914250662, 12.12957133169093282, -50.84295307432606137 ) ) ;
#24732=CARTESIAN_POINT ( 'NONE',  ( -5.900206406879871857, 18.27989588542834554, -72.44295307432605568 ) ) ;
#24736=CARTESIAN_POINT ( 'NONE',  ( 3.043106805520193525, 20.33772366180932067, -40.50704692567387610 ) ) ;
#24737=CARTESIAN_POINT ( 'NONE',  ( -1.985016409143819605, 13.60418594181426855, -34.34999999999995879 ) ) ;
#24738=CARTESIAN_POINT ( 'NONE',  ( 4.107178604518054499, 18.15051318458946383, -60.29999999999996163 ) ) ;
#24748=CARTESIAN_POINT ( 'NONE',  ( 0.7939530028709752552, 21.58445996917927445, -28.20704692567387184 ) ) ;
#24749=CARTESIAN_POINT ( 'NONE',  ( 4.206979645153768210, 13.29302035484617406, -69.74999999999997158 ) ) ;
#24763=CARTESIAN_POINT ( 'NONE',  ( -5.611429750749524992, 16.75827493613162034, -60.30704692567387326 ) ) ;
#24767=CARTESIAN_POINT ( 'NONE',  ( -2.698247469942396837, 22.47571708489507358, -75.89295307432605853 ) ) ;
#24785=CARTESIAN_POINT ( 'NONE',  ( -0.8851648821498765418, 11.91128888458923285, -49.19999999999996732 ) ) ;
#24789=CARTESIAN_POINT ( 'NONE',  ( 0.7939530028709752552, 21.58445996917927445, -73.20704692567387895 ) ) ;
#24790=CARTESIAN_POINT ( 'NONE',  ( -4.107178604518053611, 16.84948681541050775, -61.79999999999996874 ) ) ;
#24796=CARTESIAN_POINT ( 'NONE',  ( 0.6505131845895220088, 21.60717860451803674, -74.69999999999997442 ) ) ;
#24801=CARTESIAN_POINT ( 'NONE',  ( -3.826489000663265472, 15.37892550466785480, -39.14295307432606563 ) ) ;
#24804=CARTESIAN_POINT ( 'NONE',  ( -4.342430937695320736, 18.03316848959025620, -57.44295307432606990 ) ) ;
#24821=CARTESIAN_POINT ( 'NONE',  ( 5.876318620034919782, 16.56928256419707068, -60.44999999999997442 ) ) ;
#24843=CARTESIAN_POINT ( 'NONE',  ( -1.081538986177402961, 23.35243083318996327, -46.04295307432605711 ) ) ;
#24852=CARTESIAN_POINT ( 'NONE',  ( 0.8348115903393232839, 13.20534463599456387, -68.54295307432605000 ) ) ;
#24863=CARTESIAN_POINT ( 'NONE',  ( -3.091735541773221296, 20.59173554177323950, -44.24999999999997868 ) ) ;
#24886=CARTESIAN_POINT ( 'NONE',  ( 4.318543150850366885, 16.81600996003516713, -27.44999999999996376 ) ) ;
#24891=CARTESIAN_POINT ( 'NONE',  ( -0.6505131845895224529, 13.39282139548194195, -31.19999999999996376 ) ) ;
#24902=CARTESIAN_POINT ( 'NONE',  ( -4.318543150850367773, 18.18399003996480801, -55.94999999999997442 ) ) ;
#24904=CARTESIAN_POINT ( 'NONE',  ( 4.103766977300021601, 21.39838383358913987, -46.50704692567387610 ) ) ;
#24905=CARTESIAN_POINT ( 'NONE',  ( -5.041649132594344884, 20.06884854047834921, -32.09999999999996589 ) ) ;
#24907=CARTESIAN_POINT ( 'NONE',  ( -0.6839900399647736995, 21.81854315085035623, -71.54999999999994031 ) ) ;
#24918=CARTESIAN_POINT ( 'NONE',  ( -2.837105286290963146, 12.26822144673588255, -29.85704692567387397 ) ) ;
#24924=CARTESIAN_POINT ( 'NONE',  ( 0.7417250638684235176, 23.11142975074950101, -49.19295307432605568 ) ) ;
#24942=CARTESIAN_POINT ( 'NONE',  ( -5.107581180293630396, 19.93944961101426827, -72.59295307432606137 ) ) ;
#24947=CARTESIAN_POINT ( 'NONE',  ( 1.758463861404912620, 13.72892860598888731, -44.40704692567387468 ) ) ;
#24948=CARTESIAN_POINT ( 'NONE',  ( -3.705139346311794313, 19.38786279086902198, -32.09999999999996589 ) ) ;
#24949=CARTESIAN_POINT ( 'NONE',  ( 3.895814058185739448, 19.48501640914375344, -60.14999999999995595 ) ) ;
#24960=CARTESIAN_POINT ( 'NONE',  ( 2.983759233219601459, 14.30028814967311668, -26.25704692567387255 ) ) ;
#24961=CARTESIAN_POINT ( 'NONE',  ( 4.206979645153768210, 13.29302035484617406, -66.74999999999997158 ) ) ;
#24971=CARTESIAN_POINT ( 'NONE',  ( 5.852430833189966819, 16.41846101382252243, -52.95704692567387895 ) ) ;
#24974=CARTESIAN_POINT ( 'NONE',  ( 2.568848540478311460, 12.45835086740561692, -27.89999999999996660 ) ) ;
#24990=CARTESIAN_POINT ( 'NONE',  ( -4.206979645153768210, 21.70697964515380107, -47.24999999999995026 ) ) ;
#24995=CARTESIAN_POINT ( 'NONE',  ( -2.983759233219601903, 20.69971185032686023, -72.75704692567386189 ) ) ;
#24996=CARTESIAN_POINT ( 'NONE',  ( 0.6505131845895220088, 21.60717860451803674, -56.69999999999997442 ) ) ;
#25003=CARTESIAN_POINT ( 'NONE',  ( -3.895814058185739448, 15.51498359085620571, -73.64999999999993463 ) ) ;
#25007=CARTESIAN_POINT ( 'NONE',  ( 4.318543150850367773, 16.81600996003516357, -72.44999999999994600 ) ) ;
#25010=CARTESIAN_POINT ( 'NONE',  ( -3.771071394011080269, 19.25846386140493394, -45.59295307432606137 ) ) ;
#25025=CARTESIAN_POINT ( 'NONE',  ( -5.588711115410763597, 16.61483511785016987, -61.79999999999996874 ) ) ;
#25045=CARTESIAN_POINT ( 'NONE',  ( 5.565992480072003978, 18.52860470043125574, -49.79295307432606421 ) ) ;
#25053=CARTESIAN_POINT ( 'NONE',  ( 0.5070733663080689846, 21.62989723985679902, -67.19295307432605568 ) ) ;
#25068=CARTESIAN_POINT ( 'NONE',  ( -3.091735541773221296, 20.59173554177323950, -47.24999999999995026 ) ) ;
#25092=CARTESIAN_POINT ( 'NONE',  ( 3.091735541773220852, 14.40826445822673740, -27.74999999999995737 ) ) ;
#25098=CARTESIAN_POINT ( 'NONE',  ( 0.6839900399647733664, 13.18145684914961357, -34.04999999999995453 ) ) ;
#25107=CARTESIAN_POINT ( 'NONE',  ( 3.895814058185739448, 19.48501640914375344, -60.14999999999995595 ) ) ;
#25109=CARTESIAN_POINT ( 'NONE',  ( -0.7798958854283041253, 23.40020640687986386, -46.05704692567387326 ) ) ;
#25110=CARTESIAN_POINT ( 'NONE',  ( 0.9307174358028527106, 11.62368137996505801, -34.04999999999996163 ) ) ;
#25112=CARTESIAN_POINT ( 'NONE',  ( 3.826489000663266360, 19.62107449533211678, -28.64295307432606208 ) ) ;
#25123=CARTESIAN_POINT ( 'NONE',  ( 4.103766977300021601, 21.39838383358913987, -25.50704692567387610 ) ) ;
#25129=CARTESIAN_POINT ( 'NONE',  ( 1.081538986177402295, 11.64756916681001186, -41.54295307432605000 ) ) ;
#25147=CARTESIAN_POINT ( 'NONE',  ( 2.564989113914249330, 22.87042866830903876, -70.34295307432606137 ) ) ;
#25152=CARTESIAN_POINT ( 'NONE',  ( -3.091735541773221296, 20.59173554177323950, -38.24999999999996447 ) ) ;
#25153=CARTESIAN_POINT ( 'NONE',  ( -1.985016409143819605, 13.60418594181426855, -67.34999999999996589 ) ) ;
#25164=CARTESIAN_POINT ( 'NONE',  ( -3.043106805520194413, 14.66227633819065623, -30.00704692567387610 ) ) ;
#25165=CARTESIAN_POINT ( 'NONE',  ( -5.301103610786608300, 14.79895279989743528, -64.64999999999996305 ) ) ;
#25180=CARTESIAN_POINT ( 'NONE',  ( -4.103766977300021601, 13.60161616641083704, -54.00704692567387610 ) ) ;
#25184=CARTESIAN_POINT ( 'NONE',  ( 5.900206406879871857, 16.72010411457162604, -67.94295307432605568 ) ) ;
#25199=CARTESIAN_POINT ( 'NONE',  ( -4.206979645153768210, 21.70697964515380107, -50.24999999999997158 ) ) ;
#25203=CARTESIAN_POINT ( 'NONE',  ( -3.043106805520194413, 14.66227633819065623, -63.00704692567389031 ) ) ;
#25204=CARTESIAN_POINT ( 'NONE',  ( -0.6839900399647738105, 21.81854315085035623, -56.54999999999996874 ) ) ;
#25208=CARTESIAN_POINT ( 'NONE',  ( -0.6839900399647736995, 21.81854315085035623, -71.54999999999994031 ) ) ;
#25210=CARTESIAN_POINT ( 'NONE',  ( -0.5331684895902242260, 21.84243093769531185, -52.05704692567388747 ) ) ;
#25213=CARTESIAN_POINT ( 'NONE',  ( -4.107178604518053611, 16.84948681541050775, -73.79999999999996874 ) ) ;
#25216=CARTESIAN_POINT ( 'NONE',  ( -4.084459969179292216, 16.70604699712905372, -42.29295307432605711 ) ) ;
#25229=CARTESIAN_POINT ( 'NONE',  ( 4.206979645153767322, 13.29302035484617051, -54.74999999999997158 ) ) ;
#25252=CARTESIAN_POINT ( 'NONE',  ( -0.7417250638684240727, 11.88857024925047057, -44.69295307432606279 ) ) ;
#25259=CARTESIAN_POINT ( 'NONE',  ( 3.826489000663266360, 19.62107449533211678, -58.64295307432606563 ) ) ;
#25273=CARTESIAN_POINT ( 'NONE',  ( 0.6505131845895220088, 21.60717860451803674, -38.69999999999996021 ) ) ;
#25300=CARTESIAN_POINT ( 'NONE',  ( -3.895814058185739892, 15.51498359085620748, -31.64999999999996660 ) ) ;
#25304=CARTESIAN_POINT ( 'NONE',  ( -1.081538986177402961, 23.35243083318996327, -31.04295307432605355 ) ) ;
#25305=CARTESIAN_POINT ( 'NONE',  ( -4.129897239856814117, 16.99292663369196177, -69.30704692567387326 ) ) ;
#25314=CARTESIAN_POINT ( 'NONE',  ( -4.318543150850367773, 18.18399003996480801, -58.94999999999995310 ) ) ;
#25318=CARTESIAN_POINT ( 'NONE',  ( 1.028604700431328567, 23.06599248007198355, -34.20704692567387184 ) ) ;
#25319=CARTESIAN_POINT ( 'NONE',  ( -5.876318620034919782, 18.43071743580290089, -25.94999999999996732 ) ) ;
#25321=CARTESIAN_POINT ( 'NONE',  ( -0.6505131845895224529, 13.39282139548194195, -73.19999999999997442 ) ) ;
#25324=AXIS2_PLACEMENT_3D ( 'NONE', #15460, #8643, #37993 ) ;
#25333=CARTESIAN_POINT ( 'NONE',  ( 5.852430833189966819, 16.41846101382252243, -28.95704692567387184 ) ) ;
#25338=CARTESIAN_POINT ( 'NONE',  ( -1.081538986177402961, 23.35243083318996327, -40.04295307432605000 ) ) ;
#25357=CARTESIAN_POINT ( 'NONE',  ( -5.900206406879871857, 18.27989588542834554, -63.44295307432605568 ) ) ;
#25364=CARTESIAN_POINT ( 'NONE',  ( 3.895814058185739448, 19.48501640914375344, -36.14999999999994884 ) ) ;
#25365=CARTESIAN_POINT ( 'NONE',  ( -4.318543150850367773, 18.18399003996480801, -58.94999999999995310 ) ) ;
#25376=CARTESIAN_POINT ( 'NONE',  ( -4.294655364005415699, 18.33481159033935626, -27.45704692567386829 ) ) ;
#25377=CARTESIAN_POINT ( 'NONE',  ( 2.568848540478311460, 12.45835086740561692, -51.89999999999997016 ) ) ;
#25390=CARTESIAN_POINT ( 'NONE',  ( -4.103766977300021601, 13.60161616641083704, -57.00704692567387610 ) ) ;
#25393=CARTESIAN_POINT ( 'NONE',  ( -2.564989113914250662, 12.12957133169093282, -65.84295307432604716 ) ) ;
#25408=CARTESIAN_POINT ( 'NONE',  ( -4.001075405444606936, 13.49892459455542060, -37.49999999999996447 ) ) ;
#25413=CARTESIAN_POINT ( 'NONE',  ( 1.758463861404912620, 13.72892860598888731, -62.40704692567388179 ) ) ;
#25414=CARTESIAN_POINT ( 'NONE',  ( -1.985016409143819605, 13.60418594181426855, -58.34999999999996589 ) ) ;
#25422=CARTESIAN_POINT ( 'NONE',  ( 2.940415233664778416, 20.44041523366473712, -62.99999999999997158 ) ) ;
#25424=CARTESIAN_POINT ( 'NONE',  ( 4.129897239856814117, 18.00707336630801336, -58.80704692567387326 ) ) ;
#25427=CARTESIAN_POINT ( 'NONE',  ( 0.5070733663080689846, 21.62989723985679902, -28.19295307432605568 ) ) ;
#25431=CARTESIAN_POINT ( 'NONE',  ( -3.199711850326840246, 20.48375923321962233, -45.74295307432605995 ) ) ;
#25447=CARTESIAN_POINT ( 'NONE',  ( -5.041649132594344884, 20.06884854047834921, -44.09999999999996589 ) ) ;
#25467=CARTESIAN_POINT ( 'NONE',  ( -0.6505131845895224529, 13.39282139548194195, -46.19999999999996021 ) ) ;
#25468=CARTESIAN_POINT ( 'NONE',  ( 5.107581180293630396, 15.06055038898570686, -44.09295307432605426 ) ) ;
#25478=CARTESIAN_POINT ( 'NONE',  ( -2.837723661809363751, 14.45689319447982335, -59.99295307432606705 ) ) ;
#25494=CARTESIAN_POINT ( 'NONE',  ( 0.6839900399647733664, 13.18145684914961357, -37.04999999999996163 ) ) ;
#25517=CARTESIAN_POINT ( 'NONE',  ( 1.887862790868997109, 13.79486065368817194, -33.89999999999996305 ) ) ;
#25521=CARTESIAN_POINT ( 'NONE',  ( -5.107581180293630396, 19.93944961101426827, -33.59295307432606137 ) ) ;
#25523=CARTESIAN_POINT ( 'NONE',  ( 0.6505131845895220088, 21.60717860451803674, -29.69999999999996376 ) ) ;
#25530=CARTESIAN_POINT ( 'NONE',  ( -4.107178604518053611, 16.84948681541050775, -43.79999999999996163 ) ) ;
#25533=CARTESIAN_POINT ( 'NONE',  ( 2.439449611014226971, 12.39241881970633230, -38.40704692567386758 ) ) ;
#25534=CARTESIAN_POINT ( 'NONE',  ( 5.588711115410763597, 18.38516488214980882, -27.29999999999996163 ) ) ;
#25535=CARTESIAN_POINT ( 'NONE',  ( 4.318543150850367773, 16.81600996003516357, -66.44999999999997442 ) ) ;
#25547=CARTESIAN_POINT ( 'NONE',  ( 4.099003336600150149, 13.18504404629255689, -26.25704692567387255 ) ) ;
#25551=CARTESIAN_POINT ( 'NONE',  ( 5.107581180293630396, 15.06055038898570686, -44.09295307432605426 ) ) ;
#25567=CARTESIAN_POINT ( 'NONE',  ( 3.898383833589191383, 21.60376697729997275, -61.49295307432606705 ) ) ;
#25573=CARTESIAN_POINT ( 'NONE',  ( -1.985016409143819605, 13.60418594181426855, -55.34999999999997300 ) ) ;
#25584=CARTESIAN_POINT ( 'NONE',  ( 4.099003336600150149, 13.18504404629255689, -65.25704692567387610 ) ) ;
#25585=CARTESIAN_POINT ( 'NONE',  ( -0.8851648821498765418, 11.91128888458923285, -55.19999999999997442 ) ) ;
#25597=CARTESIAN_POINT ( 'NONE',  ( 5.611429750749524992, 18.24172506386835479, -58.80704692567387326 ) ) ;
#25600=CARTESIAN_POINT ( 'NONE',  ( -2.564989113914250662, 12.12957133169093282, -71.84295307432606137 ) ) ;
#25618=CARTESIAN_POINT ( 'NONE',  ( -0.9307174358028533767, 23.37631862003491889, -41.54999999999996874 ) ) ;
#25622=CARTESIAN_POINT ( 'NONE',  ( 3.639207298612508801, 15.48273827966686866, -62.10704692567388463 ) ) ;
#25623=CARTESIAN_POINT ( 'NONE',  ( -2.940415233664778860, 14.55958476633523802, -52.49999999999996447 ) ) ;
#25632=CARTESIAN_POINT ( 'NONE',  ( 3.895814058185739448, 19.48501640914375344, -66.14999999999997726 ) ) ;
#25634=CARTESIAN_POINT ( 'NONE',  ( -2.983759233219601903, 20.69971185032686023, -42.75704692567387610 ) ) ;
#25637=CARTESIAN_POINT ( 'NONE',  ( 2.017261720333081598, 13.86079270138745834, -29.39295307432606208 ) ) ;
#25640=CARTESIAN_POINT ( 'NONE',  ( -0.5070733663080690956, 13.37010276014318144, -47.69295307432606279 ) ) ;
#25654=CARTESIAN_POINT ( 'NONE',  ( -5.588711115410763597, 16.61483511785016987, -49.79999999999996874 ) ) ;
#25671=CARTESIAN_POINT ( 'NONE',  ( -4.001075405444606936, 13.49892459455542060, -73.49999999999997158 ) ) ;
#25676=CARTESIAN_POINT ( 'NONE',  ( 0.6505131845895220088, 21.60717860451803674, -41.69999999999996732 ) ) ;
#25677=CARTESIAN_POINT ( 'NONE',  ( 4.318543150850366885, 16.81600996003516713, -72.44999999999996021 ) ) ;
#25685=CARTESIAN_POINT ( 'NONE',  ( -2.837723661809363751, 14.45689319447982335, -53.99295307432605995 ) ) ;
#25700=CARTESIAN_POINT ( 'NONE',  ( -2.940415233664778860, 14.55958476633523802, -34.49999999999997158 ) ) ;
#25725=CARTESIAN_POINT ( 'NONE',  ( 3.043106805520193525, 20.33772366180932067, -34.50704692567386900 ) ) ;
#25726=CARTESIAN_POINT ( 'NONE',  ( -4.107178604518053611, 16.84948681541050775, -25.79999999999996163 ) ) ;
#25729=CARTESIAN_POINT ( 'NONE',  ( -5.231778553264134324, 14.66289471370907727, -30.14295307432606208 ) ) ;
#25730=CARTESIAN_POINT ( 'NONE',  ( 2.983759233219601459, 14.30028814967311668, -71.25704692567387610 ) ) ;
#25738=CARTESIAN_POINT ( 'NONE',  ( 1.985016409143818272, 21.39581405818570303, -44.84999999999996589 ) ) ;
#25741=CARTESIAN_POINT ( 'NONE',  ( 2.837105286290961370, 22.73177855326409613, -37.35704692567387752 ) ) ;
#25742=CARTESIAN_POINT ( 'NONE',  ( -0.9307174358028534877, 23.37631862003491889, -26.54999999999996163 ) ) ;
#25743=CARTESIAN_POINT ( 'NONE',  ( 3.895814058185739448, 19.48501640914375344, -63.14999999999997016 ) ) ;
#25753=EDGE_LOOP ( 'NONE', ( #6638, #23832, #26808, #8066 ) ) ;
#25757=CARTESIAN_POINT ( 'NONE',  ( 1.081538986177402295, 11.64756916681001186, -44.54295307432605711 ) ) ;
#25771=CARTESIAN_POINT ( 'NONE',  ( -2.564989113914250662, 12.12957133169093282, -65.84295307432604716 ) ) ;
#25776=CARTESIAN_POINT ( 'NONE',  ( -2.940415233664778860, 14.55958476633523802, -25.49999999999996803 ) ) ;
#25777=CARTESIAN_POINT ( 'NONE',  ( -3.705139346311794313, 19.38786279086902198, -59.09999999999997300 ) ) ;
#25790=CARTESIAN_POINT ( 'NONE',  ( -4.099003336600151925, 21.81495595370741469, -66.75704692567384768 ) ) ;
#25791=CARTESIAN_POINT ( 'NONE',  ( 5.041649132594343996, 14.93115145952162415, -54.59999999999996589 ) ) ;
#25804=CARTESIAN_POINT ( 'NONE',  ( 4.975717084895059372, 14.80175253005754143, -59.10704692567387752 ) ) ;
#25808=CARTESIAN_POINT ( 'NONE',  ( 1.081538986177402295, 11.64756916681001186, -71.54295307432605000 ) ) ;
#25826=CARTESIAN_POINT ( 'NONE',  ( 2.568848540478311460, 12.45835086740561692, -45.89999999999997016 ) ) ;
#25830=CARTESIAN_POINT ( 'NONE',  ( 4.294655364005415699, 16.66518840966061887, -58.95704692567386473 ) ) ;
#25831=CARTESIAN_POINT ( 'NONE',  ( 3.895814058185739892, 19.48501640914376054, -48.14999999999997016 ) ) ;
#25839=CARTESIAN_POINT ( 'NONE',  ( -4.107178604518053611, 16.84948681541050775, -67.79999999999996874 ) ) ;
#25841=CARTESIAN_POINT ( 'NONE',  ( -4.294655364005415699, 18.33481159033935626, -42.45704692567387184 ) ) ;
#25847=CARTESIAN_POINT ( 'NONE',  ( 2.017261720333081598, 13.86079270138745834, -41.39295307432605853 ) ) ;
#25860=CARTESIAN_POINT ( 'NONE',  ( -2.568848540478311904, 22.54164913259435465, -44.39999999999997016 ) ) ;
#25877=CARTESIAN_POINT ( 'NONE',  ( 5.301103610786608300, 20.20104720010253985, -72.14999999999996305 ) ) ;
#25882=CARTESIAN_POINT ( 'NONE',  ( 4.107178604518054499, 18.15051318458946383, -45.29999999999996874 ) ) ;
#25892=CARTESIAN_POINT ( 'NONE',  ( 3.771071394011080269, 15.74153613859503764, -59.09295307432605426 ) ) ;
#25907=CARTESIAN_POINT ( 'NONE',  ( -4.318543150850367773, 18.18399003996480801, -31.94999999999994955 ) ) ;
#25935=CARTESIAN_POINT ( 'NONE',  ( 3.043106805520193525, 20.33772366180932067, -31.50704692567387610 ) ) ;
#25940=CARTESIAN_POINT ( 'NONE',  ( -2.564989113914250662, 12.12957133169093282, -35.84295307432606137 ) ) ;
#25941=CARTESIAN_POINT ( 'NONE',  ( -0.6839900399647736995, 21.81854315085035623, -29.54999999999996518 ) ) ;
#25949=CARTESIAN_POINT ( 'NONE',  ( 4.107178604518054499, 18.15051318458946383, -45.29999999999996874 ) ) ;
#25953=CARTESIAN_POINT ( 'NONE',  ( 0.7798958854283032371, 11.59979359312010772, -38.55704692567387326 ) ) ;
#25970=CARTESIAN_POINT ( 'NONE',  ( -1.081538986177402961, 23.35243083318996327, -37.04295307432605711 ) ) ;
#25990=CARTESIAN_POINT ( 'NONE',  ( 2.940415233664778416, 20.44041523366473712, -53.99999999999996447 ) ) ;
#26000=CARTESIAN_POINT ( 'NONE',  ( -1.028604700431329233, 11.93400751992799513, -65.70704692567387895 ) ) ;
#26001=CARTESIAN_POINT ( 'NONE',  ( -0.9307174358028534877, 23.37631862003491889, -56.54999999999996874 ) ) ;
#26013=CARTESIAN_POINT ( 'NONE',  ( -5.611429750749524992, 16.75827493613162034, -42.30704692567387326 ) ) ;
#26016=CARTESIAN_POINT ( 'NONE',  ( -5.107581180293630396, 19.93944961101426827, -69.59295307432604716 ) ) ;
#26034=CARTESIAN_POINT ( 'NONE',  ( 5.041649132594343996, 14.93115145952162415, -42.59999999999996589 ) ) ;
#26037=CARTESIAN_POINT ( 'NONE',  ( 2.121074495332174958, 21.32648900066323350, -64.35704692567387042 ) ) ;
#26039=CARTESIAN_POINT ( 'NONE',  ( 1.887862790868997109, 13.79486065368817194, -45.89999999999997016 ) ) ;
#26047=CARTESIAN_POINT ( 'NONE',  ( 4.318543150850367773, 16.81600996003516357, -63.44999999999996732 ) ) ;
#26051=CARTESIAN_POINT ( 'NONE',  ( -2.983759233219601903, 20.69971185032686023, -45.75704692567386900 ) ) ;
#26056=CARTESIAN_POINT ( 'NONE',  ( -3.771071394011080269, 19.25846386140493394, -39.59295307432606137 ) ) ;
#26070=CARTESIAN_POINT ( 'NONE',  ( 0.8851648821498760977, 23.08871111541074228, -47.69999999999996732 ) ) ;
#26086=CARTESIAN_POINT ( 'NONE',  ( -0.9307174358028533767, 23.37631862003491889, -71.54999999999994031 ) ) ;
#26091=CARTESIAN_POINT ( 'NONE',  ( 4.318543150850367773, 16.81600996003516357, -45.44999999999996021 ) ) ;
#26103=CARTESIAN_POINT ( 'NONE',  ( 0.5070733663080689846, 21.62989723985679902, -55.19295307432606279 ) ) ;
#26119=CARTESIAN_POINT ( 'NONE',  ( -3.705139346311794313, 19.38786279086902198, -35.09999999999996589 ) ) ;
#26149=CARTESIAN_POINT ( 'NONE',  ( -0.5331684895902242260, 21.84243093769531185, -37.05704692567387326 ) ) ;
#26153=CARTESIAN_POINT ( 'NONE',  ( 5.107581180293630396, 15.06055038898570686, -38.09295307432605426 ) ) ;
#26154=CARTESIAN_POINT ( 'NONE',  ( 4.318543150850367773, 16.81600996003516357, -27.44999999999996021 ) ) ;
#26161=CARTESIAN_POINT ( 'NONE',  ( 2.940415233664778416, 20.44041523366473712, -41.99999999999996447 ) ) ;
#26164=CARTESIAN_POINT ( 'NONE',  ( -5.370428668309080500, 14.93501088608579153, -39.15704692567386758 ) ) ;
#26165=CARTESIAN_POINT ( 'NONE',  ( -0.8851648821498765418, 11.91128888458923285, -31.19999999999996376 ) ) ;
#26166=CARTESIAN_POINT ( 'NONE',  ( -4.318543150850367773, 18.18399003996480801, -61.94999999999997442 ) ) ;
#26180=CARTESIAN_POINT ( 'NONE',  ( -5.231778553264134324, 14.66289471370907727, -33.14295307432605853 ) ) ;
#26201=CARTESIAN_POINT ( 'NONE',  ( -1.887862790868997553, 21.20513934631180319, -53.39999999999997016 ) ) ;
#26211=CARTESIAN_POINT ( 'NONE',  ( 0.7798958854283032371, 11.59979359312010772, -62.55704692567387326 ) ) ;
#26212=CARTESIAN_POINT ( 'NONE',  ( -2.701047200102606460, 12.19889638921340591, -58.34999999999996589 ) ) ;
#26224=CARTESIAN_POINT ( 'NONE',  ( 5.611429750749524992, 18.24172506386835479, -46.80704692567388037 ) ) ;
#26229=CARTESIAN_POINT ( 'NONE',  ( 1.081538986177402295, 11.64756916681001186, -56.54295307432606421 ) ) ;
#26246=CARTESIAN_POINT ( 'NONE',  ( -4.001075405444606936, 13.49892459455542060, -43.49999999999997158 ) ) ;
#26249=CARTESIAN_POINT ( 'NONE',  ( -2.983759233219601903, 20.69971185032686023, -57.75704692567386900 ) ) ;
#26250=CARTESIAN_POINT ( 'NONE',  ( -3.091735541773221296, 20.59173554177323950, -47.24999999999995737 ) ) ;
#26259=CARTESIAN_POINT ( 'NONE',  ( -0.6839900399647736995, 21.81854315085035623, -68.54999999999998295 ) ) ;
#26261=CARTESIAN_POINT ( 'NONE',  ( -1.758463861404912842, 21.27107139401109137, -45.90704692567387468 ) ) ;
#26265=CARTESIAN_POINT ( 'NONE',  ( -4.084459969179292216, 16.70604699712905372, -36.29295307432605000 ) ) ;
#26273=CARTESIAN_POINT ( 'NONE',  ( 0.7798958854283032371, 11.59979359312010772, -71.55704692567385905 ) ) ;
#26278=CARTESIAN_POINT ( 'NONE',  ( 4.206979645153767322, 13.29302035484617051, -36.74999999999994316 ) ) ;
#26297=CARTESIAN_POINT ( 'NONE',  ( 4.001075405444606048, 21.50107540544455276, -74.99999999999997158 ) ) ;
#26302=CARTESIAN_POINT ( 'NONE',  ( -1.887862790868997553, 21.20513934631180319, -41.39999999999996305 ) ) ;
#26303=CARTESIAN_POINT ( 'NONE',  ( -1.985016409143819605, 13.60418594181426855, -73.34999999999996589 ) ) ;
#26312=CARTESIAN_POINT ( 'NONE',  ( -4.084459969179292216, 16.70604699712905372, -48.29295307432606421 ) ) ;
#26317=CARTESIAN_POINT ( 'NONE',  ( -4.084459969179292216, 16.70604699712905372, -60.29295307432605000 ) ) ;
#26328=CARTESIAN_POINT ( 'NONE',  ( -3.895814058185739448, 15.51498359085620571, -28.64999999999995950 ) ) ;
#26335=CARTESIAN_POINT ( 'NONE',  ( -4.001075405444606936, 13.49892459455542060, -73.49999999999997158 ) ) ;
#26352=CARTESIAN_POINT ( 'NONE',  ( -0.7939530028709754772, 13.41554003082070246, -29.70704692567387184 ) ) ;
#26356=CARTESIAN_POINT ( 'NONE',  ( 2.564989113914249330, 22.87042866830903876, -28.34295307432605426 ) ) ;
#26357=CARTESIAN_POINT ( 'NONE',  ( -0.5331684895902242260, 21.84243093769531185, -67.05704692567387326 ) ) ;
#26364=CARTESIAN_POINT ( 'NONE',  ( -4.318543150850367773, 18.18399003996480801, -46.94999999999996021 ) ) ;
#26367=CARTESIAN_POINT ( 'NONE',  ( 5.852430833189966819, 16.41846101382252243, -31.95704692567387184 ) ) ;
#26369=CARTESIAN_POINT ( 'NONE',  ( 4.318543150850367773, 16.81600996003516357, -60.44999999999997442 ) ) ;
#26382=CARTESIAN_POINT ( 'NONE',  ( 5.565992480072003978, 18.52860470043125574, -31.79295307432605355 ) ) ;
#26401=CARTESIAN_POINT ( 'NONE',  ( 2.940415233664778416, 20.44041523366473712, -41.99999999999996447 ) ) ;
#26409=CARTESIAN_POINT ( 'NONE',  ( -4.084459969179292216, 16.70604699712905372, -30.29295307432605355 ) ) ;
#26411=CARTESIAN_POINT ( 'NONE',  ( 5.370428668309080500, 20.06498911391418360, -64.65704692567386758 ) ) ;
#26412=CARTESIAN_POINT ( 'NONE',  ( 5.876318620034919782, 16.56928256419707068, -42.44999999999996732 ) ) ;
#26425=CARTESIAN_POINT ( 'NONE',  ( 4.103766977300021601, 21.39838383358913987, -40.50704692567387610 ) ) ;
#26432=CARTESIAN_POINT ( 'NONE',  ( -2.564989113914250662, 12.12957133169093282, -62.84295307432604716 ) ) ;
#26446=CARTESIAN_POINT ( 'NONE',  ( -0.8851648821498765418, 11.91128888458923285, -28.19999999999996732 ) ) ;
#26449=CARTESIAN_POINT ( 'NONE',  ( 0.7939530028709752552, 21.58445996917927445, -49.20704692567387184 ) ) ;
#26450=CARTESIAN_POINT ( 'NONE',  ( -0.6505131845895224529, 13.39282139548194195, -46.19999999999996021 ) ) ;
#26460=CARTESIAN_POINT ( 'NONE',  ( -2.940415233664778860, 14.55958476633523802, -52.49999999999996447 ) ) ;
#26463=CARTESIAN_POINT ( 'NONE',  ( 2.983759233219601459, 14.30028814967311668, -47.25704692567386900 ) ) ;
#26467=CARTESIAN_POINT ( 'NONE',  ( -0.5070733663080690956, 13.37010276014318144, -35.69295307432606279 ) ) ;
#26474=CARTESIAN_POINT ( 'NONE',  ( 2.439449611014226971, 12.39241881970633230, -71.40704692567388179 ) ) ;
#26483=CARTESIAN_POINT ( 'NONE',  ( 0.8851648821498760977, 23.08871111541074228, -35.69999999999996732 ) ) ;
#26501=CARTESIAN_POINT ( 'NONE',  ( 2.568848540478311460, 12.45835086740561692, -57.89999999999996305 ) ) ;
#26506=CARTESIAN_POINT ( 'NONE',  ( -0.6505131845895224529, 13.39282139548194195, -34.19999999999996732 ) ) ;
#26518=CARTESIAN_POINT ( 'NONE',  ( 4.342430937695320736, 16.96683151040971538, -46.94295307432605568 ) ) ;
#26523=CARTESIAN_POINT ( 'NONE',  ( -0.5070733663080690956, 13.37010276014318144, -62.69295307432606279 ) ) ;
#26544=CARTESIAN_POINT ( 'NONE',  ( 2.701047200102605572, 22.80110361078655856, -62.84999999999995879 ) ) ;
#26554=DIRECTION ( 'NONE',  ( -0.7071067811865509034, -0.7071067811865441310, 0.000000000000000000 ) ) ;
#26558=CARTESIAN_POINT ( 'NONE',  ( -5.565992480072003978, 16.47139529956871229, -66.29295307432606421 ) ) ;
#26562=CARTESIAN_POINT ( 'NONE',  ( 4.129897239856814117, 18.00707336630801336, -37.80704692567387326 ) ) ;
#26566=CARTESIAN_POINT ( 'NONE',  ( 2.017261720333081598, 13.86079270138745834, -74.39295307432605853 ) ) ;
#26567=CARTESIAN_POINT ( 'NONE',  ( -2.121074495332175847, 13.67351099933674341, -65.85704692567387042 ) ) ;
#26575=CARTESIAN_POINT ( 'NONE',  ( -1.985016409143819605, 13.60418594181426855, -40.34999999999996589 ) ) ;
#26579=CARTESIAN_POINT ( 'NONE',  ( -2.837105286290963146, 12.26822144673588255, -29.85704692567387397 ) ) ;
#26581=CARTESIAN_POINT ( 'NONE',  ( 2.940415233664778416, 20.44041523366473712, -50.99999999999997158 ) ) ;
#26593=CARTESIAN_POINT ( 'NONE',  ( 0.7417250638684235176, 23.11142975074950101, -31.19295307432605568 ) ) ;
#26612=CARTESIAN_POINT ( 'NONE',  ( 1.985016409143818272, 21.39581405818570303, -47.84999999999994458 ) ) ;
#26621=CARTESIAN_POINT ( 'NONE',  ( 2.940415233664778416, 20.44041523366473712, -65.99999999999997158 ) ) ;
#26623=CARTESIAN_POINT ( 'NONE',  ( 2.837105286290961370, 22.73177855326409613, -52.35704692567387042 ) ) ;
#26624=CARTESIAN_POINT ( 'NONE',  ( 0.8851648821498760977, 23.08871111541074228, -47.69999999999996732 ) ) ;
#26636=CARTESIAN_POINT ( 'NONE',  ( 4.099003336600150149, 13.18504404629255689, -41.25704692567387610 ) ) ;
#26643=CARTESIAN_POINT ( 'NONE',  ( -1.081538986177402961, 23.35243083318996327, -58.04295307432605711 ) ) ;
#26657=CARTESIAN_POINT ( 'NONE',  ( 4.206979645153767322, 13.29302035484617051, -33.74999999999996447 ) ) ;
#26660=CARTESIAN_POINT ( 'NONE',  ( -3.639207298612509689, 19.51726172033310647, -57.60704692567387752 ) ) ;
#26661=CARTESIAN_POINT ( 'NONE',  ( 3.091735541773220852, 14.40826445822673740, -42.74999999999997158 ) ) ;
#26662=CARTESIAN_POINT ( 'NONE',  ( -4.107178604518053611, 16.84948681541050775, -73.79999999999996874 ) ) ;
#26671=CARTESIAN_POINT ( 'NONE',  ( 2.940415233664778416, 20.44041523366473712, -50.99999999999997158 ) ) ;
#26673=CARTESIAN_POINT ( 'NONE',  ( 3.965139115708213868, 19.34895832295540430, -34.65704692567386758 ) ) ;
#26674=CARTESIAN_POINT ( 'NONE',  ( 4.001075405444606048, 21.50107540544455276, -71.99999999999997158 ) ) ;
#26677=CARTESIAN_POINT ( 'NONE',  ( 3.826489000663266360, 19.62107449533211678, -37.64295307432604432 ) ) ;
#26686=CARTESIAN_POINT ( 'NONE',  ( -0.7798958854283041253, 23.40020640687986386, -73.05704692567387326 ) ) ;
#26692=CARTESIAN_POINT ( 'NONE',  ( -5.876318620034919782, 18.43071743580290089, -37.94999999999996021 ) ) ;
#26710=CARTESIAN_POINT ( 'NONE',  ( 0.8851648821498760977, 23.08871111541074228, -56.69999999999997442 ) ) ;
#26716=CARTESIAN_POINT ( 'NONE',  ( -3.705139346311794313, 19.38786279086902198, -35.09999999999996589 ) ) ;
#26717=CARTESIAN_POINT ( 'NONE',  ( 0.6839900399647732554, 13.18145684914961357, -67.04999999999995453 ) ) ;
#26732=CARTESIAN_POINT ( 'NONE',  ( -3.771071394011080269, 19.25846386140493394, -42.59295307432605426 ) ) ;
#26737=CARTESIAN_POINT ( 'NONE',  ( 4.084459969179292216, 18.29395300287091430, -61.79295307432605000 ) ) ;
#26748=CARTESIAN_POINT ( 'NONE',  ( -4.107178604518053611, 16.84948681541050775, -28.79999999999996518 ) ) ;
#26756=CARTESIAN_POINT ( 'NONE',  ( -4.001075405444606936, 13.49892459455542060, -70.49999999999997158 ) ) ;
#26774=CARTESIAN_POINT ( 'NONE',  ( -2.564989113914250662, 12.12957133169093282, -59.84295307432606137 ) ) ;
#26783=CARTESIAN_POINT ( 'NONE',  ( -1.081538986177402961, 23.35243083318996327, -28.04295307432605355 ) ) ;
#26784=CARTESIAN_POINT ( 'NONE',  ( -3.043106805520194413, 14.66227633819065623, -69.00704692567386189 ) ) ;
#26797=CARTESIAN_POINT ( 'NONE',  ( 1.028604700431328567, 23.06599248007198355, -28.20704692567387184 ) ) ;
#26799=CARTESIAN_POINT ( 'NONE',  ( -0.6839900399647736995, 21.81854315085035623, -53.54999999999996163 ) ) ;
#26808=ORIENTED_EDGE ( 'NONE', *, *, #2342, .T. ) ;
#26810=CARTESIAN_POINT ( 'NONE',  ( 5.231778553264135212, 20.33710528629089254, -34.64295307432605142 ) ) ;
#26827=CARTESIAN_POINT ( 'NONE',  ( 0.6505131845895220088, 21.60717860451803674, -41.69999999999996732 ) ) ;
#26835=CARTESIAN_POINT ( 'NONE',  ( 0.6839900399647733664, 13.18145684914961357, -70.04999999999996874 ) ) ;
#26837=CARTESIAN_POINT ( 'NONE',  ( -0.7798958854283041253, 23.40020640687986386, -61.05704692567386616 ) ) ;
#26838=CARTESIAN_POINT ( 'NONE',  ( 2.701047200102605128, 22.80110361078656211, -47.84999999999995168 ) ) ;
#26852=CARTESIAN_POINT ( 'NONE',  ( -2.837105286290963146, 12.26822144673588255, -44.85704692567387752 ) ) ;
#26856=CARTESIAN_POINT ( 'NONE',  ( 0.7417250638684235176, 23.11142975074950101, -64.19295307432605568 ) ) ;
#26871=CARTESIAN_POINT ( 'NONE',  ( 5.041649132594343996, 14.93115145952162415, -30.59999999999996589 ) ) ;
#26874=CARTESIAN_POINT ( 'NONE',  ( 3.043106805520193525, 20.33772366180932067, -52.50704692567387610 ) ) ;
#26876=CARTESIAN_POINT ( 'NONE',  ( 1.985016409143818272, 21.39581405818570303, -71.84999999999998010 ) ) ;
#26885=CARTESIAN_POINT ( 'NONE',  ( 2.940415233664778416, 20.44041523366473712, -56.99999999999996447 ) ) ;
#26887=CARTESIAN_POINT ( 'NONE',  ( 4.129897239856814117, 18.00707336630801336, -31.80704692567387326 ) ) ;
#26891=CARTESIAN_POINT ( 'NONE',  ( 4.342430937695320736, 16.96683151040971538, -37.94295307432606279 ) ) ;
#26897=CARTESIAN_POINT ( 'NONE',  ( 2.837105286290961370, 22.73177855326409613, -70.35704692567388463 ) ) ;
#26905=CARTESIAN_POINT ( 'NONE',  ( -0.8851648821498765418, 11.91128888458923285, -37.19999999999996732 ) ) ;
#26923=CARTESIAN_POINT ( 'NONE',  ( -2.701047200102606016, 12.19889638921340413, -58.34999999999995879 ) ) ;
#26928=CARTESIAN_POINT ( 'NONE',  ( 1.887862790868997109, 13.79486065368817194, -33.89999999999996305 ) ) ;
#26929=CARTESIAN_POINT ( 'NONE',  ( 4.318543150850366885, 16.81600996003516713, -66.44999999999997442 ) ) ;
#26942=CARTESIAN_POINT ( 'NONE',  ( -0.5070733663080690956, 13.37010276014318144, -47.69295307432606279 ) ) ;
#26947=CARTESIAN_POINT ( 'NONE',  ( -4.084459969179292216, 16.70604699712905372, -63.29295307432605000 ) ) ;
#26957=CARTESIAN_POINT ( 'NONE',  ( 4.107178604518054499, 18.15051318458946383, -30.29999999999996518 ) ) ;
#26964=CARTESIAN_POINT ( 'NONE',  ( 5.041649132594343996, 14.93115145952162415, -69.59999999999996589 ) ) ;
#26983=CARTESIAN_POINT ( 'NONE',  ( -0.7417250638684240727, 11.88857024925047057, -56.69295307432606279 ) ) ;
#26991=CARTESIAN_POINT ( 'NONE',  ( 5.900206406879871857, 16.72010411457162604, -28.94295307432605568 ) ) ;
#26993=CARTESIAN_POINT ( 'NONE',  ( -3.965139115708213868, 15.65104167704456906, -69.15704692567386758 ) ) ;
#27006=CARTESIAN_POINT ( 'NONE',  ( -4.975717084895059372, 20.19824746994243370, -30.60704692567387752 ) ) ;
#27008=CARTESIAN_POINT ( 'NONE',  ( -1.985016409143819605, 13.60418594181426855, -52.34999999999994458 ) ) ;
#27020=CARTESIAN_POINT ( 'NONE',  ( 2.837723661809363307, 20.54310680552015356, -70.49295307432603863 ) ) ;
#27039=CARTESIAN_POINT ( 'NONE',  ( -2.940415233664778860, 14.55958476633523802, -43.49999999999997158 ) ) ;
#27048=CARTESIAN_POINT ( 'NONE',  ( 1.985016409143818272, 21.39581405818570303, -62.84999999999995879 ) ) ;
#27050=CARTESIAN_POINT ( 'NONE',  ( 4.975717084895059372, 14.80175253005754143, -53.10704692567387752 ) ) ;
#27051=CARTESIAN_POINT ( 'NONE',  ( -5.301103610786608300, 14.79895279989743528, -43.64999999999996305 ) ) ;
#27064=CARTESIAN_POINT ( 'NONE',  ( 2.439449611014226971, 12.39241881970633230, -38.40704692567386758 ) ) ;
#27067=CARTESIAN_POINT ( 'NONE',  ( -2.564989113914250662, 12.12957133169093282, -56.84295307432604716 ) ) ;
#27081=CARTESIAN_POINT ( 'NONE',  ( -0.9307174358028533767, 23.37631862003491889, -29.54999999999996518 ) ) ;
#27084=CARTESIAN_POINT ( 'NONE',  ( 3.965139115708213868, 19.34895832295540430, -52.65704692567388179 ) ) ;
#27085=CARTESIAN_POINT ( 'NONE',  ( -0.6505131845895224529, 13.39282139548194195, -70.19999999999997442 ) ) ;
#27093=CARTESIAN_POINT ( 'NONE',  ( -0.6505131845895224529, 13.39282139548194195, -55.19999999999997442 ) ) ;
#27095=CARTESIAN_POINT ( 'NONE',  ( -0.7939530028709754772, 13.41554003082070246, -35.70704692567387184 ) ) ;
#27106=CARTESIAN_POINT ( 'NONE',  ( -4.975717084895059372, 20.19824746994243370, -69.60704692567387042 ) ) ;
#27111=CARTESIAN_POINT ( 'NONE',  ( 5.876318620034919782, 16.56928256419707068, -42.44999999999996732 ) ) ;
#27124=CARTESIAN_POINT ( 'NONE',  ( -4.001075405444606936, 13.49892459455542060, -25.49999999999996803 ) ) ;
#27128=CARTESIAN_POINT ( 'NONE',  ( -0.9307174358028533767, 23.37631862003491889, -59.54999999999994742 ) ) ;
#27133=CARTESIAN_POINT ( 'NONE',  ( -0.6505131845895224529, 13.39282139548194195, -37.19999999999996732 ) ) ;
#27134=CARTESIAN_POINT ( 'NONE',  ( 2.940415233664778416, 20.44041523366473712, -71.99999999999997158 ) ) ;
#27145=CARTESIAN_POINT ( 'NONE',  ( 0.5070733663080689846, 21.62989723985679902, -43.19295307432606279 ) ) ;
#27151=CARTESIAN_POINT ( 'NONE',  ( -3.771071394011080269, 19.25846386140493394, -63.59295307432605426 ) ) ;
#27171=CARTESIAN_POINT ( 'NONE',  ( -4.206979645153768210, 21.70697964515380107, -71.24999999999994316 ) ) ;
#27191=CARTESIAN_POINT ( 'NONE',  ( -3.898383833589191827, 13.39623302270000771, -53.99295307432605995 ) ) ;
#27202=CARTESIAN_POINT ( 'NONE',  ( -2.017261720333081598, 21.13920729861251857, -72.89295307432605853 ) ) ;
#27204=CARTESIAN_POINT ( 'NONE',  ( -2.121074495332175847, 13.67351099933674341, -62.85704692567387042 ) ) ;
#27218=CARTESIAN_POINT ( 'NONE',  ( -4.107178604518053611, 16.84948681541050775, -58.79999999999996163 ) ) ;
#27230=CARTESIAN_POINT ( 'NONE',  ( -0.8348115903393239501, 21.79465536400541126, -70.04295307432606421 ) ) ;
#27251=CARTESIAN_POINT ( 'NONE',  ( 3.895814058185739448, 19.48501640914375344, -48.14999999999997726 ) ) ;
#27261=CARTESIAN_POINT ( 'NONE',  ( 1.985016409143818272, 21.39581405818570303, -68.84999999999996589 ) ) ;
#27263=CARTESIAN_POINT ( 'NONE',  ( -2.439449611014227859, 22.60758118029364283, -60.90704692567388179 ) ) ;
#27264=CARTESIAN_POINT ( 'NONE',  ( -5.301103610786608300, 14.79895279989743528, -46.64999999999996305 ) ) ;
#27277=CARTESIAN_POINT ( 'NONE',  ( 5.852430833189966819, 16.41846101382252243, -34.95704692567387895 ) ) ;
#27280=CARTESIAN_POINT ( 'NONE',  ( -4.314955953707389824, 21.59900333660018390, -48.74295307432605284 ) ) ;
#27297=CARTESIAN_POINT ( 'NONE',  ( -0.9307174358028533767, 23.37631862003491889, -35.54999999999994742 ) ) ;
#27301=CARTESIAN_POINT ( 'NONE',  ( -0.7939530028709754772, 13.41554003082070246, -47.70704692567387184 ) ) ;
#27302=CARTESIAN_POINT ( 'NONE',  ( 3.091735541773220852, 14.40826445822673563, -69.74999999999997158 ) ) ;
#27308=CARTESIAN_POINT ( 'NONE',  ( 3.091735541773220852, 14.40826445822673563, -57.74999999999995737 ) ) ;
#27311=CARTESIAN_POINT ( 'NONE',  ( 2.121074495332174958, 21.32648900066323350, -40.35704692567387752 ) ) ;
#27312=CARTESIAN_POINT ( 'NONE',  ( -0.8851648821498765418, 11.91128888458923285, -73.19999999999997442 ) ) ;
#27323=CARTESIAN_POINT ( 'NONE',  ( -2.837105286290963146, 12.26822144673588255, -65.85704692567387042 ) ) ;
#27327=CARTESIAN_POINT ( 'NONE',  ( 0.8851648821498760977, 23.08871111541074228, -32.69999999999996732 ) ) ;
#27340=CARTESIAN_POINT ( 'NONE',  ( -0.9307174358028533767, 23.37631862003491889, -62.54999999999996874 ) ) ;
#27345=CARTESIAN_POINT ( 'NONE',  ( 0.6839900399647733664, 13.18145684914961357, -31.04999999999995808 ) ) ;
#27346=CARTESIAN_POINT ( 'NONE',  ( 0.6839900399647732554, 13.18145684914961357, -70.04999999999996874 ) ) ;
#27358=CARTESIAN_POINT ( 'NONE',  ( 3.199711850326839357, 14.51624076678035635, -32.24295307432605284 ) ) ;
#27364=CARTESIAN_POINT ( 'NONE',  ( 3.199711850326839357, 14.51624076678035635, -59.24295307432605995 ) ) ;
#27379=CARTESIAN_POINT ( 'NONE',  ( -5.588711115410763597, 16.61483511785016987, -70.79999999999996874 ) ) ;
#27401=CARTESIAN_POINT ( 'NONE',  ( -2.564989113914250662, 12.12957133169093282, -53.84295307432606137 ) ) ;
#27410=CARTESIAN_POINT ( 'NONE',  ( 2.017261720333081598, 13.86079270138745834, -62.39295307432605853 ) ) ;
#27413=CARTESIAN_POINT ( 'NONE',  ( -4.129897239856814117, 16.99292663369196177, -57.30704692567387326 ) ) ;
#27426=CARTESIAN_POINT ( 'NONE',  ( 0.6839900399647733664, 13.18145684914961357, -58.04999999999996874 ) ) ;
#27435=CARTESIAN_POINT ( 'NONE',  ( -5.565992480072003978, 16.47139529956871229, -27.29295307432605355 ) ) ;
#27451=CARTESIAN_POINT ( 'NONE',  ( -1.887862790868997553, 21.20513934631180319, -38.39999999999997016 ) ) ;
#27456=CARTESIAN_POINT ( 'NONE',  ( -2.940415233664778860, 14.55958476633523802, -34.49999999999997158 ) ) ;
#27465=CARTESIAN_POINT ( 'NONE',  ( -4.107178604518053611, 16.84948681541050775, -61.79999999999996874 ) ) ;
#27467=CARTESIAN_POINT ( 'NONE',  ( 5.611429750749524992, 18.24172506386835479, -58.80704692567387326 ) ) ;
#27468=CARTESIAN_POINT ( 'NONE',  ( 0.9307174358028527106, 11.62368137996505801, -40.04999999999996163 ) ) ;
#27482=CARTESIAN_POINT ( 'NONE',  ( 0.7798958854283032371, 11.59979359312010772, -38.55704692567387326 ) ) ;
#27487=CARTESIAN_POINT ( 'NONE',  ( -2.698247469942396837, 22.47571708489507358, -54.89295307432605853 ) ) ;
#27505=CARTESIAN_POINT ( 'NONE',  ( 3.898383833589191383, 21.60376697729997275, -70.49295307432603863 ) ) ;
#27508=CARTESIAN_POINT ( 'NONE',  ( -3.043106805520194413, 14.66227633819065623, -48.00704692567387610 ) ) ;
#27509=CARTESIAN_POINT ( 'NONE',  ( 3.705139346311793869, 15.61213720913094960, -72.59999999999996589 ) ) ;
#27518=CARTESIAN_POINT ( 'NONE',  ( 3.705139346311793869, 15.61213720913094960, -48.59999999999996589 ) ) ;
#27520=CARTESIAN_POINT ( 'NONE',  ( 1.758463861404912620, 13.72892860598888731, -38.40704692567386758 ) ) ;
#27521=CARTESIAN_POINT ( 'NONE',  ( -0.8851648821498765418, 11.91128888458923285, -70.19999999999997442 ) ) ;
#27533=CARTESIAN_POINT ( 'NONE',  ( 5.852430833189966819, 16.41846101382252243, -61.95704692567387895 ) ) ;
#27539=CARTESIAN_POINT ( 'NONE',  ( -5.301103610786608300, 14.79895279989743706, -31.64999999999995950 ) ) ;
#27555=CARTESIAN_POINT ( 'NONE',  ( 0.9307174358028528216, 11.62368137996505801, -55.04999999999995453 ) ) ;
#27558=CARTESIAN_POINT ( 'NONE',  ( -3.705139346311794313, 19.38786279086902198, -26.09999999999996234 ) ) ;
#27559=CARTESIAN_POINT ( 'NONE',  ( 4.107178604518054499, 18.15051318458946383, -72.29999999999996874 ) ) ;
#27565=CARTESIAN_POINT ( 'NONE',  ( 4.107178604518054499, 18.15051318458946383, -69.29999999999996874 ) ) ;
#27570=CARTESIAN_POINT ( 'NONE',  ( 3.826489000663266360, 19.62107449533211678, -40.64295307432606563 ) ) ;
#27573=CARTESIAN_POINT ( 'NONE',  ( -0.8348115903393239501, 21.79465536400541126, -52.04295307432606421 ) ) ;
#27587=CARTESIAN_POINT ( 'NONE',  ( -4.206979645153768210, 21.70697964515380107, -62.24999999999995737 ) ) ;
#27606=CARTESIAN_POINT ( 'NONE',  ( 2.698247469942395949, 12.52428291510489977, -59.39295307432605853 ) ) ;
#27613=CARTESIAN_POINT ( 'NONE',  ( -3.771071394011080269, 19.25846386140493394, -60.59295307432606847 ) ) ;
#27615=CARTESIAN_POINT ( 'NONE',  ( -3.965139115708213868, 15.65104167704456906, -57.15704692567387468 ) ) ;
#27626=CARTESIAN_POINT ( 'NONE',  ( 1.887862790868997109, 13.79486065368817194, -48.89999999999997016 ) ) ;
#27634=CARTESIAN_POINT ( 'NONE',  ( 4.342430937695320736, 16.96683151040971538, -70.94295307432606990 ) ) ;
#27647=CARTESIAN_POINT ( 'NONE',  ( 3.705139346311793869, 15.61213720913094960, -42.59999999999996589 ) ) ;
#27652=CARTESIAN_POINT ( 'NONE',  ( -4.318543150850367773, 18.18399003996480801, -31.94999999999994955 ) ) ;
#27661=CARTESIAN_POINT ( 'NONE',  ( 0.6839900399647733664, 13.18145684914961357, -52.04999999999997584 ) ) ;
#27663=CARTESIAN_POINT ( 'NONE',  ( -2.439449611014227859, 22.60758118029364283, -45.90704692567387468 ) ) ;
#27664=CARTESIAN_POINT ( 'NONE',  ( 4.206979645153768210, 13.29302035484617406, -39.74999999999996447 ) ) ;
#27668=CARTESIAN_POINT ( 'NONE',  ( -2.940415233664778860, 14.55958476633523802, -73.49999999999997158 ) ) ;
#27679=CARTESIAN_POINT ( 'NONE',  ( -0.7798958854283041253, 23.40020640687986386, -40.05704692567387326 ) ) ;
#27682=CARTESIAN_POINT ( 'NONE',  ( 5.565992480072003978, 18.52860470043125574, -52.79295307432607132 ) ) ;
#27699=CARTESIAN_POINT ( 'NONE',  ( 5.041649132594343996, 14.93115145952162415, -27.59999999999996589 ) ) ;
#27702=CARTESIAN_POINT ( 'NONE',  ( 4.294655364005415699, 16.66518840966061887, -40.95704692567387184 ) ) ;
#27703=CARTESIAN_POINT ( 'NONE',  ( 1.887862790868997109, 13.79486065368817194, -30.89999999999996305 ) ) ;
#27704=CARTESIAN_POINT ( 'NONE',  ( 4.318543150850367773, 16.81600996003516357, -63.44999999999996732 ) ) ;
#27714=CARTESIAN_POINT ( 'NONE',  ( -3.043106805520194413, 14.66227633819065623, -27.00704692567387610 ) ) ;
#27715=CARTESIAN_POINT ( 'NONE',  ( -5.876318620034919782, 18.43071743580290089, -67.94999999999996021 ) ) ;
#27729=CARTESIAN_POINT ( 'NONE',  ( -2.439449611014227859, 22.60758118029364283, -60.90704692567388179 ) ) ;
#27733=CARTESIAN_POINT ( 'NONE',  ( -2.701047200102606016, 12.19889638921340413, -31.34999999999996945 ) ) ;
#27734=ORIENTED_EDGE ( 'NONE', *, *, #19680, .F. ) ;
#27749=CARTESIAN_POINT ( 'NONE',  ( 4.001075405444606048, 21.50107540544455276, -53.99999999999996447 ) ) ;
#27754=CARTESIAN_POINT ( 'NONE',  ( -4.129897239856814117, 16.99292663369196177, -72.30704692567387326 ) ) ;
#27755=CARTESIAN_POINT ( 'NONE',  ( 2.940415233664778416, 20.44041523366473712, -53.99999999999996447 ) ) ;
#27761=CARTESIAN_POINT ( 'NONE',  ( 1.985016409143818272, 21.39581405818570303, -71.84999999999998010 ) ) ;
#27767=CARTESIAN_POINT ( 'NONE',  ( 2.017261720333081598, 13.86079270138745834, -38.39295307432605142 ) ) ;
#27770=CARTESIAN_POINT ( 'NONE',  ( -1.848958322955462474, 13.53486088429179546, -50.84295307432606137 ) ) ;
#27787=CARTESIAN_POINT ( 'NONE',  ( -5.301103610786608300, 14.79895279989743706, -55.64999999999994174 ) ) ;
#27808=CARTESIAN_POINT ( 'NONE',  ( 2.698247469942395949, 12.52428291510489977, -44.39295307432605853 ) ) ;
#27818=CARTESIAN_POINT ( 'NONE',  ( -1.848958322955462474, 13.53486088429179546, -62.84295307432604716 ) ) ;
#27831=CARTESIAN_POINT ( 'NONE',  ( 0.6505131845895220088, 21.60717860451803674, -47.69999999999996732 ) ) ;
#27842=CARTESIAN_POINT ( 'NONE',  ( -4.084459969179292216, 16.70604699712905372, -69.29295307432606421 ) ) ;
#27853=CARTESIAN_POINT ( 'NONE',  ( -0.6505131845895224529, 13.39282139548194195, -34.19999999999996732 ) ) ;
#27857=CARTESIAN_POINT ( 'NONE',  ( -1.887862790868997553, 21.20513934631180319, -38.39999999999997016 ) ) ;
#27866=CARTESIAN_POINT ( 'NONE',  ( -1.985016409143819605, 13.60418594181426855, -58.34999999999995879 ) ) ;
#27868=CARTESIAN_POINT ( 'NONE',  ( -5.370428668309080500, 14.93501088608579153, -48.15704692567388179 ) ) ;
#27869=CARTESIAN_POINT ( 'NONE',  ( -4.206979645153769098, 21.70697964515380107, -38.24999999999996447 ) ) ;
#27872=CARTESIAN_POINT ( 'NONE',  ( -3.771071394011080269, 19.25846386140493394, -30.59295307432605782 ) ) ;
#27883=CARTESIAN_POINT ( 'NONE',  ( 2.837105286290961370, 22.73177855326409613, -31.35704692567387042 ) ) ;
#27889=CARTESIAN_POINT ( 'NONE',  ( 5.565992480072003978, 18.52860470043125574, -49.79295307432606421 ) ) ;
#27908=CARTESIAN_POINT ( 'NONE',  ( -0.9307174358028533767, 23.37631862003491889, -26.54999999999996163 ) ) ;
#27912=CARTESIAN_POINT ( 'NONE',  ( -1.758463861404912842, 21.27107139401109137, -42.90704692567387468 ) ) ;
#27913=CARTESIAN_POINT ( 'NONE',  ( 2.940415233664778416, 20.44041523366473712, -38.99999999999996447 ) ) ;
#27914=CARTESIAN_POINT ( 'NONE',  ( -3.705139346311794313, 19.38786279086902198, -62.09999999999996589 ) ) ;
#27923=CARTESIAN_POINT ( 'NONE',  ( -5.611429750749524992, 16.75827493613162034, -72.30704692567387326 ) ) ;
#27924=CARTESIAN_POINT ( 'NONE',  ( 2.568848540478311460, 12.45835086740561692, -60.89999999999997016 ) ) ;
#27936=CARTESIAN_POINT ( 'NONE',  ( -4.099003336600151925, 21.81495595370741469, -60.75704692567388321 ) ) ;
#27941=CARTESIAN_POINT ( 'NONE',  ( 2.568848540478311460, 12.45835086740561692, -30.89999999999996305 ) ) ;
#27956=CARTESIAN_POINT ( 'NONE',  ( 0.8851648821498760977, 23.08871111541074228, -53.69999999999996732 ) ) ;
#27960=CARTESIAN_POINT ( 'NONE',  ( 4.129897239856814117, 18.00707336630801336, -70.80704692567387326 ) ) ;
#27961=CARTESIAN_POINT ( 'NONE',  ( -3.091735541773221296, 20.59173554177323950, -53.24999999999996447 ) ) ;
#27968=CARTESIAN_POINT ( 'NONE',  ( 0.6505131845895220088, 21.60717860451803674, -71.69999999999997442 ) ) ;
#27972=CARTESIAN_POINT ( 'NONE',  ( 1.848958322955461808, 21.46513911570817612, -40.34295307432606137 ) ) ;
#27975=CARTESIAN_POINT ( 'NONE',  ( -3.771071394011080269, 19.25846386140493394, -54.59295307432605426 ) ) ;
#27992=CARTESIAN_POINT ( 'NONE',  ( 5.588711115410763597, 18.38516488214980882, -57.29999999999996874 ) ) ;
#28003=EDGE_CURVE ( 'NONE', #21597, #3983, #12259, .T. ) ;
#28016=CARTESIAN_POINT ( 'NONE',  ( 5.231778553264135212, 20.33710528629089254, -43.64295307432605853 ) ) ;
#28024=CARTESIAN_POINT ( 'NONE',  ( -3.826489000663265472, 15.37892550466785480, -66.14295307432605853 ) ) ;
#28036=CARTESIAN_POINT ( 'NONE',  ( 1.887862790868997109, 13.79486065368817194, -42.89999999999996305 ) ) ;
#28061=CARTESIAN_POINT ( 'NONE',  ( -3.091735541773221296, 20.59173554177323950, -38.24999999999996447 ) ) ;
#28067=CARTESIAN_POINT ( 'NONE',  ( -3.705139346311794313, 19.38786279086902198, -38.09999999999996589 ) ) ;
#28076=CARTESIAN_POINT ( 'NONE',  ( 0.6505131845895220088, 21.60717860451803674, -53.69999999999996732 ) ) ;
#28077=CARTESIAN_POINT ( 'NONE',  ( -4.975717084895059372, 20.19824746994243370, -51.60704692567387752 ) ) ;
#28078=CARTESIAN_POINT ( 'NONE',  ( -2.568848540478311904, 22.54164913259435465, -35.39999999999996305 ) ) ;
#28080=CARTESIAN_POINT ( 'NONE',  ( 4.084459969179292216, 18.29395300287091430, -28.79295307432605355 ) ) ;
#28092=CARTESIAN_POINT ( 'NONE',  ( 1.028604700431328567, 23.06599248007198355, -25.20704692567387539 ) ) ;
#28097=CARTESIAN_POINT ( 'NONE',  ( 5.565992480072003978, 18.52860470043125574, -55.79295307432606421 ) ) ;
#28115=CARTESIAN_POINT ( 'NONE',  ( -2.698247469942396837, 22.47571708489507358, -75.89295307432605853 ) ) ;
#28119=CARTESIAN_POINT ( 'NONE',  ( -3.965139115708213868, 15.65104167704456906, -42.15704692567387468 ) ) ;
#28120=CARTESIAN_POINT ( 'NONE',  ( 1.985016409143818272, 21.39581405818570303, -35.84999999999996589 ) ) ;
#28121=CARTESIAN_POINT ( 'NONE',  ( -2.940415233664778860, 14.55958476633523802, -61.49999999999997158 ) ) ;
#28132=CARTESIAN_POINT ( 'NONE',  ( 4.294655364005415699, 16.66518840966061887, -25.95704692567387184 ) ) ;
#28133=CARTESIAN_POINT ( 'NONE',  ( -4.206979645153769098, 21.70697964515380107, -65.24999999999995737 ) ) ;
#28144=CARTESIAN_POINT ( 'NONE',  ( -4.103766977300021601, 13.60161616641083704, -69.00704692567386189 ) ) ;
#28147=CARTESIAN_POINT ( 'NONE',  ( 5.041649132594343996, 14.93115145952162415, -33.59999999999996589 ) ) ;
#28167=CARTESIAN_POINT ( 'NONE',  ( -4.206979645153768210, 21.70697964515380107, -53.24999999999996447 ) ) ;
#28171=CARTESIAN_POINT ( 'NONE',  ( -2.940415233664778860, 14.55958476633523802, -28.49999999999996447 ) ) ;
#28172=CARTESIAN_POINT ( 'NONE',  ( 4.107178604518054499, 18.15051318458946383, -57.29999999999996874 ) ) ;
#28178=CARTESIAN_POINT ( 'NONE',  ( -0.6505131845895224529, 13.39282139548194195, -73.19999999999997442 ) ) ;
#28182=CARTESIAN_POINT ( 'NONE',  ( -0.5070733663080690956, 13.37010276014318144, -38.69295307432606279 ) ) ;
#28185=CARTESIAN_POINT ( 'NONE',  ( -3.199711850326840246, 20.48375923321962233, -57.74295307432607416 ) ) ;
#28202=CARTESIAN_POINT ( 'NONE',  ( -2.568848540478311904, 22.54164913259435465, -53.39999999999997016 ) ) ;
#28223=CARTESIAN_POINT ( 'NONE',  ( -1.081538986177402961, 23.35243083318996327, -43.04295307432605711 ) ) ;
#28232=CARTESIAN_POINT ( 'NONE',  ( 3.199711850326839357, 14.51624076678035635, -65.24295307432606705 ) ) ;
#28245=CARTESIAN_POINT ( 'NONE',  ( -0.6505131845895224529, 13.39282139548194195, -43.19999999999996732 ) ) ;
#28273=CARTESIAN_POINT ( 'NONE',  ( -0.6839900399647738105, 21.81854315085035623, -32.54999999999996163 ) ) ;
#28277=CARTESIAN_POINT ( 'NONE',  ( 3.895814058185739448, 19.48501640914375344, -36.14999999999994884 ) ) ;
#28284=CARTESIAN_POINT ( 'NONE',  ( -2.940415233664778860, 14.55958476633523802, -55.49999999999996447 ) ) ;
#28287=CARTESIAN_POINT ( 'NONE',  ( -5.852430833189966819, 18.58153898617744915, -48.45704692567387895 ) ) ;
#28288=CARTESIAN_POINT ( 'NONE',  ( 4.206979645153768210, 13.29302035484617406, -33.74999999999996447 ) ) ;
#28290=CARTESIAN_POINT ( 'NONE',  ( 3.705139346311793869, 15.61213720913094960, -69.59999999999996589 ) ) ;
#28301=CARTESIAN_POINT ( 'NONE',  ( 4.975717084895059372, 14.80175253005754143, -29.10704692567387752 ) ) ;
#28305=CARTESIAN_POINT ( 'NONE',  ( 5.900206406879871857, 16.72010411457162604, -43.94295307432605568 ) ) ;
#28321=( NAMED_UNIT ( * ) SI_UNIT ( $, .STERADIAN. ) SOLID_ANGLE_UNIT ( ) );
#28322=CARTESIAN_POINT ( 'NONE',  ( -0.7417250638684240727, 11.88857024925047057, -71.69295307432605568 ) ) ;
#28328=CARTESIAN_POINT ( 'NONE',  ( -0.6505131845895224529, 13.39282139548194195, -37.19999999999996732 ) ) ;
#28329=CARTESIAN_POINT ( 'NONE',  ( -4.318543150850367773, 18.18399003996480801, -64.94999999999996021 ) ) ;
#28340=CARTESIAN_POINT ( 'NONE',  ( 4.103766977300021601, 21.39838383358913987, -73.50704692567386189 ) ) ;
#28341=CARTESIAN_POINT ( 'NONE',  ( -4.206979645153769098, 21.70697964515380107, -62.24999999999996447 ) ) ;
#28353=CARTESIAN_POINT ( 'NONE',  ( -5.611429750749524992, 16.75827493613162034, -54.30704692567388037 ) ) ;
#28356=CARTESIAN_POINT ( 'NONE',  ( -2.564989113914250662, 12.12957133169093282, -74.84295307432606137 ) ) ;
#28372=CARTESIAN_POINT ( 'NONE',  ( -5.876318620034919782, 18.43071743580290089, -55.94999999999997442 ) ) ;
#28376=CARTESIAN_POINT ( 'NONE',  ( -2.121074495332175847, 13.67351099933674341, -68.85704692567387042 ) ) ;
#28377=CARTESIAN_POINT ( 'NONE',  ( -3.091735541773221296, 20.59173554177323950, -59.24999999999997158 ) ) ;
#28383=CARTESIAN_POINT ( 'NONE',  ( 3.895814058185739448, 19.48501640914375344, -72.14999999999996305 ) ) ;
#28387=CARTESIAN_POINT ( 'NONE',  ( -4.129897239856814117, 16.99292663369196177, -54.30704692567388037 ) ) ;
#28390=CARTESIAN_POINT ( 'NONE',  ( -1.887862790868997553, 21.20513934631180319, -74.39999999999996305 ) ) ;
#28393=CARTESIAN_POINT ( 'NONE',  ( 1.848958322955461808, 21.46513911570817612, -49.34295307432604716 ) ) ;
#28408=CARTESIAN_POINT ( 'NONE',  ( 2.701047200102605572, 22.80110361078655856, -59.84999999999996589 ) ) ;
#28429=CARTESIAN_POINT ( 'NONE',  ( 4.314955953707388936, 13.40099666339979123, -41.24295307432605284 ) ) ;
#28437=CARTESIAN_POINT ( 'NONE',  ( -3.199711850326840246, 20.48375923321962233, -54.74295307432605995 ) ) ;
#28452=CARTESIAN_POINT ( 'NONE',  ( 0.6505131845895220088, 21.60717860451803674, -44.69999999999996021 ) ) ;
#28477=CARTESIAN_POINT ( 'NONE',  ( 3.895814058185739892, 19.48501640914376054, -30.14999999999997016 ) ) ;
#28482=CARTESIAN_POINT ( 'NONE',  ( -3.639207298612509689, 19.51726172033310647, -69.60704692567387042 ) ) ;
#28489=CARTESIAN_POINT ( 'NONE',  ( -0.6839900399647736995, 21.81854315085035623, -56.54999999999996874 ) ) ;
#28492=CARTESIAN_POINT ( 'NONE',  ( -1.028604700431329233, 11.93400751992799513, -44.70704692567387184 ) ) ;
#28493=CARTESIAN_POINT ( 'NONE',  ( -3.895814058185739448, 15.51498359085620571, -73.64999999999993463 ) ) ;
#28506=CARTESIAN_POINT ( 'NONE',  ( 4.103766977300021601, 21.39838383358913987, -28.50704692567387610 ) ) ;
#28513=CARTESIAN_POINT ( 'NONE',  ( 5.231778553264135212, 20.33710528629089254, -40.64295307432606563 ) ) ;
#28531=CARTESIAN_POINT ( 'NONE',  ( -0.7417250638684240727, 11.88857024925047057, -65.69295307432605568 ) ) ;
#28536=CARTESIAN_POINT ( 'NONE',  ( -1.985016409143819605, 13.60418594181426855, -37.34999999999994458 ) ) ;
#28537=CARTESIAN_POINT ( 'NONE',  ( 0.6505131845895220088, 21.60717860451803674, -53.69999999999996732 ) ) ;
#28549=CARTESIAN_POINT ( 'NONE',  ( -3.043106805520194413, 14.66227633819065623, -24.00704692567387610 ) ) ;
#28550=CARTESIAN_POINT ( 'NONE',  ( -0.8851648821498765418, 11.91128888458923285, -52.19999999999996732 ) ) ;
#28561=CARTESIAN_POINT ( 'NONE',  ( 5.611429750749524992, 18.24172506386835479, -52.80704692567387326 ) ) ;
#28565=CARTESIAN_POINT ( 'NONE',  ( -3.898383833589191827, 13.39623302270000771, -68.99295307432605284 ) ) ;
#28583=CARTESIAN_POINT ( 'NONE',  ( 5.588711115410763597, 18.38516488214980882, -39.29999999999996874 ) ) ;
#28587=CARTESIAN_POINT ( 'NONE',  ( -4.294655364005415699, 18.33481159033935626, -66.45704692567387895 ) ) ;
#28588=CARTESIAN_POINT ( 'NONE',  ( 0.6839900399647732554, 13.18145684914961357, -55.04999999999996163 ) ) ;
#28596=CARTESIAN_POINT ( 'NONE',  ( 3.091735541773220852, 14.40826445822673563, -66.74999999999997158 ) ) ;
#28598=CARTESIAN_POINT ( 'NONE',  ( -2.983759233219601903, 20.69971185032686023, -57.75704692567386900 ) ) ;
#28601=CARTESIAN_POINT ( 'NONE',  ( -2.017261720333081598, 21.13920729861251857, -27.89295307432605853 ) ) ;
#28604=CARTESIAN_POINT ( 'NONE',  ( -1.848958322955462474, 13.53486088429179546, -41.84295307432606137 ) ) ;
#28619=CARTESIAN_POINT ( 'NONE',  ( 4.206979645153767322, 13.29302035484617051, -45.74999999999995737 ) ) ;
#28640=CARTESIAN_POINT ( 'NONE',  ( -3.895814058185739448, 15.51498359085620571, -46.64999999999994884 ) ) ;
#28641=CARTESIAN_POINT ( 'NONE',  ( -5.107581180293630396, 19.93944961101426827, -42.59295307432605426 ) ) ;
#28649=CARTESIAN_POINT ( 'NONE',  ( -3.771071394011080269, 19.25846386140493394, -54.59295307432605426 ) ) ;
#28660=CARTESIAN_POINT ( 'NONE',  ( -2.940415233664778860, 14.55958476633523802, -37.49999999999996447 ) ) ;
#28686=CARTESIAN_POINT ( 'NONE',  ( 1.985016409143818272, 21.39581405818570659, -26.84999999999996234 ) ) ;
#28689=CARTESIAN_POINT ( 'NONE',  ( 4.314955953707388936, 13.40099666339979123, -32.24295307432605284 ) ) ;
#28690=CARTESIAN_POINT ( 'NONE',  ( -1.887862790868997553, 21.20513934631180319, -29.39999999999996660 ) ) ;
#28697=CARTESIAN_POINT ( 'NONE',  ( -0.6505131845895224529, 13.39282139548194195, -43.19999999999996732 ) ) ;
#28700=CARTESIAN_POINT ( 'NONE',  ( 5.611429750749524992, 18.24172506386835479, -37.80704692567387326 ) ) ;
#28702=CARTESIAN_POINT ( 'NONE',  ( -3.091735541773221296, 20.59173554177323950, -65.24999999999995737 ) ) ;
#28712=CARTESIAN_POINT ( 'NONE',  ( -5.852430833189966819, 18.58153898617744915, -30.45704692567387184 ) ) ;
#28718=CARTESIAN_POINT ( 'NONE',  ( -2.698247469942396837, 22.47571708489507358, -45.89295307432605853 ) ) ;
#28733=CARTESIAN_POINT ( 'NONE',  ( 2.698247469942395949, 12.52428291510489977, -62.39295307432605853 ) ) ;
#28738=CARTESIAN_POINT ( 'NONE',  ( -3.895814058185739448, 15.51498359085620571, -25.64999999999996305 ) ) ;
#28739=CARTESIAN_POINT ( 'NONE',  ( -4.318543150850367773, 18.18399003996480801, -52.94999999999994600 ) ) ;
#28751=CARTESIAN_POINT ( 'NONE',  ( -2.837105286290963146, 12.26822144673588255, -65.85704692567387042 ) ) ;
#28752=CARTESIAN_POINT ( 'NONE',  ( 5.588711115410763597, 18.38516488214980882, -54.29999999999996874 ) ) ;
#28763=CARTESIAN_POINT ( 'NONE',  ( 5.852430833189966819, 16.41846101382252243, -58.95704692567386473 ) ) ;
#28769=CARTESIAN_POINT ( 'NONE',  ( 4.314955953707388936, 13.40099666339979123, -68.24295307432605284 ) ) ;
#28785=CARTESIAN_POINT ( 'NONE',  ( 4.001075405444606048, 21.50107540544455276, -38.99999999999996447 ) ) ;
#28789=CARTESIAN_POINT ( 'NONE',  ( -2.983759233219601903, 20.69971185032686023, -66.75704692567384768 ) ) ;
#28790=CARTESIAN_POINT ( 'NONE',  ( -4.318543150850366885, 18.18399003996480801, -49.94999999999995310 ) ) ;
#28801=CARTESIAN_POINT ( 'NONE',  ( 4.318543150850367773, 16.81600996003516357, -66.44999999999997442 ) ) ;
#28804=CARTESIAN_POINT ( 'NONE',  ( -3.043106805520194413, 14.66227633819065623, -51.00704692567387610 ) ) ;
#28807=CARTESIAN_POINT ( 'NONE',  ( -1.985016409143819605, 13.60418594181426855, -73.34999999999996589 ) ) ;
#28810=CARTESIAN_POINT ( 'NONE',  ( -4.342430937695320736, 18.03316848959025620, -45.44295307432605568 ) ) ;
#28824=CARTESIAN_POINT ( 'NONE',  ( 5.301103610786608300, 20.20104720010253985, -45.14999999999994884 ) ) ;
#28839=CARTESIAN_POINT ( 'NONE',  ( -0.9307174358028533767, 23.37631862003491889, -68.54999999999998295 ) ) ;
#28845=CARTESIAN_POINT ( 'NONE',  ( -4.107178604518053611, 16.84948681541050775, -46.79999999999996874 ) ) ;
#28856=CARTESIAN_POINT ( 'NONE',  ( -4.342430937695320736, 18.03316848959025620, -54.44295307432606990 ) ) ;
#28874=CARTESIAN_POINT ( 'NONE',  ( -4.107178604518053611, 16.84948681541050775, -37.79999999999996874 ) ) ;
#28900=CARTESIAN_POINT ( 'NONE',  ( -4.129897239856814117, 16.99292663369196177, -33.30704692567387326 ) ) ;
#28901=CARTESIAN_POINT ( 'NONE',  ( -0.6505131845895224529, 13.39282139548194195, -28.19999999999996732 ) ) ;
#28904=CARTESIAN_POINT ( 'NONE',  ( -5.107581180293630396, 19.93944961101426827, -30.59295307432605782 ) ) ;
#28905=CARTESIAN_POINT ( 'NONE',  ( -3.895814058185739448, 15.51498359085620571, -25.64999999999996305 ) ) ;
#28912=CARTESIAN_POINT ( 'NONE',  ( -3.895814058185739448, 15.51498359085620571, -49.64999999999995595 ) ) ;
#28915=CARTESIAN_POINT ( 'NONE',  ( 5.370428668309080500, 20.06498911391418360, -40.65704692567387468 ) ) ;
#28917=CARTESIAN_POINT ( 'NONE',  ( -4.318543150850367773, 18.18399003996480801, -64.94999999999996021 ) ) ;
#28930=CARTESIAN_POINT ( 'NONE',  ( -2.564989113914250662, 12.12957133169093282, -38.84295307432606137 ) ) ;
#28944=CARTESIAN_POINT ( 'NONE',  ( 5.231778553264135212, 20.33710528629089254, -67.64295307432605853 ) ) ;
#28951=CARTESIAN_POINT ( 'NONE',  ( -1.985016409143819605, 13.60418594181426855, -52.34999999999994458 ) ) ;
#28962=CARTESIAN_POINT ( 'NONE',  ( 4.103766977300021601, 21.39838383358913987, -61.50704692567389031 ) ) ;
#28963=CARTESIAN_POINT ( 'NONE',  ( -5.041649132594344884, 20.06884854047834921, -56.09999999999996589 ) ) ;
#28974=CARTESIAN_POINT ( 'NONE',  ( -5.852430833189966819, 18.58153898617744915, -51.45704692567387895 ) ) ;
#28979=CARTESIAN_POINT ( 'NONE',  ( 5.565992480072003978, 18.52860470043125574, -67.79295307432606421 ) ) ;
#28996=CARTESIAN_POINT ( 'NONE',  ( 2.568848540478311460, 12.45835086740561692, -42.89999999999996305 ) ) ;
#29000=CARTESIAN_POINT ( 'NONE',  ( 2.983759233219601459, 14.30028814967311668, -59.25704692567388321 ) ) ;
#29001=CARTESIAN_POINT ( 'NONE',  ( -3.091735541773221296, 20.59173554177323950, -50.24999999999997158 ) ) ;
#29012=CARTESIAN_POINT ( 'NONE',  ( -2.940415233664778860, 14.55958476633523802, -61.49999999999997158 ) ) ;
#29014=CARTESIAN_POINT ( 'NONE',  ( 4.129897239856814117, 18.00707336630801336, -49.80704692567388037 ) ) ;
#29019=CARTESIAN_POINT ( 'NONE',  ( -0.8348115903393239501, 21.79465536400541126, -43.04295307432605711 ) ) ;
#29033=CARTESIAN_POINT ( 'NONE',  ( 2.568848540478311460, 12.45835086740561692, -45.89999999999997016 ) ) ;
#29049=CARTESIAN_POINT ( 'NONE',  ( 2.701047200102605572, 22.80110361078655856, -74.84999999999993747 ) ) ;
#29055=CARTESIAN_POINT ( 'NONE',  ( -3.705139346311794313, 19.38786279086902198, -47.09999999999996589 ) ) ;
#29065=CARTESIAN_POINT ( 'NONE',  ( -4.084459969179292216, 16.70604699712905372, -51.29295307432606421 ) ) ;
#29078=CARTESIAN_POINT ( 'NONE',  ( 3.895814058185739448, 19.48501640914375344, -36.14999999999994884 ) ) ;
#29103=CARTESIAN_POINT ( 'NONE',  ( 0.7939530028709752552, 21.58445996917927445, -34.20704692567387184 ) ) ;
#29104=CARTESIAN_POINT ( 'NONE',  ( -4.107178604518053611, 16.84948681541050775, -31.79999999999996874 ) ) ;
#29107=CARTESIAN_POINT ( 'NONE',  ( 5.231778553264135212, 20.33710528629089254, -34.64295307432605142 ) ) ;
#29108=CARTESIAN_POINT ( 'NONE',  ( 2.121074495332174958, 21.32648900066323350, -70.35704692567388463 ) ) ;
#29115=CARTESIAN_POINT ( 'NONE',  ( -1.887862790868997553, 21.20513934631180319, -47.39999999999997016 ) ) ;
#29117=CARTESIAN_POINT ( 'NONE',  ( 4.103766977300021601, 21.39838383358913987, -40.50704692567387610 ) ) ;
#29118=CARTESIAN_POINT ( 'NONE',  ( -4.206979645153769098, 21.70697964515380107, -26.24999999999996803 ) ) ;
#29119=CARTESIAN_POINT ( 'NONE',  ( -3.705139346311794313, 19.38786279086902198, -68.09999999999996589 ) ) ;
#29133=CARTESIAN_POINT ( 'NONE',  ( 3.898383833589191383, 21.60376697729997275, -37.49295307432604574 ) ) ;
#29151=CARTESIAN_POINT ( 'NONE',  ( -3.091735541773221296, 20.59173554177323950, -50.24999999999997158 ) ) ;
#29162=CARTESIAN_POINT ( 'NONE',  ( 2.837105286290961370, 22.73177855326409613, -70.35704692567388463 ) ) ;
#29163=CARTESIAN_POINT ( 'NONE',  ( -2.701047200102606460, 12.19889638921340591, -52.34999999999995879 ) ) ;
#29175=CARTESIAN_POINT ( 'NONE',  ( 4.975717084895059372, 14.80175253005754143, -50.10704692567387752 ) ) ;
#29178=CARTESIAN_POINT ( 'NONE',  ( -0.7417250638684240727, 11.88857024925047057, -71.69295307432605568 ) ) ;
#29194=CARTESIAN_POINT ( 'NONE',  ( -2.568848540478311904, 22.54164913259435465, -38.39999999999997016 ) ) ;
#29197=CARTESIAN_POINT ( 'NONE',  ( -4.129897239856814117, 16.99292663369196177, -63.30704692567387326 ) ) ;
#29199=CARTESIAN_POINT ( 'NONE',  ( 3.705139346311793869, 15.61213720913094960, -45.59999999999996589 ) ) ;
#29210=CARTESIAN_POINT ( 'NONE',  ( 4.318543150850367773, 16.81600996003516357, -60.44999999999997442 ) ) ;
#29212=CARTESIAN_POINT ( 'NONE',  ( -4.294655364005415699, 18.33481159033935626, -48.45704692567387895 ) ) ;
#29217=CARTESIAN_POINT ( 'NONE',  ( -0.8348115903393239501, 21.79465536400541126, -31.04295307432605355 ) ) ;
#29229=CARTESIAN_POINT ( 'NONE',  ( -4.001075405444606936, 13.49892459455542060, -49.49999999999996447 ) ) ;
#29248=CARTESIAN_POINT ( 'NONE',  ( -4.206979645153768210, 21.70697964515380107, -74.24999999999997158 ) ) ;
#29253=CARTESIAN_POINT ( 'NONE',  ( -2.940415233664778860, 14.55958476633523802, -43.49999999999997158 ) ) ;
#29266=CARTESIAN_POINT ( 'NONE',  ( -4.342430937695320736, 18.03316848959025620, -51.44295307432605568 ) ) ;
#29283=CARTESIAN_POINT ( 'NONE',  ( 3.705139346311793869, 15.61213720913094960, -33.59999999999996589 ) ) ;
#29309=CARTESIAN_POINT ( 'NONE',  ( 2.121074495332174958, 21.32648900066323350, -31.35704692567387042 ) ) ;
#29314=CARTESIAN_POINT ( 'NONE',  ( 1.081538986177402295, 11.64756916681001186, -38.54295307432605000 ) ) ;
#29315=CARTESIAN_POINT ( 'NONE',  ( -1.758463861404912842, 21.27107139401109137, -72.90704692567388179 ) ) ;
#29324=CARTESIAN_POINT ( 'NONE',  ( 4.107178604518054499, 18.15051318458946383, -48.29999999999996874 ) ) ;
#29327=CARTESIAN_POINT ( 'NONE',  ( -5.611429750749524992, 16.75827493613162034, -39.30704692567388037 ) ) ;
#29328=CARTESIAN_POINT ( 'NONE',  ( 5.041649132594343996, 14.93115145952162415, -27.59999999999996589 ) ) ;
#29329=CARTESIAN_POINT ( 'NONE',  ( 3.895814058185739448, 19.48501640914375344, -69.14999999999994884 ) ) ;
#29342=CARTESIAN_POINT ( 'NONE',  ( 0.7417250638684235176, 23.11142975074950101, -28.19295307432605568 ) ) ;
#29363=CARTESIAN_POINT ( 'NONE',  ( 0.6839900399647733664, 13.18145684914961357, -28.04999999999995453 ) ) ;
#29364=CARTESIAN_POINT ( 'NONE',  ( 1.887862790868997109, 13.79486065368817194, -51.89999999999997016 ) ) ;
#29374=CARTESIAN_POINT ( 'NONE',  ( -5.852430833189966819, 18.58153898617744915, -69.45704692567387895 ) ) ;
#29375=CARTESIAN_POINT ( 'NONE',  ( -4.001075405444606936, 13.49892459455542060, -55.49999999999996447 ) ) ;
#29389=CARTESIAN_POINT ( 'NONE',  ( 5.611429750749524992, 18.24172506386835479, -49.80704692567388037 ) ) ;
#29393=CARTESIAN_POINT ( 'NONE',  ( 3.898383833589191383, 21.60376697729997275, -64.49295307432606705 ) ) ;
#29410=CARTESIAN_POINT ( 'NONE',  ( 4.206979645153767322, 13.29302035484617051, -45.74999999999995737 ) ) ;
#29413=CARTESIAN_POINT ( 'NONE',  ( -4.294655364005415699, 18.33481159033935626, -48.45704692567387895 ) ) ;
#29414=CARTESIAN_POINT ( 'NONE',  ( 3.895814058185739892, 19.48501640914376054, -45.14999999999996305 ) ) ;
#29423=CARTESIAN_POINT ( 'NONE',  ( -3.091735541773221296, 20.59173554177323950, -62.24999999999995737 ) ) ;
#29426=CARTESIAN_POINT ( 'NONE',  ( -2.121074495332175847, 13.67351099933674341, -47.85704692567386331 ) ) ;
#29431=CARTESIAN_POINT ( 'NONE',  ( -1.848958322955462474, 13.53486088429179546, -35.84295307432606137 ) ) ;
#29438=CARTESIAN_POINT ( 'NONE',  ( -4.103766977300021601, 13.60161616641083704, -72.00704692567386189 ) ) ;
#29445=CARTESIAN_POINT ( 'NONE',  ( 5.876318620034919782, 16.56928256419707068, -51.44999999999997442 ) ) ;
#29463=CARTESIAN_POINT ( 'NONE',  ( -5.041649132594344884, 20.06884854047834921, -68.09999999999996589 ) ) ;
#29468=CARTESIAN_POINT ( 'NONE',  ( -3.895814058185739448, 15.51498359085620571, -40.64999999999994174 ) ) ;
#29469=CARTESIAN_POINT ( 'NONE',  ( -3.895814058185739892, 15.51498359085620748, -73.64999999999994884 ) ) ;
#29481=CARTESIAN_POINT ( 'NONE',  ( 3.771071394011080269, 15.74153613859503764, -44.09295307432605426 ) ) ;
#29486=CARTESIAN_POINT ( 'NONE',  ( -0.5070733663080690956, 13.37010276014318144, -59.69295307432605568 ) ) ;
#29498=CARTESIAN_POINT ( 'NONE',  ( 1.985016409143818272, 21.39581405818570303, -32.84999999999996589 ) ) ;
#29507=CARTESIAN_POINT ( 'NONE',  ( 0.7798958854283032371, 11.59979359312010772, -26.55704692567386971 ) ) ;
#29528=CARTESIAN_POINT ( 'NONE',  ( 1.758463861404912620, 13.72892860598888731, -38.40704692567386758 ) ) ;
#29533=CARTESIAN_POINT ( 'NONE',  ( 5.565992480072003978, 18.52860470043125574, -31.79295307432605355 ) ) ;
#29535=CARTESIAN_POINT ( 'NONE',  ( -3.965139115708213868, 15.65104167704456906, -60.15704692567387468 ) ) ;
#29543=CARTESIAN_POINT ( 'NONE',  ( -1.985016409143819605, 13.60418594181426855, -46.34999999999997300 ) ) ;
#29546=CARTESIAN_POINT ( 'NONE',  ( -0.7798958854283041253, 23.40020640687986386, -34.05704692567386616 ) ) ;
#29548=CARTESIAN_POINT ( 'NONE',  ( 3.091735541773220852, 14.40826445822673563, -63.74999999999997868 ) ) ;
#29560=CARTESIAN_POINT ( 'NONE',  ( -4.206979645153769098, 21.70697964515380107, -29.24999999999996447 ) ) ;
#29562=CARTESIAN_POINT ( 'NONE',  ( -5.231778553264134324, 14.66289471370907727, -36.14295307432605142 ) ) ;
#29581=CARTESIAN_POINT ( 'NONE',  ( 4.318543150850367773, 16.81600996003516357, -42.44999999999996732 ) ) ;
#29589=CARTESIAN_POINT ( 'NONE',  ( 1.848958322955461808, 21.46513911570817612, -28.34295307432605426 ) ) ;
#29591=CARTESIAN_POINT ( 'NONE',  ( 4.103766977300021601, 21.39838383358913987, -67.50704692567386189 ) ) ;
#29592=CARTESIAN_POINT ( 'NONE',  ( 0.8851648821498760977, 23.08871111541074228, -44.69999999999996021 ) ) ;
#29605=CARTESIAN_POINT ( 'NONE',  ( 2.439449611014226971, 12.39241881970633230, -47.40704692567387468 ) ) ;
#29609=CARTESIAN_POINT ( 'NONE',  ( -5.565992480072003978, 16.47139529956871229, -60.29295307432605000 ) ) ;
#29625=CARTESIAN_POINT ( 'NONE',  ( -5.301103610786608300, 14.79895279989743706, -28.64999999999995950 ) ) ;
#29629=CARTESIAN_POINT ( 'NONE',  ( 3.965139115708213868, 19.34895832295540430, -55.65704692567387468 ) ) ;
#29630=CARTESIAN_POINT ( 'NONE',  ( 3.091735541773220852, 14.40826445822673740, -48.74999999999995737 ) ) ;
#29639=CARTESIAN_POINT ( 'NONE',  ( 3.705139346311793869, 15.61213720913094960, -51.59999999999996589 ) ) ;
#29641=CARTESIAN_POINT ( 'NONE',  ( -3.965139115708213868, 15.65104167704456906, -48.15704692567388179 ) ) ;
#29645=CARTESIAN_POINT ( 'NONE',  ( 0.5070733663080689846, 21.62989723985679902, -37.19295307432606279 ) ) ;
#29651=CARTESIAN_POINT ( 'NONE',  ( 3.639207298612508801, 15.48273827966686866, -26.10704692567387397 ) ) ;
#29657=CARTESIAN_POINT ( 'NONE',  ( 2.701047200102605572, 22.80110361078655856, -41.84999999999995879 ) ) ;
#29677=CARTESIAN_POINT ( 'NONE',  ( -0.9307174358028533767, 23.37631862003491889, -74.54999999999994031 ) ) ;
#29683=CARTESIAN_POINT ( 'NONE',  ( -3.705139346311794313, 19.38786279086902198, -32.09999999999996589 ) ) ;
#29684=CARTESIAN_POINT ( 'NONE',  ( 0.6505131845895220088, 21.60717860451803674, -74.69999999999997442 ) ) ;
#29697=CARTESIAN_POINT ( 'NONE',  ( -3.199711850326840246, 20.48375923321962233, -42.74295307432605284 ) ) ;
#29702=CARTESIAN_POINT ( 'NONE',  ( -0.5070733663080690956, 13.37010276014318144, -68.69295307432605568 ) ) ;
#29713=CARTESIAN_POINT ( 'NONE',  ( 2.940415233664778416, 20.44041523366473712, -26.99999999999996803 ) ) ;
#29721=CARTESIAN_POINT ( 'NONE',  ( 5.041649132594343996, 14.93115145952162415, -63.59999999999995879 ) ) ;
#29735=CARTESIAN_POINT ( 'NONE',  ( -2.564989113914250662, 12.12957133169093282, -62.84295307432604716 ) ) ;
#29739=CARTESIAN_POINT ( 'NONE',  ( -3.965139115708213868, 15.65104167704456906, -33.15704692567386047 ) ) ;
#29743=CARTESIAN_POINT ( 'NONE',  ( -3.199711850326840246, 20.48375923321962233, -75.74295307432603863 ) ) ;
#29745=CARTESIAN_POINT ( 'NONE',  ( -2.983759233219601903, 20.69971185032686023, -66.75704692567384768 ) ) ;
#29754=CARTESIAN_POINT ( 'NONE',  ( -3.895814058185739448, 15.51498359085620571, -40.64999999999994174 ) ) ;
#29757=CARTESIAN_POINT ( 'NONE',  ( -4.975717084895059372, 20.19824746994243370, -27.60704692567387397 ) ) ;
#29759=CARTESIAN_POINT ( 'NONE',  ( -4.107178604518053611, 16.84948681541050775, -52.79999999999996874 ) ) ;
#29772=CARTESIAN_POINT ( 'NONE',  ( -2.698247469942396837, 22.47571708489507358, -33.89295307432605142 ) ) ;
#29791=CARTESIAN_POINT ( 'NONE',  ( -3.895814058185739448, 15.51498359085620571, -43.64999999999996305 ) ) ;
#29800=CARTESIAN_POINT ( 'NONE',  ( -2.940415233664778860, 14.55958476633523802, -73.49999999999997158 ) ) ;
#29802=CARTESIAN_POINT ( 'NONE',  ( 5.370428668309080500, 20.06498911391418360, -52.65704692567388179 ) ) ;
#29803=CARTESIAN_POINT ( 'NONE',  ( 4.206979645153768210, 13.29302035484617406, -48.74999999999995737 ) ) ;
#29819=CARTESIAN_POINT ( 'NONE',  ( -2.439449611014227859, 22.60758118029364283, -45.90704692567387468 ) ) ;
#29823=CARTESIAN_POINT ( 'NONE',  ( -1.081538986177402961, 23.35243083318996327, -64.04295307432605000 ) ) ;
#29838=CARTESIAN_POINT ( 'NONE',  ( -5.876318620034919782, 18.43071743580290089, -31.94999999999994955 ) ) ;
#29841=CARTESIAN_POINT ( 'NONE',  ( -0.7939530028709754772, 13.41554003082070246, -56.70704692567387184 ) ) ;
#29842=CARTESIAN_POINT ( 'NONE',  ( 0.6505131845895220088, 21.60717860451803674, -35.69999999999996732 ) ) ;
#29852=CARTESIAN_POINT ( 'NONE',  ( -0.6505131845895224529, 13.39282139548194195, -52.19999999999996732 ) ) ;
#29855=CARTESIAN_POINT ( 'NONE',  ( 1.758463861404912620, 13.72892860598888731, -32.40704692567386758 ) ) ;
#29859=CARTESIAN_POINT ( 'NONE',  ( 3.199711850326839357, 14.51624076678035635, -32.24295307432605284 ) ) ;
#29866=CARTESIAN_POINT ( 'NONE',  ( -2.983759233219601903, 20.69971185032686023, -24.75704692567387610 ) ) ;
#29873=CARTESIAN_POINT ( 'NONE',  ( 5.588711115410763597, 18.38516488214980882, -42.29999999999996874 ) ) ;
#29890=CARTESIAN_POINT ( 'NONE',  ( -0.8851648821498765418, 11.91128888458923285, -64.19999999999996021 ) ) ;
#29895=CARTESIAN_POINT ( 'NONE',  ( -3.091735541773221296, 20.59173554177323950, -35.24999999999997158 ) ) ;
#29896=CARTESIAN_POINT ( 'NONE',  ( -4.107178604518053611, 16.84948681541050775, -64.79999999999996874 ) ) ;
#29908=CARTESIAN_POINT ( 'NONE',  ( 3.826489000663266360, 19.62107449533211678, -43.64295307432605853 ) ) ;
#29913=CARTESIAN_POINT ( 'NONE',  ( -1.848958322955462474, 13.53486088429179546, -65.84295307432604716 ) ) ;
#29932=CARTESIAN_POINT ( 'NONE',  ( 2.568848540478311460, 12.45835086740561692, -66.89999999999997726 ) ) ;
#29948=CARTESIAN_POINT ( 'NONE',  ( -5.231778553264134324, 14.66289471370907727, -60.14295307432605142 ) ) ;
#29956=CARTESIAN_POINT ( 'NONE',  ( -1.758463861404912842, 21.27107139401109137, -63.90704692567388179 ) ) ;
#29968=CARTESIAN_POINT ( 'NONE',  ( -0.7798958854283041253, 23.40020640687986386, -28.05704692567386971 ) ) ;
#29970=CARTESIAN_POINT ( 'NONE',  ( 2.940415233664778416, 20.44041523366473712, -59.99999999999997158 ) ) ;
#29982=CARTESIAN_POINT ( 'NONE',  ( -2.564989113914250662, 12.12957133169093282, -35.84295307432606137 ) ) ;
#30003=CARTESIAN_POINT ( 'NONE',  ( 2.940415233664778416, 20.44041523366473712, -47.99999999999996447 ) ) ;
#30012=CARTESIAN_POINT ( 'NONE',  ( -1.887862790868997553, 21.20513934631180319, -68.39999999999997726 ) ) ;
#30014=CARTESIAN_POINT ( 'NONE',  ( -4.099003336600151925, 21.81495595370741469, -60.75704692567388321 ) ) ;
#30015=CARTESIAN_POINT ( 'NONE',  ( -2.568848540478311904, 22.54164913259435465, -41.39999999999996305 ) ) ;
#30029=CARTESIAN_POINT ( 'NONE',  ( -2.698247469942396837, 22.47571708489507358, -39.89295307432605853 ) ) ;
#30031=CARTESIAN_POINT ( 'NONE',  ( 2.837105286290961370, 22.73177855326409613, -43.35704692567387752 ) ) ;
#30035=CARTESIAN_POINT ( 'NONE',  ( 5.900206406879871857, 16.72010411457162604, -58.94295307432605568 ) ) ;
#30050=CARTESIAN_POINT ( 'NONE',  ( 2.568848540478311460, 12.45835086740561692, -33.89999999999996305 ) ) ;
#30053=CARTESIAN_POINT ( 'NONE',  ( 0.5331684895902240040, 13.15756906230466328, -56.55704692567387326 ) ) ;
#30054=CARTESIAN_POINT ( 'NONE',  ( -1.887862790868997553, 21.20513934631180319, -74.39999999999996305 ) ) ;
#30062=CARTESIAN_POINT ( 'NONE',  ( 3.895814058185739448, 19.48501640914375344, -54.14999999999997726 ) ) ;
#30064=CARTESIAN_POINT ( 'NONE',  ( -4.129897239856814117, 16.99292663369196177, -39.30704692567388037 ) ) ;
#30069=CARTESIAN_POINT ( 'NONE',  ( 0.5070733663080689846, 21.62989723985679902, -31.19295307432605568 ) ) ;
#30078=CARTESIAN_POINT ( 'NONE',  ( 3.043106805520193525, 20.33772366180932067, -28.50704692567387610 ) ) ;
#30085=CARTESIAN_POINT ( 'NONE',  ( 2.701047200102605572, 22.80110361078655856, -35.84999999999996589 ) ) ;
#30098=CARTESIAN_POINT ( 'NONE',  ( 4.001075405444606048, 21.50107540544455276, -62.99999999999997158 ) ) ;
#30105=CARTESIAN_POINT ( 'NONE',  ( 1.887862790868997109, 13.79486065368817194, -36.89999999999997016 ) ) ;
#30106=CARTESIAN_POINT ( 'NONE',  ( -4.318543150850366885, 18.18399003996480801, -64.94999999999996021 ) ) ;
#30107=CIRCLE ( 'NONE', #38945, 0.7500000000000012212 ) ;
#30119=CARTESIAN_POINT ( 'NONE',  ( 2.017261720333081598, 13.86079270138745834, -41.39295307432605853 ) ) ;
#30124=CARTESIAN_POINT ( 'NONE',  ( 3.199711850326839357, 14.51624076678035635, -62.24295307432607416 ) ) ;
#30134=CARTESIAN_POINT ( 'NONE',  ( -2.940415233664778860, 14.55958476633523802, -28.49999999999996447 ) ) ;
#30142=CARTESIAN_POINT ( 'NONE',  ( 5.588711115410763597, 18.38516488214980882, -69.29999999999996874 ) ) ;
#30161=CARTESIAN_POINT ( 'NONE',  ( 5.107581180293630396, 15.06055038898570686, -53.09295307432605426 ) ) ;
#30171=CARTESIAN_POINT ( 'NONE',  ( -1.848958322955462474, 13.53486088429179546, -71.84295307432606137 ) ) ;
#30173=CARTESIAN_POINT ( 'NONE',  ( -3.965139115708213868, 15.65104167704456906, -66.15704692567388179 ) ) ;
#30186=CARTESIAN_POINT ( 'NONE',  ( 5.370428668309080500, 20.06498911391418360, -31.65704692567386402 ) ) ;
#30198=CARTESIAN_POINT ( 'NONE',  ( 0.7417250638684235176, 23.11142975074950101, -34.19295307432605568 ) ) ;
#30218=CARTESIAN_POINT ( 'NONE',  ( -0.6505131845895224529, 13.39282139548194195, -46.19999999999996021 ) ) ;
#30228=CARTESIAN_POINT ( 'NONE',  ( -0.6505131845895224529, 13.39282139548194195, -64.19999999999996021 ) ) ;
#30230=CARTESIAN_POINT ( 'NONE',  ( -2.837105286290963146, 12.26822144673588255, -53.85704692567387042 ) ) ;
#30231=CARTESIAN_POINT ( 'NONE',  ( 2.568848540478311460, 12.45835086740561692, -48.89999999999997016 ) ) ;
#30246=CARTESIAN_POINT ( 'NONE',  ( -0.7798958854283041253, 23.40020640687986386, -49.05704692567388037 ) ) ;
#30250=CARTESIAN_POINT ( 'NONE',  ( 2.698247469942395949, 12.52428291510489977, -59.39295307432605853 ) ) ;
#30266=CARTESIAN_POINT ( 'NONE',  ( 2.568848540478311460, 12.45835086740561692, -36.89999999999997016 ) ) ;
#30269=CARTESIAN_POINT ( 'NONE',  ( 3.639207298612508801, 15.48273827966686866, -50.10704692567387752 ) ) ;
#30270=CARTESIAN_POINT ( 'NONE',  ( -1.985016409143819605, 13.60418594181426855, -70.34999999999993747 ) ) ;
#30277=CARTESIAN_POINT ( 'NONE',  ( -1.985016409143819605, 13.60418594181426855, -58.34999999999995879 ) ) ;
#30279=CARTESIAN_POINT ( 'NONE',  ( -2.121074495332175847, 13.67351099933674341, -35.85704692567387752 ) ) ;
#30291=CARTESIAN_POINT ( 'NONE',  ( -2.439449611014227859, 22.60758118029364283, -69.90704692567388179 ) ) ;
#30296=CARTESIAN_POINT ( 'NONE',  ( 5.301103610786608300, 20.20104720010253985, -36.14999999999994884 ) ) ;
#30313=CARTESIAN_POINT ( 'NONE',  ( 5.588711115410763597, 18.38516488214980882, -57.29999999999996874 ) ) ;
#30318=CARTESIAN_POINT ( 'NONE',  ( -0.6839900399647736995, 21.81854315085035623, -32.54999999999996163 ) ) ;
#30319=CARTESIAN_POINT ( 'NONE',  ( 3.705139346311793869, 15.61213720913094960, -69.59999999999996589 ) ) ;
#30330=CARTESIAN_POINT ( 'NONE',  ( -4.084459969179292216, 16.70604699712905372, -42.29295307432605711 ) ) ;
#30334=CARTESIAN_POINT ( 'NONE',  ( 0.8348115903393232839, 13.20534463599456387, -65.54295307432606421 ) ) ;
#30354=CARTESIAN_POINT ( 'NONE',  ( 5.588711115410763597, 18.38516488214980882, -63.29999999999996874 ) ) ;
#30374=CARTESIAN_POINT ( 'NONE',  ( -5.231778553264134324, 14.66289471370907727, -57.14295307432605142 ) ) ;
#30383=CARTESIAN_POINT ( 'NONE',  ( -3.826489000663265472, 15.37892550466785480, -72.14295307432605853 ) ) ;
#30385=CARTESIAN_POINT ( 'NONE',  ( -3.639207298612509689, 19.51726172033310647, -63.60704692567387752 ) ) ;
#30397=CARTESIAN_POINT ( 'NONE',  ( 2.837105286290961370, 22.73177855326409613, -28.35704692567387397 ) ) ;
#30399=CARTESIAN_POINT ( 'NONE',  ( 0.6505131845895220088, 21.60717860451803674, -50.69999999999996732 ) ) ;
#30411=CARTESIAN_POINT ( 'NONE',  ( -0.5070733663080690956, 13.37010276014318144, -71.69295307432605568 ) ) ;
#30429=CARTESIAN_POINT ( 'NONE',  ( 4.107178604518054499, 18.15051318458946383, -48.29999999999996874 ) ) ;
#30439=CARTESIAN_POINT ( 'NONE',  ( -3.705139346311794313, 19.38786279086902198, -68.09999999999996589 ) ) ;
#30441=CARTESIAN_POINT ( 'NONE',  ( -4.099003336600151925, 21.81495595370741469, -51.75704692567388321 ) ) ;
#30442=CARTESIAN_POINT ( 'NONE',  ( 5.588711115410763597, 18.38516488214980882, -48.29999999999996874 ) ) ;
#30455=CARTESIAN_POINT ( 'NONE',  ( -4.099003336600151925, 21.81495595370741469, -36.75704692567386900 ) ) ;
#30459=CARTESIAN_POINT ( 'NONE',  ( -3.898383833589191827, 13.39623302270000771, -50.99295307432605995 ) ) ;
#30475=CARTESIAN_POINT ( 'NONE',  ( -5.876318620034919782, 18.43071743580290089, -34.94999999999996732 ) ) ;
#30478=CARTESIAN_POINT ( 'NONE',  ( 4.129897239856814117, 18.00707336630801336, -46.80704692567388037 ) ) ;
#30479=CARTESIAN_POINT ( 'NONE',  ( -3.091735541773221296, 20.59173554177323950, -71.24999999999994316 ) ) ;
#30487=CARTESIAN_POINT ( 'NONE',  ( -4.107178604518053611, 16.84948681541050775, -55.79999999999996874 ) ) ;
#30489=CARTESIAN_POINT ( 'NONE',  ( -0.5331684895902242260, 21.84243093769531185, -37.05704692567387326 ) ) ;
#30490=CARTESIAN_POINT ( 'NONE',  ( 4.001075405444606048, 21.50107540544455276, -74.99999999999997158 ) ) ;
#30499=CARTESIAN_POINT ( 'NONE',  ( -5.611429750749524992, 16.75827493613162034, -66.30704692567387326 ) ) ;
#30505=CARTESIAN_POINT ( 'NONE',  ( -2.701047200102606016, 12.19889638921340413, -40.34999999999996589 ) ) ;
#30523=CARTESIAN_POINT ( 'NONE',  ( -4.001075405444606936, 13.49892459455542060, -58.49999999999997158 ) ) ;
#30528=CARTESIAN_POINT ( 'NONE',  ( -3.895814058185739448, 15.51498359085620571, -37.64999999999996305 ) ) ;
#30529=CARTESIAN_POINT ( 'NONE',  ( 1.985016409143818272, 21.39581405818570659, -65.84999999999995168 ) ) ;
#30539=CARTESIAN_POINT ( 'NONE',  ( 0.8348115903393232839, 13.20534463599456387, -32.54295307432605711 ) ) ;
#30545=CARTESIAN_POINT ( 'NONE',  ( -2.017261720333081598, 21.13920729861251857, -57.89295307432605853 ) ) ;
#30564=CARTESIAN_POINT ( 'NONE',  ( -0.8851648821498765418, 11.91128888458923285, -67.19999999999997442 ) ) ;
#30583=CARTESIAN_POINT ( 'NONE',  ( 3.898383833589191383, 21.60376697729997275, -58.49295307432606705 ) ) ;
#30593=CARTESIAN_POINT ( 'NONE',  ( 3.826489000663266360, 19.62107449533211678, -61.64295307432606563 ) ) ;
#30595=CARTESIAN_POINT ( 'NONE',  ( 0.5331684895902240040, 13.15756906230466328, -59.55704692567387326 ) ) ;
#30607=CARTESIAN_POINT ( 'NONE',  ( 3.705139346311793869, 15.61213720913094960, -51.59999999999996589 ) ) ;
#30619=CARTESIAN_POINT ( 'NONE',  ( 1.848958322955461808, 21.46513911570817612, -73.34295307432607558 ) ) ;
#30635=CARTESIAN_POINT ( 'NONE',  ( 1.985016409143818272, 21.39581405818570659, -41.84999999999996589 ) ) ;
#30640=CARTESIAN_POINT ( 'NONE',  ( -3.705139346311794313, 19.38786279086902198, -32.09999999999996589 ) ) ;
#30650=CARTESIAN_POINT ( 'NONE',  ( -4.318543150850367773, 18.18399003996480801, -61.94999999999997442 ) ) ;
#30653=CARTESIAN_POINT ( 'NONE',  ( 4.103766977300021601, 21.39838383358913987, -55.50704692567387610 ) ) ;
#30654=CARTESIAN_POINT ( 'NONE',  ( 0.8851648821498760977, 23.08871111541074228, -38.69999999999996021 ) ) ;
#30667=CARTESIAN_POINT ( 'NONE',  ( 4.103766977300021601, 21.39838383358913987, -34.50704692567386900 ) ) ;
#30670=CARTESIAN_POINT ( 'NONE',  ( -4.314955953707389824, 21.59900333660018390, -51.74295307432605995 ) ) ;
#30687=CARTESIAN_POINT ( 'NONE',  ( -4.314955953707389824, 21.59900333660018390, -72.74295307432603863 ) ) ;
#30690=CARTESIAN_POINT ( 'NONE',  ( 1.758463861404912620, 13.72892860598888731, -47.40704692567387468 ) ) ;
#30691=CARTESIAN_POINT ( 'NONE',  ( 3.091735541773220852, 14.40826445822673563, -72.74999999999995737 ) ) ;
#30698=CARTESIAN_POINT ( 'NONE',  ( -3.895814058185739448, 15.51498359085620571, -49.64999999999995595 ) ) ;
#30702=CARTESIAN_POINT ( 'NONE',  ( 4.294655364005415699, 16.66518840966061887, -37.95704692567387184 ) ) ;
#30716=CARTESIAN_POINT ( 'NONE',  ( -0.7798958854283041253, 23.40020640687986386, -64.05704692567387326 ) ) ;
#30720=CARTESIAN_POINT ( 'NONE',  ( -5.041649132594344884, 20.06884854047834921, -32.09999999999996589 ) ) ;
#30737=CARTESIAN_POINT ( 'NONE',  ( 0.8851648821498760977, 23.08871111541074228, -62.69999999999996732 ) ) ;
#30741=CARTESIAN_POINT ( 'NONE',  ( -3.043106805520194413, 14.66227633819065623, -69.00704692567386189 ) ) ;
#30742=CARTESIAN_POINT ( 'NONE',  ( -0.6505131845895224529, 13.39282139548194195, -64.19999999999996021 ) ) ;
#30753=CARTESIAN_POINT ( 'NONE',  ( 2.837723661809363307, 20.54310680552015356, -40.49295307432605995 ) ) ;
#30757=CARTESIAN_POINT ( 'NONE',  ( 0.8348115903393232839, 13.20534463599456387, -56.54295307432606421 ) ) ;
#30773=CARTESIAN_POINT ( 'NONE',  ( 5.588711115410763597, 18.38516488214980882, -60.29999999999996163 ) ) ;
#30794=CARTESIAN_POINT ( 'NONE',  ( -2.564989113914250662, 12.12957133169093282, -56.84295307432604716 ) ) ;
#30803=CARTESIAN_POINT ( 'NONE',  ( -3.199711850326840246, 20.48375923321962233, -60.74295307432605995 ) ) ;
#30805=CARTESIAN_POINT ( 'NONE',  ( -3.639207298612509689, 19.51726172033310647, -57.60704692567387752 ) ) ;
#30818=CARTESIAN_POINT ( 'NONE',  ( -1.887862790868997553, 21.20513934631180319, -41.39999999999996305 ) ) ;
#30829=CARTESIAN_POINT ( 'NONE',  ( -3.771071394011080269, 19.25846386140493394, -75.59295307432606137 ) ) ;
#30846=CARTESIAN_POINT ( 'NONE',  ( 0.6505131845895220088, 21.60717860451803674, -38.69999999999996021 ) ) ;
#30851=CARTESIAN_POINT ( 'NONE',  ( -0.6839900399647736995, 21.81854315085035623, -35.54999999999994742 ) ) ;
#30860=CARTESIAN_POINT ( 'NONE',  ( 3.091735541773220852, 14.40826445822673563, -60.74999999999995737 ) ) ;
#30862=CARTESIAN_POINT ( 'NONE',  ( -5.611429750749524992, 16.75827493613162034, -42.30704692567387326 ) ) ;
#30863=CARTESIAN_POINT ( 'NONE',  ( -5.041649132594344884, 20.06884854047834921, -35.09999999999996589 ) ) ;
#30866=CARTESIAN_POINT ( 'NONE',  ( -3.705139346311794313, 19.38786279086902198, -71.09999999999996589 ) ) ;
#30877=CARTESIAN_POINT ( 'NONE',  ( 4.099003336600150149, 13.18504404629255689, -38.25704692567386900 ) ) ;
#30883=CARTESIAN_POINT ( 'NONE',  ( -5.565992480072003978, 16.47139529956871229, -48.29295307432606421 ) ) ;
#30901=CARTESIAN_POINT ( 'NONE',  ( 2.564989113914249330, 22.87042866830903876, -73.34295307432607558 ) ) ;
#30904=CARTESIAN_POINT ( 'NONE',  ( 2.983759233219601459, 14.30028814967311668, -41.25704692567387610 ) ) ;
#30905=CARTESIAN_POINT ( 'NONE',  ( -1.985016409143819605, 13.60418594181426855, -31.34999999999996945 ) ) ;
#30906=CARTESIAN_POINT ( 'NONE',  ( 3.705139346311793869, 15.61213720913094960, -66.59999999999996589 ) ) ;
#30917=CARTESIAN_POINT ( 'NONE',  ( -4.975717084895059372, 20.19824746994243370, -72.60704692567387042 ) ) ;
#30918=CARTESIAN_POINT ( 'NONE',  ( -5.041649132594344884, 20.06884854047834921, -65.09999999999996589 ) ) ;
#30929=CARTESIAN_POINT ( 'NONE',  ( 2.439449611014226971, 12.39241881970633230, -65.40704692567388179 ) ) ;
#30933=CARTESIAN_POINT ( 'NONE',  ( 0.8851648821498760977, 23.08871111541074228, -26.69999999999996732 ) ) ;
#30949=CARTESIAN_POINT ( 'NONE',  ( 5.876318620034919782, 16.56928256419707068, -54.44999999999996021 ) ) ;
#30953=CARTESIAN_POINT ( 'NONE',  ( -1.758463861404912842, 21.27107139401109137, -72.90704692567388179 ) ) ;
#30954=CARTESIAN_POINT ( 'NONE',  ( 3.895814058185739892, 19.48501640914376054, -54.14999999999997016 ) ) ;
#30966=CARTESIAN_POINT ( 'NONE',  ( 4.084459969179292216, 18.29395300287091430, -37.79295307432605711 ) ) ;
#30969=CARTESIAN_POINT ( 'NONE',  ( -2.837723661809363751, 14.45689319447982335, -50.99295307432605995 ) ) ;
#30984=CARTESIAN_POINT ( 'NONE',  ( -0.9307174358028533767, 23.37631862003491889, -53.54999999999996163 ) ) ;
#31006=CARTESIAN_POINT ( 'NONE',  ( 0.7417250638684235176, 23.11142975074950101, -55.19295307432606279 ) ) ;
#31014=CARTESIAN_POINT ( 'NONE',  ( -3.771071394011080269, 19.25846386140493394, -63.59295307432605426 ) ) ;
#31016=CARTESIAN_POINT ( 'NONE',  ( 4.129897239856814117, 18.00707336630801336, -52.80704692567387326 ) ) ;
#31028=CARTESIAN_POINT ( 'NONE',  ( 3.705139346311793869, 15.61213720913094960, -48.59999999999996589 ) ) ;
#31038=CARTESIAN_POINT ( 'NONE',  ( -3.771071394011080269, 19.25846386140493394, -69.59295307432604716 ) ) ;
#31051=CARTESIAN_POINT ( 'NONE',  ( -2.940415233664778860, 14.55958476633523802, -37.49999999999996447 ) ) ;
#31056=CARTESIAN_POINT ( 'NONE',  ( -2.940415233664778860, 14.55958476633523802, -31.49999999999996447 ) ) ;
#31065=CARTESIAN_POINT ( 'NONE',  ( 3.091735541773220852, 14.40826445822673563, -57.74999999999995737 ) ) ;
#31067=CARTESIAN_POINT ( 'NONE',  ( -0.7798958854283041253, 23.40020640687986386, -49.05704692567388037 ) ) ;
#31068=CARTESIAN_POINT ( 'NONE',  ( -5.876318620034919782, 18.43071743580290089, -34.94999999999996732 ) ) ;
#31071=CARTESIAN_POINT ( 'NONE',  ( -1.887862790868997553, 21.20513934631180319, -74.39999999999996305 ) ) ;
#31082=CARTESIAN_POINT ( 'NONE',  ( 4.975717084895059372, 14.80175253005754143, -32.10704692567387042 ) ) ;
#31087=CARTESIAN_POINT ( 'NONE',  ( 5.107581180293630396, 15.06055038898570686, -47.09295307432606137 ) ) ;
#31103=CARTESIAN_POINT ( 'NONE',  ( -1.081538986177402961, 23.35243083318996327, -73.04295307432606421 ) ) ;
#31106=CARTESIAN_POINT ( 'NONE',  ( 3.965139115708213868, 19.34895832295540430, -46.65704692567388179 ) ) ;
#31107=CARTESIAN_POINT ( 'NONE',  ( 3.895814058185739448, 19.48501640914375344, -33.14999999999996305 ) ) ;
#31108=CARTESIAN_POINT ( 'NONE',  ( -0.6505131845895224529, 13.39282139548194195, -67.19999999999997442 ) ) ;
#31118=CARTESIAN_POINT ( 'NONE',  ( -2.121074495332175847, 13.67351099933674341, -26.85704692567387397 ) ) ;
#31119=CARTESIAN_POINT ( 'NONE',  ( 0.8851648821498760977, 23.08871111541074228, -62.69999999999996732 ) ) ;
#31130=CARTESIAN_POINT ( 'NONE',  ( -4.103766977300021601, 13.60161616641083704, -63.00704692567389031 ) ) ;
#31135=CARTESIAN_POINT ( 'NONE',  ( 2.564989113914249330, 22.87042866830903876, -76.34295307432604716 ) ) ;
#31149=CARTESIAN_POINT ( 'NONE',  ( 0.8851648821498760977, 23.08871111541074228, -50.69999999999996732 ) ) ;
#31153=CARTESIAN_POINT ( 'NONE',  ( -1.758463861404912842, 21.27107139401109137, -69.90704692567388179 ) ) ;
#31154=CARTESIAN_POINT ( 'NONE',  ( 1.985016409143818272, 21.39581405818570659, -56.84999999999996589 ) ) ;
#31165=CARTESIAN_POINT ( 'NONE',  ( -0.8348115903393239501, 21.79465536400541126, -40.04295307432605000 ) ) ;
#31168=CARTESIAN_POINT ( 'NONE',  ( -4.084459969179292216, 16.70604699712905372, -57.29295307432606421 ) ) ;
#31184=CARTESIAN_POINT ( 'NONE',  ( -5.876318620034919782, 18.43071743580290089, -58.94999999999995310 ) ) ;
#31205=CARTESIAN_POINT ( 'NONE',  ( -3.898383833589191827, 13.39623302270000771, -47.99295307432606705 ) ) ;
#31214=CARTESIAN_POINT ( 'NONE',  ( 4.084459969179292216, 18.29395300287091430, -64.79295307432606421 ) ) ;
#31228=CARTESIAN_POINT ( 'NONE',  ( 3.091735541773220852, 14.40826445822673563, -45.74999999999995737 ) ) ;
#31253=CARTESIAN_POINT ( 'NONE',  ( 4.318543150850366885, 16.81600996003516713, -39.44999999999996021 ) ) ;
#31257=CARTESIAN_POINT ( 'NONE',  ( 1.985016409143818272, 21.39581405818570303, -32.84999999999996589 ) ) ;
#31266=CARTESIAN_POINT ( 'NONE',  ( -1.887862790868997553, 21.20513934631180319, -56.39999999999996305 ) ) ;
#31268=CARTESIAN_POINT ( 'NONE',  ( 4.975717084895059372, 14.80175253005754143, -47.10704692567387042 ) ) ;
#31269=CARTESIAN_POINT ( 'NONE',  ( 2.701047200102605128, 22.80110361078656211, -35.84999999999996589 ) ) ;
#31272=CARTESIAN_POINT ( 'NONE',  ( -3.199711850326840246, 20.48375923321962233, -30.74295307432605640 ) ) ;
#31283=CARTESIAN_POINT ( 'NONE',  ( -0.8851648821498765418, 11.91128888458923285, -73.19999999999997442 ) ) ;
#31288=CARTESIAN_POINT ( 'NONE',  ( 1.081538986177402295, 11.64756916681001186, -53.54295307432606421 ) ) ;
#31307=CARTESIAN_POINT ( 'NONE',  ( 5.231778553264135212, 20.33710528629089254, -70.64295307432605853 ) ) ;
#31311=CARTESIAN_POINT ( 'NONE',  ( -4.294655364005415699, 18.33481159033935626, -39.45704692567387184 ) ) ;
#31314=CARTESIAN_POINT ( 'NONE',  ( 4.107178604518054499, 18.15051318458946383, -30.29999999999996518 ) ) ;
#31315=CARTESIAN_POINT ( 'NONE',  ( -0.6505131845895224529, 13.39282139548194195, -64.19999999999996021 ) ) ;
#31326=CARTESIAN_POINT ( 'NONE',  ( 4.129897239856814117, 18.00707336630801336, -28.80704692567387326 ) ) ;
#31327=CARTESIAN_POINT ( 'NONE',  ( 4.001075405444606048, 21.50107540544455276, -68.99999999999995737 ) ) ;
#31337=CARTESIAN_POINT ( 'NONE',  ( 1.028604700431328567, 23.06599248007198355, -61.20704692567387184 ) ) ;
#31342=CARTESIAN_POINT ( 'NONE',  ( 0.9307174358028528216, 11.62368137996505801, -28.04999999999995453 ) ) ;
#31357=CARTESIAN_POINT ( 'NONE',  ( 2.701047200102605572, 22.80110361078655856, -47.84999999999994458 ) ) ;
#31361=CARTESIAN_POINT ( 'NONE',  ( 2.983759233219601459, 14.30028814967311668, -68.25704692567387610 ) ) ;
#31362=CARTESIAN_POINT ( 'NONE',  ( 4.107178604518054499, 18.15051318458946383, -60.29999999999996163 ) ) ;
#31366=AXIS2_PLACEMENT_3D ( 'NONE', #20654, #11082, #36603 ) ;
#31375=CARTESIAN_POINT ( 'NONE',  ( 4.342430937695320736, 16.96683151040971538, -37.94295307432606279 ) ) ;
#31378=CARTESIAN_POINT ( 'NONE',  ( 4.084459969179292216, 18.29395300287091430, -52.79295307432607132 ) ) ;
#31392=CARTESIAN_POINT ( 'NONE',  ( 5.588711115410763597, 18.38516488214980882, -54.29999999999996874 ) ) ;
#31416=CARTESIAN_POINT ( 'NONE',  ( -2.564989113914250662, 12.12957133169093282, -47.84295307432606137 ) ) ;
#31423=CARTESIAN_POINT ( 'NONE',  ( 4.084459969179292216, 18.29395300287091430, -67.79295307432606421 ) ) ;
#31435=CARTESIAN_POINT ( 'NONE',  ( 2.940415233664778416, 20.44041523366473712, -47.99999999999996447 ) ) ;
#31461=CARTESIAN_POINT ( 'NONE',  ( -3.705139346311794313, 19.38786279086902198, -26.09999999999996234 ) ) ;
#31468=CARTESIAN_POINT ( 'NONE',  ( -3.091735541773221296, 20.59173554177323950, -38.24999999999996447 ) ) ;
#31477=CARTESIAN_POINT ( 'NONE',  ( -4.107178604518053611, 16.84948681541050775, -55.79999999999996874 ) ) ;
#31479=CARTESIAN_POINT ( 'NONE',  ( -4.099003336600151925, 21.81495595370741469, -48.75704692567386189 ) ) ;
#31480=CARTESIAN_POINT ( 'NONE',  ( -5.588711115410763597, 16.61483511785016987, -40.79999999999996874 ) ) ;
#31482=CARTESIAN_POINT ( 'NONE',  ( 4.342430937695320736, 16.96683151040971538, -28.94295307432605568 ) ) ;
#31493=CARTESIAN_POINT ( 'NONE',  ( 1.028604700431328567, 23.06599248007198355, -28.20704692567387184 ) ) ;
#31498=CARTESIAN_POINT ( 'NONE',  ( -4.314955953707389824, 21.59900333660018390, -42.74295307432605284 ) ) ;
#31515=( LENGTH_UNIT ( ) NAMED_UNIT ( * ) SI_UNIT ( .MILLI., .METRE. ) );
#31516=CARTESIAN_POINT ( 'NONE',  ( -5.565992480072003978, 16.47139529956871229, -75.29295307432605000 ) ) ;
#31521=CARTESIAN_POINT ( 'NONE',  ( -1.887862790868997553, 21.20513934631180319, -35.39999999999996305 ) ) ;
#31522=CARTESIAN_POINT ( 'NONE',  ( -0.6839900399647736995, 21.81854315085035623, -59.54999999999994742 ) ) ;
#31533=CARTESIAN_POINT ( 'NONE',  ( -2.983759233219601903, 20.69971185032686023, -30.75704692567387610 ) ) ;
#31534=CARTESIAN_POINT ( 'NONE',  ( 5.301103610786608300, 20.20104720010254340, -69.14999999999996305 ) ) ;
#31544=CARTESIAN_POINT ( 'NONE',  ( -4.975717084895059372, 20.19824746994243370, -54.60704692567387752 ) ) ;
#31547=CARTESIAN_POINT ( 'NONE',  ( 5.041649132594343996, 14.93115145952162415, -30.59999999999996589 ) ) ;
#31566=CARTESIAN_POINT ( 'NONE',  ( 2.568848540478311460, 12.45835086740561692, -54.89999999999996305 ) ) ;
#31570=CARTESIAN_POINT ( 'NONE',  ( 0.6505131845895220088, 21.60717860451803674, -26.69999999999996732 ) ) ;
#31571=CARTESIAN_POINT ( 'NONE',  ( -3.705139346311794313, 19.38786279086902198, -62.09999999999996589 ) ) ;
#31579=CARTESIAN_POINT ( 'NONE',  ( 3.091735541773220852, 14.40826445822673563, -72.74999999999995737 ) ) ;
#31583=CARTESIAN_POINT ( 'NONE',  ( 0.6505131845895220088, 21.60717860451803674, -71.69999999999997442 ) ) ;
#31586=CARTESIAN_POINT ( 'NONE',  ( 2.017261720333081598, 13.86079270138745834, -44.39295307432605853 ) ) ;
#31604=CARTESIAN_POINT ( 'NONE',  ( 2.568848540478311460, 12.45835086740561692, -57.89999999999996305 ) ) ;
#31625=CARTESIAN_POINT ( 'NONE',  ( -0.7417250638684240727, 11.88857024925047057, -47.69295307432606279 ) ) ;
#31632=CARTESIAN_POINT ( 'NONE',  ( -4.084459969179292216, 16.70604699712905372, -60.29295307432605000 ) ) ;
#31646=CARTESIAN_POINT ( 'NONE',  ( 4.318543150850367773, 16.81600996003516357, -45.44999999999996021 ) ) ;
#31669=CARTESIAN_POINT ( 'NONE',  ( 1.985016409143818272, 21.39581405818570659, -29.84999999999996589 ) ) ;
#31674=CARTESIAN_POINT ( 'NONE',  ( 4.318543150850367773, 16.81600996003516357, -30.44999999999995310 ) ) ;
#31683=CARTESIAN_POINT ( 'NONE',  ( -3.091735541773221296, 20.59173554177323950, -59.24999999999997158 ) ) ;
#31685=CARTESIAN_POINT ( 'NONE',  ( -5.611429750749524992, 16.75827493613162034, -48.30704692567388037 ) ) ;
#31687=CARTESIAN_POINT ( 'NONE',  ( 2.564989113914249330, 22.87042866830903876, -40.34295307432606137 ) ) ;
#31688=CARTESIAN_POINT ( 'NONE',  ( -2.017261720333081598, 21.13920729861251857, -30.89295307432606208 ) ) ;
#31700=CARTESIAN_POINT ( 'NONE',  ( -4.103766977300021601, 13.60161616641083704, -30.00704692567387610 ) ) ;
#31704=CARTESIAN_POINT ( 'NONE',  ( -5.900206406879871857, 18.27989588542834554, -42.44295307432605568 ) ) ;
#31719=CARTESIAN_POINT ( 'NONE',  ( 3.898383833589191383, 21.60376697729997275, -64.49295307432606705 ) ) ;
#31724=CARTESIAN_POINT ( 'NONE',  ( 3.705139346311793869, 15.61213720913094960, -39.59999999999996589 ) ) ;
#31725=CARTESIAN_POINT ( 'NONE',  ( 0.6839900399647733664, 13.18145684914961357, -67.04999999999994031 ) ) ;
#31736=CARTESIAN_POINT ( 'NONE',  ( -3.965139115708213868, 15.65104167704456906, -30.15704692567386758 ) ) ;
#31737=CARTESIAN_POINT ( 'NONE',  ( -5.301103610786608300, 14.79895279989743528, -67.64999999999997726 ) ) ;
#31749=CARTESIAN_POINT ( 'NONE',  ( -2.837105286290963146, 12.26822144673588255, -56.85704692567387042 ) ) ;
#31752=CARTESIAN_POINT ( 'NONE',  ( 5.900206406879871857, 16.72010411457162604, -70.94295307432606990 ) ) ;
#31767=CARTESIAN_POINT ( 'NONE',  ( -5.876318620034919782, 18.43071743580290089, -52.94999999999994600 ) ) ;
#31771=CARTESIAN_POINT ( 'NONE',  ( 3.043106805520193525, 20.33772366180932067, -61.50704692567389031 ) ) ;
#31772=CARTESIAN_POINT ( 'NONE',  ( 4.318543150850366885, 16.81600996003516713, -57.44999999999996021 ) ) ;
#31779=CARTESIAN_POINT ( 'NONE',  ( -3.895814058185739448, 15.51498359085620571, -64.64999999999994884 ) ) ;
#31781=CARTESIAN_POINT ( 'NONE',  ( 0.5331684895902240040, 13.15756906230466328, -50.55704692567388747 ) ) ;
#31785=CARTESIAN_POINT ( 'NONE',  ( -3.091735541773221296, 20.59173554177323950, -71.24999999999994316 ) ) ;
#31788=CARTESIAN_POINT ( 'NONE',  ( -0.8348115903393239501, 21.79465536400541126, -46.04295307432605711 ) ) ;
#31802=CARTESIAN_POINT ( 'NONE',  ( -5.301103610786608300, 14.79895279989743706, -43.64999999999996305 ) ) ;
#31824=CARTESIAN_POINT ( 'NONE',  ( 3.705139346311793869, 15.61213720913094960, -45.59999999999996589 ) ) ;
#31826=CARTESIAN_POINT ( 'NONE',  ( -5.231778553264134324, 14.66289471370907727, -48.14295307432606563 ) ) ;
#31838=CARTESIAN_POINT ( 'NONE',  ( 3.199711850326839357, 14.51624076678035635, -59.24295307432605995 ) ) ;
#31854=CARTESIAN_POINT ( 'NONE',  ( -1.985016409143819605, 13.60418594181426855, -34.34999999999995879 ) ) ;
#31878=CARTESIAN_POINT ( 'NONE',  ( 4.107178604518054499, 18.15051318458946383, -27.29999999999996163 ) ) ;
#31882=CARTESIAN_POINT ( 'NONE',  ( 3.898383833589191383, 21.60376697729997275, -34.49295307432605995 ) ) ;
#31883=CARTESIAN_POINT ( 'NONE',  ( 0.7939530028709752552, 21.58445996917927445, -73.20704692567387895 ) ) ;
#31892=CARTESIAN_POINT ( 'NONE',  ( 2.940415233664778416, 20.44041523366473712, -47.99999999999996447 ) ) ;
#31895=CARTESIAN_POINT ( 'NONE',  ( -4.099003336600151925, 21.81495595370741469, -39.75704692567386900 ) ) ;
#31896=CARTESIAN_POINT ( 'NONE',  ( 2.568848540478311460, 12.45835086740561692, -27.89999999999996660 ) ) ;
#31897=CARTESIAN_POINT ( 'NONE',  ( -0.6839900399647736995, 21.81854315085035623, -65.54999999999996874 ) ) ;
#31908=CARTESIAN_POINT ( 'NONE',  ( 4.206979645153767322, 13.29302035484617051, -72.74999999999995737 ) ) ;
#31913=CARTESIAN_POINT ( 'NONE',  ( -5.107581180293630396, 19.93944961101426827, -45.59295307432606137 ) ) ;
#31922=DIRECTION ( 'NONE',  ( -0.7037848285661852943, 0.7037848285661920666, -0.09681854243956063144 ) ) ;
#31930=CARTESIAN_POINT ( 'NONE',  ( 0.7417250638684235176, 23.11142975074950101, -64.19295307432605568 ) ) ;
#31936=CARTESIAN_POINT ( 'NONE',  ( 1.887862790868997109, 13.79486065368817194, -27.89999999999996660 ) ) ;
#31937=CARTESIAN_POINT ( 'NONE',  ( 4.107178604518054499, 18.15051318458946383, -57.29999999999996874 ) ) ;
#31949=CARTESIAN_POINT ( 'NONE',  ( 4.099003336600150149, 13.18504404629255689, -62.25704692567386900 ) ) ;
#31950=CARTESIAN_POINT ( 'NONE',  ( -5.588711115410763597, 16.61483511785016987, -58.79999999999996163 ) ) ;
#31961=CARTESIAN_POINT ( 'NONE',  ( 2.439449611014226971, 12.39241881970633230, -53.40704692567386758 ) ) ;
#31965=CARTESIAN_POINT ( 'NONE',  ( -2.564989113914250662, 12.12957133169093282, -68.84295307432606137 ) ) ;
#31982=( BOUNDED_SURFACE ( )  B_SPLINE_SURFACE ( 3, 2, ( 
 ( #23905, #23253, #4324, #7733, #30054, #3898, #4534, #7093, #26662, #20493, #20707, #39623, #20070, #1349, #1142, #30691, #27509, #13895, #10495, #17307, #7305, #26876, #39845, #20910, #14112, #30479, #14322, #10707, #33461, #16879, #33882, #30270, #27085, #33032, #40052, #27302, #40267, #11136, #4743, #10283, #40675, #1766, #24526, #37493, #11533, #14747, #8977, #8143, #2391, #37703, #8348, #25153, #31108, #31725, #5793, #21739, #30906, #12162, #24319, #18767, #34505, #21327, #34090, #38118, #18341, #8560, #34713, #28329, #1962, #21948, #2593, #41315, #31315, #34301, #5164, #34923, #5363, #27704, #14946, #15157, #21119, #2174, #37909, #15578, #17930, #40477, #27914, #15381, #11332, #21537, #28121, #41107, #11955, #18138, #37288, #4948, #40888, #11743, #24738, #24949, #8766, #5581, #18553, #31522, #41947, #22789, #25777, #25365, #35554, #38535, #5996, #35341, #19181, #19586, #22364, #233, #9615, #32558, #31937, #32153, #32360, #41527, #3425, #6207, #12379, #2809, #15792, #19797, #41735, #35762, #12795, #25573, #35133, #28, #18970, #3634, #38322, #13215, #6623, #32767, #25990, #38744, #28537, #3017, #26201, #12590, #22579, #28739, #13010, #22991, #16008, #28951, #16418, #39149, #29364, #35961, #6416, #10031, #9186, #9401, #19388, #3224, #22164, #16207, #6824, #29151, #38955, #9831, #24068, #20229, #4488, #20017, #32982, #16828, #20655, #20441, #7468, #36168, #30429, #27251, #30003, #26612, #39796, #1299, #40002, #7257, #10448, #7683, #3849, #10869, #23424, #14271, #30218, #13628, #23201, #1095, #7039, #33835, #445, #40213, #23856, #7893, #14066, #876, #16621, #36390, #11084, #655, #13846, #29791, #27039, #37034, #33191, #4055, #36821, #20862, #33633, #29581, #17040, #17470, #26401, #39573, #26827, #10661, #13416, #23641, #39351, #36604, #33409, #17257, #10231, #4274, #34657, #8090, #21067, #4898, #8710, #8502, #37646, #24266, #18498, #15322, #18084, #14694, #27857, #31468, #28067, #37442, #40623, #37853, #34041, #41047, #11481, #2335, #18285, #14889, #11899, #5524, #8297, #28277, #38061, #41260, #21479, #30851, #24472, #12105, #40834, #17878, #21276, #34451, #27456, #11686, #2120, #25098, #37236, #8920, #34245, #21684, #21892, #24685, #5312, #31257, #15104, #1711, #4693, #17673, #30640, #27652, #1505, #5105, #31056, #1908, #24891, #14484, #40422, #11282, #32099, #31674, #41902, #2752, #12322, #41682, #25523, #25941, #28690, #6579, #15956, #38905, #38268, #38487, #38694, #5739, #9783, #12537, #18715, #9133, #22110, #26154, #5942, #42107, #6154, #35082, #16169, #35717, #9565, #35506, #187, #12750, #2965, #28905, #3180 ),
 ( #18916, #19133, #31883, #19339, #29315, #9349, #22315, #12960, #32516, #22741, #13167, #35292, #19544, #2542, #15736, #25730, #22522, #15526, #6365, #3385, #32313, #29108, #16372, #39105, #9985, #34871, #28482, #41472, #25305, #26993, #26784, #13804, #401, #36771, #33586, #36342, #32938, #4010, #7633, #4228, #13583, #16786, #14022, #26357, #17210, #29745, #20607, #36556, #33146, #30173, #10821, #26567, #4447, #14225, #23806, #39749, #6995, #608, #17427, #16994, #10187, #39526, #10616, #3585, #29956, #20396, #30385, #13376, #1255, #10403, #39956, #27204, #830, #23596, #7421, #33359, #36123, #40169, #22947, #35915, #39308, #6782, #23379, #7214, #20186, #1049, #19755, #32721, #16580, #29535, #23157, #19971, #3803, #30595, #17831, #1666, #2654, #4853, #25424, #34201, #15641, #14438, #14652, #15432, #24019, #28598, #30805, #36992, #27413, #27615, #41585, #20823, #24225, #8254, #40583, #7853, #18041, #12441, #21230, #11439, #12222, #19033, #24430, #38388, #40382, #11243, #37195, #9250, #28387, #2448, #1463, #22221, #35188, #37398, #21023, #5061, #6054, #34987, #31016, #41373, #32001, #8049, #5851, #25210, #2867, #38172, #9036, #18821, #15858, #22014, #28804, #11037, #33795, #31781, #33999, #4650, #17629, #35819, #29014, #16271, #16476, #22427, #6680, #39209, #36231, #19244, #505, #29212, #16685, #29641, #22849, #29426, #297, #13278, #12861, #26463, #7104, #13477, #16072, #3696, #87, #13067, #3285, #23053, #26261, #26051, #36022, #39012, #38595, #19651, #9680, #32216, #6481, #32418, #32827, #35618, #39417, #32620, #10294, #3081, #9893, #3486, #12655, #23263, #19452, #25634, #42010, #25841, #33043, #38806, #6885, #10090, #22642, #6269, #19860, #20079, #16890, #9460, #3908, #41801, #35405, #27311, #14120, #4958, #7530, #14548, #13906, #1152, #30064, #14332, #24329, #36665, #20501, #37098, #27520, #33894, #37298, #30702, #17318, #4753, #17730, #10930, #17524, #30489, #1358, #940, #40488, #8153, #1570, #4117, #11342, #30279, #27095, #33471, #11146, #4545, #40063, #24130, #23914, #26673, #36882, #39854, #7316, #4333, #7744, #20920, #23702, #21128, #20718, #34099, #33252, #33694, #40277, #721, #29855, #7954, #13692, #17102, #26887, #39634, #10714, #10508, #23490, #36452, #20286, #31533, #37501, #35144, #1775, #31736, #25164, #9198, #15389, #2185, #17939, #37715, #2605, #1971, #31326, #18147, #2401, #12391, #24748, #8570, #38128, #15591, #21959, #25376, #21545, #5804, #27714, #31118, #15167, #11752, #14758, #24960, #8986, #28132, #18352, #18563, #38336, #34515, #18776, #21338, #34311, #14957, #34933, #21751, #8778, #8357, #28549 ),
 ( #28340, #5175, #40687, #41537, #34723, #22174, #30917, #5374, #27923, #11967, #40897, #41118, #37919, #11543, #5592, #41324, #12173, #24535, #6428, #41747, #16632, #29162, #38545, #18983, #16020, #40, #19808, #29374, #38756, #41958, #39158, #9412, #243, #12806, #32777, #19595, #16218, #13225, #35971, #9627, #29591, #39364, #6835, #38964, #32164, #25790, #455, #13020, #35355, #22589, #22800, #28751, #26000, #3435, #13426, #25584, #3643, #35565, #23002, #26411, #9841, #35771, #6632, #32568, #19192, #10242, #23211, #6006, #22376, #10039, #19399, #32371, #3235, #26211, #16427, #31949, #2819, #15803, #12603, #6218, #28962, #3027, #887, #26837, #27263, #30014, #7905, #17267, #40225, #39583, #39808, #40013, #7049, #11095, #13857, #20029, #10458, #23437, #27467, #7269, #1310, #7480, #33202, #667, #7693, #13640, #11292, #32994, #20873, #14284, #40433, #33645, #20454, #36178, #10672, #33844, #20241, #33421, #36402, #20666, #30653, #23654, #36616, #24079, #4704, #37045, #1518, #4285, #17684, #3861, #4066, #30230, #1105, #16840, #14077, #14496, #27050, #10883, #36833, #29802, #23868, #26623, #17051, #4499, #17480, #30441, #28077, #15115, #1724, #38073, #34882, #37657, #15538, #21693, #8514, #41485, #1919, #8931, #8308, #21490, #24484, #8721, #18726, #31067, #14899, #31479, #21903, #28287, #31685, #27868, #12115, #34052, #37453, #34462, #18097, #8101, #31268, #15333, #5322, #24695, #24904, #2555, #40844, #25109, #27663, #40634, #21288, #41271, #41058, #11910, #14705, #5749, #28492, #18295, #34257, #2131, #24276, #5536, #11697, #37863, #37247, #11492, #18510, #34668, #21079, #2346, #4909, #17889, #30862, #5117, #35926, #3598, #196, #3191, #38497, #19143, #6791, #6377, #41693, #28915, #29117, #35093, #19349, #9794, #19765, #31895, #13178, #41912, #29327, #26164, #35518, #35680, #12972, #25953, #25533, #39116, #32732, #9995, #28700, #16383, #12760, #25741, #15966, #35727, #38917, #38706, #6588, #9576, #9145, #32323, #22326, #2763, #32111, #2976, #3394, #6166, #22957, #16178, #16591, #15748, #22534, #22752, #25318, #29546, #19554, #38279, #12547, #9360, #12333, #35303, #32526, #22121, #5954, #18928, #7433, #36133, #1270, #26367, #23819, #30186, #4240, #36568, #20408, #39318, #7645, #33372, #27006, #20198, #39536, #10629, #7006, #26579, #13594, #36785, #19984, #32948, #16796, #17224, #10199, #20620, #10416, #30397, #26797, #29968, #1059, #3815, #29757, #618, #33599, #23607, #23392, #842, #36355, #14034, #411, #7225, #33157, #23168, #4022, #17005, #39968, #13815, #39760, #13387, #10834, #17439, #4458, #9928, #32251, #32037, #19686 ),
 ( #26297, #29049, #19901, #29677, #39242, #29248, #22460, #3116, #32868, #32453, #25671, #12898, #13100, #19067, #3319, #35851, #3731, #15896, #10123, #25877, #13312, #23089, #19485, #26086, #39044, #22885, #9498, #36057, #16717, #6926, #12690, #332, #38839, #9715, #42046, #32657, #6715, #22678, #3520, #35654, #35228, #16308, #6301, #28839, #16107, #6517, #29463, #122, #543, #16513, #13514, #41838, #38425, #9289, #22255, #6089, #2904, #38631, #35441, #19278, #17765, #39676, #33726, #39887, #23527, #33077, #40096, #3942, #7780, #17137, #20321, #17558, #29890, #20754, #33288, #40312, #10963, #36697, #4579, #14366, #30098, #7984, #30737, #27340, #17351, #10545, #4154, #20956, #20535, #13733, #976, #1182, #7144, #33508, #23950, #33927, #16924, #11179, #13946, #1391, #24162, #7561, #14152, #27128, #36915, #36487, #37131, #4787, #1600, #759, #30523, #26923, #10748, #23733, #26501, #39458, #4372, #10333, #30313, #23307, #36271, #7349, #26710, #20114, #5205, #5625, #8389, #28372, #37746, #18603, #17972, #18180, #18389, #27555, #31566, #21368, #40521, #30949, #1806, #5836, #27749, #21785, #27956, #11576, #21159, #28167, #34132, #31767, #11378, #41358, #34757, #18807, #12000, #40933, #14581, #34345, #12209, #40719, #11789, #14786, #41153, #9020, #31149, #2008, #2435, #25199, #15419, #21997, #14991, #38160, #24361, #24569, #24785, #8603, #37332, #21576, #34973, #34550, #5411, #15202, #8185, #31357, #4992, #37534, #2223, #24990, #37954, #8815, #35603, #22205, #16460, #13262, #16054, #12636, #25826, #29410, #72, #39194, #35174, #3469, #32199, #19632, #32606, #38790, #32402, #3268, #16255, #15841, #279, #10071, #26246, #19017, #6664, #3063, #28996, #6251, #26034, #19433, #41994, #38996, #12842, #41570, #9662, #25618, #6040, #9442, #35387, #35802, #38577, #23036, #22624, #36005, #31985, #19227, #6465, #15626, #6872, #22410, #28583, #2851, #28785, #19843, #41783, #9879, #29194, #13051, #9237, #22834, #2639, #12424, #25408, #38371, #40048, #24113, #30266, #17086, #7938, #10489, #17510, #16874, #4102, #33027, #17301, #27297, #39618, #23474, #10917, #30475, #36869, #40262, #36436, #20703, #491, #3892, #30050, #26657, #16667, #39841, #23901, #924, #33238, #33457, #11132, #7300, #33679, #36213, #7087, #29838, #7729, #36651, #23687, #10277, #4530, #1345, #13891, #705, #26871, #14318, #14108, #20271, #10703, #37084, #20065, #27081, #7515, #32810, #4320, #20489, #3681, #29625, #1137, #13460, #26446, #39401, #23248, #13677, #27699, #15375, #14939, #8137, #37488, #37697, #1553, #27908, #2166, #11528, #14742, #11949, #24314, #15151, #40669 ),
 ( #1761, #18548, #11737, #18335, #28115, #24520, #21322, #14533, #31516, #1957, #11328, #33878, #17924, #40881, #8343, #37283, #18133, #34294, #21115, #34086, #4944, #30901, #5159, #31103, #2385, #30687, #24942, #24732, #8553, #5573, #21531, #12156, #28322, #41099, #34499, #34708, #4739, #41308, #5357, #31307, #27505, #25147, #37904, #8760, #21734, #38112, #20906, #17717, #40473, #12371, #36331, #19962, #821, #38315, #32926, #10394, #12789, #9609, #16983, #28944, #19175, #32147, #3792, #22570, #35548, #5787, #7203, #6410, #26558, #9395, #15784, #25771, #28531, #2803, #18964, #20176, #15572, #41521, #22158, #38737, #31719, #33136, #31930, #13794, #41941, #3011, #16776, #25357, #9180, #35127, #3999, #29735, #5990, #16002, #28733, #598, #8969, #41728, #12583, #18760, #25567, #38529, #13574, #22357, #35335, #21941, #39515, #34917, #23368, #29948, #6200, #26774, #2588, #1245, #27606, #1038, #14012, #39945, #1654, #1453, #30583, #17200, #11428, #8244, #11026, #7623, #20812, #24419, #21012, #30374, #33574, #30794, #26983, #33986, #4435, #37386, #11232, #7841, #4843, #40573, #14213, #21220, #31006, #34191, #14426, #23794, #17416, #5049, #33785, #10809, #27191, #27401, #20383, #4641, #37184, #18028, #30161, #1860, #40158, #14640, #14840, #17619, #40372, #8039, #17822, #36760, #39737, #23586, #36545, #20598, #7410, #24012, #36982, #33349, #4218, #2490, #41211, #22055, #25045, #24630, #34818, #37801, #5260, #34605, #18446, #18864, #21628, #41630, #8870, #31826, #31205, #31416, #31625, #40781, #2697, #5468, #11634, #2065, #15051, #19074, #40995, #35029, #12054, #24843, #34400, #41417, #18235, #2911, #37594, #12483, #5891, #32043, #25252, #38008, #27808, #2282, #25468, #11844, #21844, #28016, #12266, #22261, #15265, #28223, #15683, #38432, #28641, #35234, #5686, #9295, #8447, #8656, #18660, #15474, #21424, #28429, #6095, #38218, #9079, #5119, #21492, #31687, #34670, #23451, #30029, #36629, #8527, #15127, #4031, #39103, #32312, #41681, #19543, #29314, #9564, #186, #26153, #15734, #9984, #35716, #3584, #12536, #6578, #13166, #16168, #12959, #19754, #3179, #22521, #35505, #32515, #25940, #38904, #9132, #22946, #9782, #35914, #12749, #19132, #29107, #31882, #6153, #22314, #6781, #18915, #2751, #25521, #42106, #35081, #32720, #35291, #16579, #3384, #6363, #16371, #28689, #38486, #9348, #29533, #12321, #32097, #19338, #2964, #25304, #38267, #15955, #28904, #22109, #41901, #25729, #5941, #38692, #3801, #400, #14020, #13374, #36554, #26991, #36341, #36122, #23804, #26356, #32937, #26783, #39954, #16785, #39307, #33584, #33358, #7851, #17627 ),
 ( #4008, #829, #6994, #11034, #23595, #29743, #10186, #39525, #7420, #13803, #607, #39748, #16993, #13582, #26566, #10402, #23378, #7213, #20184, #24018, #23155, #4445, #10615, #33145, #27202, #20394, #1047, #20821, #4226, #30383, #17208, #30171, #10818, #17425, #36768, #7631, #19970, #14223, #36990, #20605, #1253, #40167, #33793, #4648, #21228, #24428, #21636, #33997, #11853, #37396, #2289, #2075, #40790, #24852, #18455, #34199, #12061, #21850, #31423, #21436, #14650, #8252, #25053, #24639, #17829, #5059, #5269, #11241, #37602, #28024, #38015, #8047, #15273, #18038, #5479, #28232, #11643, #18242, #31214, #15059, #1663, #41218, #8879, #34826, #4851, #34614, #31014, #1868, #14848, #37809, #41003, #27818, #8664, #8458, #27410, #34409, #40581, #21021, #5693, #30593, #1461, #14436, #40380, #24223, #37193, #30803, #27613, #11437, #31632, #9734, #25478, #2498, #35038, #5899, #9945, #31838, #25892, #32051, #15693, #25259, #32268, #38226, #35867, #15483, #32472, #38857, #22903, #16125, #2920, #18669, #38442, #3336, #2707, #15909, #18873, #3134, #13121, #9304, #22269, #22694, #16324, #35672, #26103, #35242, #6535, #28437, #28649, #28856, #12492, #41426, #25685, #19501, #41856, #19084, #6104, #12707, #42059, #35457, #38647, #12914, #9514, #12275, #22476, #41640, #9088, #6318, #19293, #29266, #29065, #138, #39061, #22067, #10139, #10351, #10565, #19706, #39903, #13530, #32675, #23107, #36075, #40112, #19919, #13963, #20132, #3749, #13329, #20339, #26312, #23968, #3536, #20553, #26942, #10981, #4172, #33093, #6732, #26518, #33529, #32884, #3960, #6943, #33306, #1202, #39477, #23327, #10766, #4391, #23749, #14168, #36288, #36715, #16531, #16734, #16940, #560, #29481, #13753, #7579, #29908, #7162, #7366, #27145, #778, #17369, #29697, #26732, #39692, #30330, #23545, #36505, #39259, #351, #17155, #30119, #995, #17989, #8618, #18197, #27570, #30753, #27972, #40331, #31165, #1617, #21591, #8406, #5008, #2025, #24801, #40537, #18405, #28182, #37763, #27767, #20971, #14596, #31375, #30966, #24178, #11393, #11593, #17575, #1823, #34363, #2239, #14382, #34565, #24378, #11805, #5427, #14802, #24588, #37552, #21384, #8000, #15220, #41169, #12015, #11194, #40952, #37347, #36935, #37148, #15008, #8201, #7797, #5221, #40737, #20772, #33742, #21174, #4596, #30539, #1408, #27358, #33944, #34150, #4803, #17782, #12225, #41588, #41804, #5643, #32004, #23000, #20027, #2451, #26409, #12444, #453, #13424, #6057, #12658, #25637, #38598, #38175, #10240, #32991, #39362, #41376, #29589, #25427, #38391, #28601, #6833, #9463, #9253, #19806, #35191, #21804 ),
 ( #23209, #19035, #36176, #7047, #28390, #3859, #35969, #16838, #25213, #32775, #29800, #28807, #3641, #665, #2870, #15861, #16630, #25007, #37969, #8830, #34774, #18619, #31583, #15436, #9039, #31785, #22017, #34990, #18824, #5854, #2657, #15643, #33200, #26835, #1308, #36400, #11290, #36614, #4906, #33643, #23866, #27261, #20239, #4064, #30012, #24275, #30439, #17049, #36830, #23651, #14281, #13638, #7478, #20452, #23435, #13856, #39806, #40222, #885, #10670, #26621, #11093, #39581, #7691, #24077, #33418, #7266, #37043, #10456, #4283, #10881, #17265, #30228, #20664, #4702, #4497, #14075, #7903, #21077, #1103, #1515, #27048, #40010, #17479, #17682, #20872, #33842, #30650, #27465, #37245, #14494, #40431, #8099, #34050, #17887, #30860, #37654, #34880, #5115, #25107, #8512, #15535, #15331, #11907, #38071, #31683, #34460, #25314, #35090, #2551, #34666, #27866, #21488, #38276, #37861, #31065, #18293, #18507, #24482, #8719, #41269, #9142, #21285, #28489, #31266, #18724, #41482, #24902, #31477, #2344, #28284, #14897, #12330, #22118, #5951, #18095, #5747, #2129, #15113, #5320, #8929, #12113, #28076, #21900, #41056, #40632, #21692, #11694, #34255, #5534, #18924, #1722, #14703, #27661, #11491, #37451, #1917, #8306, #40842, #24693, #22954, #38703, #2760, #6163, #19140, #23165, #2973, #39113, #3188, #28912, #38494, #3392, #9357, #7002, #15745, #3594, #9992, #36130, #29324, #16175, #31892, #9573, #16587, #15963, #29115, #32108, #16380, #26364, #22531, #35514, #35922, #29543, #6788, #39315, #6374, #19763, #41690, #41909, #25949, #12757, #19346, #25738, #408, #22749, #193, #13175, #32320, #42114, #25530, #13384, #12969, #22323, #28697, #38913, #9791, #35724, #35299, #6586, #19551, #32523, #26161, #32729, #10195, #12544, #3812, #23389, #19981, #36352, #13591, #29754, #32945, #26575, #16793, #615, #39535, #10412, #31724, #1765, #38321, #11954, #27913, #11532, #2592, #37908, #5163, #25152, #34922, #15156, #5792, #15577, #21326, #28536, #28328, #9185, #18137, #41314, #18766, #21738, #18552, #25364, #8764, #28120, #41105, #12161, #31521, #2390, #14746, #41526, #15380, #12377, #18340, #24737, #34712, #37492, #11742, #40886, #22163, #24524, #8347, #31107, #5579, #40674, #35132, #37702, #17929, #38117, #24948, #8975, #34300, #1961, #14945, #30905, #21947, #8559, #27703, #21536, #34504, #5362, #31314, #2172, #15790, #6206, #19180, #6622, #12589, #9400, #5995, #19585, #18969, #27, #32557, #41946, #41734, #29363, #31936, #38534, #32359, #3424, #22363, #2808, #39148, #38954, #13415, #23200, #9614, #35340, #39350, #16417, #3223, #28738, #25776 ) ),
 .UNSPECIFIED., .T., .F., .F. ) 
 B_SPLINE_SURFACE_WITH_KNOTS ( ( 4, 3, 4 ),
 ( 3, 2, 2, 2, 2, 2, 2, 2, 2, 2, 2, 2, 2, 2, 2, 2, 2, 2, 2, 2, 2, 2, 2, 2, 2, 2, 2, 2, 2, 2, 2, 2, 2, 2, 2, 2, 2, 2, 2, 2, 2, 2, 2, 2, 2, 2, 2, 2, 2, 2, 2, 2, 2, 2, 2, 2, 2, 2, 2, 2, 2, 2, 2, 2, 2, 2, 2, 2, 2, 2, 2, 2, 2, 2, 2, 2, 2, 2, 2, 2, 2, 2, 2, 2, 2, 2, 2, 2, 2, 2, 2, 2, 2, 2, 2, 2, 2, 2, 2, 2, 2, 2, 2, 2, 2, 2, 2, 2, 2, 2, 2, 2, 2, 2, 2, 2, 2, 2, 2, 2, 2, 2, 2, 2, 2, 2, 2, 2, 2, 2, 2, 2, 2, 2, 2, 2, 2, 2, 2, 2, 2, 2, 2, 2, 2, 2, 2, 2, 2, 2, 2, 2, 2, 2, 2, 2, 2, 2, 2, 2, 2, 2, 2, 2, 2, 3 ),
 ( 0.000000000000000000, 0.5000000000000000000, 1.000000000000000000 ),
 ( 0.000000000000000000, 0.005882352941176470507, 0.01176470588235294101, 0.01764705882352941152, 0.02352941176470588203, 0.02941176470588235253, 0.03529411764705882304, 0.04117647058823529355, 0.04705882352941176405, 0.05294117647058823456, 0.05882352941176470507, 0.06470588235294118251, 0.07058823529411764608, 0.07647058823529412352, 0.08235294117647058709, 0.08823529411764706454, 0.09411764705882352811, 0.1000000000000000056, 0.1058823529411764691, 0.1117647058823529466, 0.1176470588235294101, 0.1235294117647058876, 0.1294117647058823650, 0.1352941176470588147, 0.1411764705882352922, 0.1470588235294117696, 0.1529411764705882470, 0.1588235294117646967, 0.1647058823529411742, 0.1705882352941176516, 0.1764705882352941291, 0.1823529411764705788, 0.1882352941176470562, 0.1941176470588235337, 0.2000000000000000111, 0.2058823529411764608, 0.2117647058823529382, 0.2176470588235294157, 0.2235294117647058931, 0.2294117647058823428, 0.2352941176470588203, 0.2411764705882352977, 0.2470588235294117752, 0.2529411764705882248, 0.2588235294117647300, 0.2647058823529411797, 0.2705882352941176294, 0.2764705882352941346, 0.2823529411764705843, 0.2882352941176470340, 0.2941176470588235392, 0.2999999999999999889, 0.3058823529411764941, 0.3117647058823529438, 0.3176470588235293935, 0.3235294117647058987, 0.3294117647058823484, 0.3352941176470587981, 0.3411764705882353033, 0.3470588235294117530, 0.3529411764705882582, 0.3588235294117647078, 0.3647058823529411575, 0.3705882352941176627, 0.3764705882352941124, 0.3823529411764705621, 0.3882352941176470673, 0.3941176470588235170, 0.4000000000000000222, 0.4058823529411764719, 0.4117647058823529216, 0.4176470588235294268, 0.4235294117647058765, 0.4294117647058823262, 0.4352941176470588314, 0.4411764705882352811, 0.4470588235294117863, 0.4529411764705882359, 0.4588235294117646856, 0.4647058823529411908, 0.4705882352941176405, 0.4764705882352940902, 0.4823529411764705954, 0.4882352941176470451, 0.4941176470588235503, 0.5000000000000000000, 0.5058823529411764497, 0.5117647058823528994, 0.5176470588235294601, 0.5235294117647059098, 0.5294117647058823595, 0.5352941176470588092, 0.5411764705882352589, 0.5470588235294118196, 0.5529411764705882693, 0.5588235294117647189, 0.5647058823529411686, 0.5705882352941176183, 0.5764705882352940680, 0.5823529411764706287, 0.5882352941176470784, 0.5941176470588235281, 0.5999999999999999778, 0.6058823529411764275, 0.6117647058823529882, 0.6176470588235294379, 0.6235294117647058876, 0.6294117647058823373, 0.6352941176470587870, 0.6411764705882353477, 0.6470588235294117974, 0.6529411764705882470, 0.6588235294117646967, 0.6647058823529411464, 0.6705882352941175961, 0.6764705882352941568, 0.6823529411764706065, 0.6882352941176470562, 0.6941176470588235059, 0.6999999999999999556, 0.7058823529411765163, 0.7117647058823529660, 0.7176470588235294157, 0.7235294117647058654, 0.7294117647058823151, 0.7352941176470588758, 0.7411764705882353255, 0.7470588235294117752, 0.7529411764705882248, 0.7588235294117646745, 0.7647058823529411242, 0.7705882352941176849, 0.7764705882352941346, 0.7823529411764705843, 0.7882352941176470340, 0.7941176470588234837, 0.8000000000000000444, 0.8058823529411764941, 0.8117647058823529438, 0.8176470588235293935, 0.8235294117647058432, 0.8294117647058824039, 0.8352941176470588536, 0.8411764705882353033, 0.8470588235294117530, 0.8529411764705882026, 0.8588235294117646523, 0.8647058823529412130, 0.8705882352941176627, 0.8764705882352941124, 0.8823529411764705621, 0.8882352941176470118, 0.8941176470588235725, 0.9000000000000000222, 0.9058823529411764719, 0.9117647058823529216, 0.9176470588235293713, 0.9235294117647059320, 0.9294117647058823817, 0.9352941176470588314, 0.9411764705882352811, 0.9470588235294117307, 0.9529411764705881804, 0.9588235294117647411, 0.9647058823529411908, 0.9705882352941176405 ),
 .UNSPECIFIED. ) 
 GEOMETRIC_REPRESENTATION_ITEM ( )  RATIONAL_B_SPLINE_SURFACE ( (
 ( 1.000000000000000000, 0.9510565162951535312, 1.000000000000000000, 0.9510565162951535312, 1.000000000000000000, 0.9510565162951535312, 1.000000000000000000, 0.9510565162951535312, 1.000000000000000000, 0.9510565162951535312, 1.000000000000000000, 0.9510565162951535312, 1.000000000000000000, 0.9510565162951535312, 1.000000000000000000, 0.9510565162951535312, 1.000000000000000000, 0.9510565162951535312, 1.000000000000000000, 0.9510565162951535312, 1.000000000000000000, 0.9510565162951535312, 1.000000000000000000, 0.9510565162951535312, 1.000000000000000000, 0.9510565162951535312, 1.000000000000000000, 0.9510565162951535312, 1.000000000000000000, 0.9510565162951535312, 1.000000000000000000, 0.9510565162951535312, 1.000000000000000000, 0.9510565162951535312, 1.000000000000000000, 0.9510565162951535312, 1.000000000000000000, 0.9510565162951535312, 1.000000000000000000, 0.9510565162951535312, 1.000000000000000000, 0.9510565162951535312, 1.000000000000000000, 0.9510565162951535312, 1.000000000000000000, 0.9510565162951535312, 1.000000000000000000, 0.9510565162951535312, 1.000000000000000000, 0.9510565162951535312, 1.000000000000000000, 0.9510565162951535312, 1.000000000000000000, 0.9510565162951535312, 1.000000000000000000, 0.9510565162951535312, 1.000000000000000000, 0.9510565162951535312, 1.000000000000000000, 0.9510565162951535312, 1.000000000000000000, 0.9510565162951535312, 1.000000000000000000, 0.9510565162951535312, 1.000000000000000000, 0.9510565162951535312, 1.000000000000000000, 0.9510565162951535312, 1.000000000000000000, 0.9510565162951535312, 1.000000000000000000, 0.9510565162951535312, 1.000000000000000000, 0.9510565162951535312, 1.000000000000000000, 0.9510565162951535312, 1.000000000000000000, 0.9510565162951535312, 1.000000000000000000, 0.9510565162951535312, 1.000000000000000000, 0.9510565162951535312, 1.000000000000000000, 0.9510565162951535312, 1.000000000000000000, 0.9510565162951535312, 1.000000000000000000, 0.9510565162951535312, 1.000000000000000000, 0.9510565162951535312, 1.000000000000000000, 0.9510565162951535312, 1.000000000000000000, 0.9510565162951535312, 1.000000000000000000, 0.9510565162951535312, 1.000000000000000000, 0.9510565162951535312, 1.000000000000000000, 0.9510565162951535312, 1.000000000000000000, 0.9510565162951535312, 1.000000000000000000, 0.9510565162951535312, 1.000000000000000000, 0.9510565162951535312, 1.000000000000000000, 0.9510565162951535312, 1.000000000000000000, 0.9510565162951535312, 1.000000000000000000, 0.9510565162951535312, 1.000000000000000000, 0.9510565162951535312, 1.000000000000000000, 0.9510565162951535312, 1.000000000000000000, 0.9510565162951535312, 1.000000000000000000, 0.9510565162951535312, 1.000000000000000000, 0.9510565162951535312, 1.000000000000000000, 0.9510565162951535312, 1.000000000000000000, 0.9510565162951535312, 1.000000000000000000, 0.9510565162951535312, 1.000000000000000000, 0.9510565162951535312, 1.000000000000000000, 0.9510565162951535312, 1.000000000000000000, 0.9510565162951535312, 1.000000000000000000, 0.9510565162951535312, 1.000000000000000000, 0.9510565162951535312, 1.000000000000000000, 0.9510565162951535312, 1.000000000000000000, 0.9510565162951535312, 1.000000000000000000, 0.9510565162951535312, 1.000000000000000000, 0.9510565162951535312, 1.000000000000000000, 0.9510565162951535312, 1.000000000000000000, 0.9510565162951535312, 1.000000000000000000, 0.9510565162951535312, 1.000000000000000000, 0.9510565162951535312, 1.000000000000000000, 0.9510565162951535312, 1.000000000000000000, 0.9510565162951535312, 1.000000000000000000, 0.9510565162951535312, 1.000000000000000000, 0.9510565162951535312, 1.000000000000000000, 0.9510565162951535312, 1.000000000000000000, 0.9510565162951535312, 1.000000000000000000, 0.9510565162951535312, 1.000000000000000000, 0.9510565162951535312, 1.000000000000000000, 0.9510565162951535312, 1.000000000000000000, 0.9510565162951535312, 1.000000000000000000, 0.9510565162951535312, 1.000000000000000000, 0.9510565162951535312, 1.000000000000000000, 0.9510565162951535312, 1.000000000000000000, 0.9510565162951535312, 1.000000000000000000, 0.9510565162951535312, 1.000000000000000000, 0.9510565162951535312, 1.000000000000000000, 0.9510565162951535312, 1.000000000000000000, 0.9510565162951535312, 1.000000000000000000, 0.9510565162951535312, 1.000000000000000000, 0.9510565162951535312, 1.000000000000000000, 0.9510565162951535312, 1.000000000000000000, 0.9510565162951535312, 1.000000000000000000, 0.9510565162951535312, 1.000000000000000000, 0.9510565162951535312, 1.000000000000000000, 0.9510565162951535312, 1.000000000000000000, 0.9510565162951535312, 1.000000000000000000, 0.9510565162951535312, 1.000000000000000000, 0.9510565162951535312, 1.000000000000000000, 0.9510565162951535312, 1.000000000000000000, 0.9510565162951535312, 1.000000000000000000, 0.9510565162951535312, 1.000000000000000000, 0.9510565162951535312, 1.000000000000000000, 0.9510565162951535312, 1.000000000000000000, 0.9510565162951535312, 1.000000000000000000, 0.9510565162951535312, 1.000000000000000000, 0.9510565162951535312, 1.000000000000000000, 0.9510565162951535312, 1.000000000000000000, 0.9510565162951535312, 1.000000000000000000, 0.9510565162951535312, 1.000000000000000000, 0.9510565162951535312, 1.000000000000000000, 0.9510565162951535312, 1.000000000000000000, 0.9510565162951535312, 1.000000000000000000, 0.9510565162951535312, 1.000000000000000000, 0.9510565162951535312, 1.000000000000000000, 0.9510565162951535312, 1.000000000000000000, 0.9510565162951535312, 1.000000000000000000, 0.9510565162951535312, 1.000000000000000000, 0.9510565162951535312, 1.000000000000000000, 0.9510565162951535312, 1.000000000000000000, 0.9510565162951535312, 1.000000000000000000, 0.9510565162951535312, 1.000000000000000000, 0.9510565162951535312, 1.000000000000000000, 0.9510565162951535312, 1.000000000000000000, 0.9510565162951535312, 1.000000000000000000, 0.9510565162951535312, 1.000000000000000000, 0.9510565162951535312, 1.000000000000000000, 0.9510565162951535312, 1.000000000000000000, 0.9510565162951535312, 1.000000000000000000, 0.9510565162951535312, 1.000000000000000000, 0.9510565162951535312, 1.000000000000000000, 0.9510565162951535312, 1.000000000000000000, 0.9510565162951535312, 1.000000000000000000, 0.9510565162951535312, 1.000000000000000000, 0.9510565162951535312, 1.000000000000000000, 0.9510565162951535312, 1.000000000000000000, 0.9510565162951535312, 1.000000000000000000, 0.9510565162951535312, 1.000000000000000000, 0.9510565162951535312, 1.000000000000000000, 0.9510565162951535312, 1.000000000000000000, 0.9510565162951535312, 1.000000000000000000, 0.9510565162951535312, 1.000000000000000000, 0.9510565162951535312, 1.000000000000000000, 0.9510565162951535312, 1.000000000000000000, 0.9510565162951535312, 1.000000000000000000, 0.9510565162951535312, 1.000000000000000000, 0.9510565162951535312, 1.000000000000000000, 0.9510565162951535312, 1.000000000000000000, 0.9510565162951535312, 1.000000000000000000, 0.9510565162951535312, 1.000000000000000000, 0.9510565162951535312, 1.000000000000000000, 0.9510565162951535312, 1.000000000000000000, 0.9510565162951535312, 1.000000000000000000, 0.9510565162951535312, 1.000000000000000000, 0.9510565162951535312, 1.000000000000000000, 0.9510565162951535312, 1.000000000000000000, 0.9510565162951535312, 1.000000000000000000, 0.9510565162951535312, 1.000000000000000000, 0.9510565162951535312, 1.000000000000000000),
 ( 0.3333333333333333703, 0.3170188387650512141, 0.3333333333333333703, 0.3170188387650512141, 0.3333333333333333703, 0.3170188387650512141, 0.3333333333333333703, 0.3170188387650512141, 0.3333333333333333703, 0.3170188387650512141, 0.3333333333333333703, 0.3170188387650512141, 0.3333333333333333703, 0.3170188387650512141, 0.3333333333333333703, 0.3170188387650512141, 0.3333333333333333703, 0.3170188387650512141, 0.3333333333333333703, 0.3170188387650512141, 0.3333333333333333703, 0.3170188387650512141, 0.3333333333333333703, 0.3170188387650512141, 0.3333333333333333703, 0.3170188387650512141, 0.3333333333333333703, 0.3170188387650512141, 0.3333333333333333703, 0.3170188387650512141, 0.3333333333333333703, 0.3170188387650512141, 0.3333333333333333703, 0.3170188387650512141, 0.3333333333333333703, 0.3170188387650512141, 0.3333333333333333703, 0.3170188387650512141, 0.3333333333333333703, 0.3170188387650512141, 0.3333333333333333703, 0.3170188387650512141, 0.3333333333333333703, 0.3170188387650512141, 0.3333333333333333703, 0.3170188387650512141, 0.3333333333333333703, 0.3170188387650512141, 0.3333333333333333703, 0.3170188387650512141, 0.3333333333333333703, 0.3170188387650512141, 0.3333333333333333703, 0.3170188387650512141, 0.3333333333333333703, 0.3170188387650512141, 0.3333333333333333703, 0.3170188387650512141, 0.3333333333333333703, 0.3170188387650512141, 0.3333333333333333703, 0.3170188387650512141, 0.3333333333333333703, 0.3170188387650512141, 0.3333333333333333703, 0.3170188387650512141, 0.3333333333333333703, 0.3170188387650512141, 0.3333333333333333703, 0.3170188387650512141, 0.3333333333333333703, 0.3170188387650512141, 0.3333333333333333703, 0.3170188387650512141, 0.3333333333333333703, 0.3170188387650512141, 0.3333333333333333703, 0.3170188387650512141, 0.3333333333333333703, 0.3170188387650512141, 0.3333333333333333703, 0.3170188387650512141, 0.3333333333333333703, 0.3170188387650512141, 0.3333333333333333703, 0.3170188387650512141, 0.3333333333333333703, 0.3170188387650512141, 0.3333333333333333703, 0.3170188387650512141, 0.3333333333333333703, 0.3170188387650512141, 0.3333333333333333703, 0.3170188387650512141, 0.3333333333333333703, 0.3170188387650512141, 0.3333333333333333703, 0.3170188387650512141, 0.3333333333333333703, 0.3170188387650512141, 0.3333333333333333703, 0.3170188387650512141, 0.3333333333333333703, 0.3170188387650512141, 0.3333333333333333703, 0.3170188387650512141, 0.3333333333333333703, 0.3170188387650512141, 0.3333333333333333703, 0.3170188387650512141, 0.3333333333333333703, 0.3170188387650512141, 0.3333333333333333703, 0.3170188387650512141, 0.3333333333333333703, 0.3170188387650512141, 0.3333333333333333703, 0.3170188387650512141, 0.3333333333333333703, 0.3170188387650512141, 0.3333333333333333703, 0.3170188387650512141, 0.3333333333333333703, 0.3170188387650512141, 0.3333333333333333703, 0.3170188387650512141, 0.3333333333333333703, 0.3170188387650512141, 0.3333333333333333703, 0.3170188387650512141, 0.3333333333333333703, 0.3170188387650512141, 0.3333333333333333703, 0.3170188387650512141, 0.3333333333333333703, 0.3170188387650512141, 0.3333333333333333703, 0.3170188387650512141, 0.3333333333333333703, 0.3170188387650512141, 0.3333333333333333703, 0.3170188387650512141, 0.3333333333333333703, 0.3170188387650512141, 0.3333333333333333703, 0.3170188387650512141, 0.3333333333333333703, 0.3170188387650512141, 0.3333333333333333703, 0.3170188387650512141, 0.3333333333333333703, 0.3170188387650512141, 0.3333333333333333703, 0.3170188387650512141, 0.3333333333333333703, 0.3170188387650512141, 0.3333333333333333703, 0.3170188387650512141, 0.3333333333333333703, 0.3170188387650512141, 0.3333333333333333703, 0.3170188387650512141, 0.3333333333333333703, 0.3170188387650512141, 0.3333333333333333703, 0.3170188387650512141, 0.3333333333333333703, 0.3170188387650512141, 0.3333333333333333703, 0.3170188387650512141, 0.3333333333333333703, 0.3170188387650512141, 0.3333333333333333703, 0.3170188387650512141, 0.3333333333333333703, 0.3170188387650512141, 0.3333333333333333703, 0.3170188387650512141, 0.3333333333333333703, 0.3170188387650512141, 0.3333333333333333703, 0.3170188387650512141, 0.3333333333333333703, 0.3170188387650512141, 0.3333333333333333703, 0.3170188387650512141, 0.3333333333333333703, 0.3170188387650512141, 0.3333333333333333703, 0.3170188387650512141, 0.3333333333333333703, 0.3170188387650512141, 0.3333333333333333703, 0.3170188387650512141, 0.3333333333333333703, 0.3170188387650512141, 0.3333333333333333703, 0.3170188387650512141, 0.3333333333333333703, 0.3170188387650512141, 0.3333333333333333703, 0.3170188387650512141, 0.3333333333333333703, 0.3170188387650512141, 0.3333333333333333703, 0.3170188387650512141, 0.3333333333333333703, 0.3170188387650512141, 0.3333333333333333703, 0.3170188387650512141, 0.3333333333333333703, 0.3170188387650512141, 0.3333333333333333703, 0.3170188387650512141, 0.3333333333333333703, 0.3170188387650512141, 0.3333333333333333703, 0.3170188387650512141, 0.3333333333333333703, 0.3170188387650512141, 0.3333333333333333703, 0.3170188387650512141, 0.3333333333333333703, 0.3170188387650512141, 0.3333333333333333703, 0.3170188387650512141, 0.3333333333333333703, 0.3170188387650512141, 0.3333333333333333703, 0.3170188387650512141, 0.3333333333333333703, 0.3170188387650512141, 0.3333333333333333703, 0.3170188387650512141, 0.3333333333333333703, 0.3170188387650512141, 0.3333333333333333703, 0.3170188387650512141, 0.3333333333333333703, 0.3170188387650512141, 0.3333333333333333703, 0.3170188387650512141, 0.3333333333333333703, 0.3170188387650512141, 0.3333333333333333703, 0.3170188387650512141, 0.3333333333333333703, 0.3170188387650512141, 0.3333333333333333703, 0.3170188387650512141, 0.3333333333333333703, 0.3170188387650512141, 0.3333333333333333703, 0.3170188387650512141, 0.3333333333333333703, 0.3170188387650512141, 0.3333333333333333703, 0.3170188387650512141, 0.3333333333333333703, 0.3170188387650512141, 0.3333333333333333703, 0.3170188387650512141, 0.3333333333333333703, 0.3170188387650512141, 0.3333333333333333703, 0.3170188387650512141, 0.3333333333333333703, 0.3170188387650512141, 0.3333333333333333703, 0.3170188387650512141, 0.3333333333333333703, 0.3170188387650512141, 0.3333333333333333703, 0.3170188387650512141, 0.3333333333333333703, 0.3170188387650512141, 0.3333333333333333703, 0.3170188387650512141, 0.3333333333333333703, 0.3170188387650512141, 0.3333333333333333703, 0.3170188387650512141, 0.3333333333333333703, 0.3170188387650512141, 0.3333333333333333703, 0.3170188387650512141, 0.3333333333333333703, 0.3170188387650512141, 0.3333333333333333703, 0.3170188387650512141, 0.3333333333333333703, 0.3170188387650512141, 0.3333333333333333703, 0.3170188387650512141, 0.3333333333333333703, 0.3170188387650512141, 0.3333333333333333703, 0.3170188387650512141, 0.3333333333333333703, 0.3170188387650512141, 0.3333333333333333703, 0.3170188387650512141, 0.3333333333333333703, 0.3170188387650512141, 0.3333333333333333703, 0.3170188387650512141, 0.3333333333333333703, 0.3170188387650512141, 0.3333333333333333703, 0.3170188387650512141, 0.3333333333333333703, 0.3170188387650512141, 0.3333333333333333703, 0.3170188387650512141, 0.3333333333333333703, 0.3170188387650512141, 0.3333333333333333703, 0.3170188387650512141, 0.3333333333333333703, 0.3170188387650512141, 0.3333333333333333703, 0.3170188387650512141, 0.3333333333333333703, 0.3170188387650512141, 0.3333333333333333703, 0.3170188387650512141, 0.3333333333333333703, 0.3170188387650512141, 0.3333333333333333703, 0.3170188387650512141, 0.3333333333333333703),
 ( 0.3333333333333333703, 0.3170188387650512141, 0.3333333333333333703, 0.3170188387650512141, 0.3333333333333333703, 0.3170188387650512141, 0.3333333333333333703, 0.3170188387650512141, 0.3333333333333333703, 0.3170188387650512141, 0.3333333333333333703, 0.3170188387650512141, 0.3333333333333333703, 0.3170188387650512141, 0.3333333333333333703, 0.3170188387650512141, 0.3333333333333333703, 0.3170188387650512141, 0.3333333333333333703, 0.3170188387650512141, 0.3333333333333333703, 0.3170188387650512141, 0.3333333333333333703, 0.3170188387650512141, 0.3333333333333333703, 0.3170188387650512141, 0.3333333333333333703, 0.3170188387650512141, 0.3333333333333333703, 0.3170188387650512141, 0.3333333333333333703, 0.3170188387650512141, 0.3333333333333333703, 0.3170188387650512141, 0.3333333333333333703, 0.3170188387650512141, 0.3333333333333333703, 0.3170188387650512141, 0.3333333333333333703, 0.3170188387650512141, 0.3333333333333333703, 0.3170188387650512141, 0.3333333333333333703, 0.3170188387650512141, 0.3333333333333333703, 0.3170188387650512141, 0.3333333333333333703, 0.3170188387650512141, 0.3333333333333333703, 0.3170188387650512141, 0.3333333333333333703, 0.3170188387650512141, 0.3333333333333333703, 0.3170188387650512141, 0.3333333333333333703, 0.3170188387650512141, 0.3333333333333333703, 0.3170188387650512141, 0.3333333333333333703, 0.3170188387650512141, 0.3333333333333333703, 0.3170188387650512141, 0.3333333333333333703, 0.3170188387650512141, 0.3333333333333333703, 0.3170188387650512141, 0.3333333333333333703, 0.3170188387650512141, 0.3333333333333333703, 0.3170188387650512141, 0.3333333333333333703, 0.3170188387650512141, 0.3333333333333333703, 0.3170188387650512141, 0.3333333333333333703, 0.3170188387650512141, 0.3333333333333333703, 0.3170188387650512141, 0.3333333333333333703, 0.3170188387650512141, 0.3333333333333333703, 0.3170188387650512141, 0.3333333333333333703, 0.3170188387650512141, 0.3333333333333333703, 0.3170188387650512141, 0.3333333333333333703, 0.3170188387650512141, 0.3333333333333333703, 0.3170188387650512141, 0.3333333333333333703, 0.3170188387650512141, 0.3333333333333333703, 0.3170188387650512141, 0.3333333333333333703, 0.3170188387650512141, 0.3333333333333333703, 0.3170188387650512141, 0.3333333333333333703, 0.3170188387650512141, 0.3333333333333333703, 0.3170188387650512141, 0.3333333333333333703, 0.3170188387650512141, 0.3333333333333333703, 0.3170188387650512141, 0.3333333333333333703, 0.3170188387650512141, 0.3333333333333333703, 0.3170188387650512141, 0.3333333333333333703, 0.3170188387650512141, 0.3333333333333333703, 0.3170188387650512141, 0.3333333333333333703, 0.3170188387650512141, 0.3333333333333333703, 0.3170188387650512141, 0.3333333333333333703, 0.3170188387650512141, 0.3333333333333333703, 0.3170188387650512141, 0.3333333333333333703, 0.3170188387650512141, 0.3333333333333333703, 0.3170188387650512141, 0.3333333333333333703, 0.3170188387650512141, 0.3333333333333333703, 0.3170188387650512141, 0.3333333333333333703, 0.3170188387650512141, 0.3333333333333333703, 0.3170188387650512141, 0.3333333333333333703, 0.3170188387650512141, 0.3333333333333333703, 0.3170188387650512141, 0.3333333333333333703, 0.3170188387650512141, 0.3333333333333333703, 0.3170188387650512141, 0.3333333333333333703, 0.3170188387650512141, 0.3333333333333333703, 0.3170188387650512141, 0.3333333333333333703, 0.3170188387650512141, 0.3333333333333333703, 0.3170188387650512141, 0.3333333333333333703, 0.3170188387650512141, 0.3333333333333333703, 0.3170188387650512141, 0.3333333333333333703, 0.3170188387650512141, 0.3333333333333333703, 0.3170188387650512141, 0.3333333333333333703, 0.3170188387650512141, 0.3333333333333333703, 0.3170188387650512141, 0.3333333333333333703, 0.3170188387650512141, 0.3333333333333333703, 0.3170188387650512141, 0.3333333333333333703, 0.3170188387650512141, 0.3333333333333333703, 0.3170188387650512141, 0.3333333333333333703, 0.3170188387650512141, 0.3333333333333333703, 0.3170188387650512141, 0.3333333333333333703, 0.3170188387650512141, 0.3333333333333333703, 0.3170188387650512141, 0.3333333333333333703, 0.3170188387650512141, 0.3333333333333333703, 0.3170188387650512141, 0.3333333333333333703, 0.3170188387650512141, 0.3333333333333333703, 0.3170188387650512141, 0.3333333333333333703, 0.3170188387650512141, 0.3333333333333333703, 0.3170188387650512141, 0.3333333333333333703, 0.3170188387650512141, 0.3333333333333333703, 0.3170188387650512141, 0.3333333333333333703, 0.3170188387650512141, 0.3333333333333333703, 0.3170188387650512141, 0.3333333333333333703, 0.3170188387650512141, 0.3333333333333333703, 0.3170188387650512141, 0.3333333333333333703, 0.3170188387650512141, 0.3333333333333333703, 0.3170188387650512141, 0.3333333333333333703, 0.3170188387650512141, 0.3333333333333333703, 0.3170188387650512141, 0.3333333333333333703, 0.3170188387650512141, 0.3333333333333333703, 0.3170188387650512141, 0.3333333333333333703, 0.3170188387650512141, 0.3333333333333333703, 0.3170188387650512141, 0.3333333333333333703, 0.3170188387650512141, 0.3333333333333333703, 0.3170188387650512141, 0.3333333333333333703, 0.3170188387650512141, 0.3333333333333333703, 0.3170188387650512141, 0.3333333333333333703, 0.3170188387650512141, 0.3333333333333333703, 0.3170188387650512141, 0.3333333333333333703, 0.3170188387650512141, 0.3333333333333333703, 0.3170188387650512141, 0.3333333333333333703, 0.3170188387650512141, 0.3333333333333333703, 0.3170188387650512141, 0.3333333333333333703, 0.3170188387650512141, 0.3333333333333333703, 0.3170188387650512141, 0.3333333333333333703, 0.3170188387650512141, 0.3333333333333333703, 0.3170188387650512141, 0.3333333333333333703, 0.3170188387650512141, 0.3333333333333333703, 0.3170188387650512141, 0.3333333333333333703, 0.3170188387650512141, 0.3333333333333333703, 0.3170188387650512141, 0.3333333333333333703, 0.3170188387650512141, 0.3333333333333333703, 0.3170188387650512141, 0.3333333333333333703, 0.3170188387650512141, 0.3333333333333333703, 0.3170188387650512141, 0.3333333333333333703, 0.3170188387650512141, 0.3333333333333333703, 0.3170188387650512141, 0.3333333333333333703, 0.3170188387650512141, 0.3333333333333333703, 0.3170188387650512141, 0.3333333333333333703, 0.3170188387650512141, 0.3333333333333333703, 0.3170188387650512141, 0.3333333333333333703, 0.3170188387650512141, 0.3333333333333333703, 0.3170188387650512141, 0.3333333333333333703, 0.3170188387650512141, 0.3333333333333333703, 0.3170188387650512141, 0.3333333333333333703, 0.3170188387650512141, 0.3333333333333333703, 0.3170188387650512141, 0.3333333333333333703, 0.3170188387650512141, 0.3333333333333333703, 0.3170188387650512141, 0.3333333333333333703, 0.3170188387650512141, 0.3333333333333333703, 0.3170188387650512141, 0.3333333333333333703, 0.3170188387650512141, 0.3333333333333333703, 0.3170188387650512141, 0.3333333333333333703, 0.3170188387650512141, 0.3333333333333333703, 0.3170188387650512141, 0.3333333333333333703, 0.3170188387650512141, 0.3333333333333333703, 0.3170188387650512141, 0.3333333333333333703, 0.3170188387650512141, 0.3333333333333333703, 0.3170188387650512141, 0.3333333333333333703, 0.3170188387650512141, 0.3333333333333333703, 0.3170188387650512141, 0.3333333333333333703, 0.3170188387650512141, 0.3333333333333333703, 0.3170188387650512141, 0.3333333333333333703, 0.3170188387650512141, 0.3333333333333333703, 0.3170188387650512141, 0.3333333333333333703, 0.3170188387650512141, 0.3333333333333333703, 0.3170188387650512141, 0.3333333333333333703, 0.3170188387650512141, 0.3333333333333333703, 0.3170188387650512141, 0.3333333333333333703),
 ( 1.000000000000000000, 0.9510565162951535312, 1.000000000000000000, 0.9510565162951535312, 1.000000000000000000, 0.9510565162951535312, 1.000000000000000000, 0.9510565162951535312, 1.000000000000000000, 0.9510565162951535312, 1.000000000000000000, 0.9510565162951535312, 1.000000000000000000, 0.9510565162951535312, 1.000000000000000000, 0.9510565162951535312, 1.000000000000000000, 0.9510565162951535312, 1.000000000000000000, 0.9510565162951535312, 1.000000000000000000, 0.9510565162951535312, 1.000000000000000000, 0.9510565162951535312, 1.000000000000000000, 0.9510565162951535312, 1.000000000000000000, 0.9510565162951535312, 1.000000000000000000, 0.9510565162951535312, 1.000000000000000000, 0.9510565162951535312, 1.000000000000000000, 0.9510565162951535312, 1.000000000000000000, 0.9510565162951535312, 1.000000000000000000, 0.9510565162951535312, 1.000000000000000000, 0.9510565162951535312, 1.000000000000000000, 0.9510565162951535312, 1.000000000000000000, 0.9510565162951535312, 1.000000000000000000, 0.9510565162951535312, 1.000000000000000000, 0.9510565162951535312, 1.000000000000000000, 0.9510565162951535312, 1.000000000000000000, 0.9510565162951535312, 1.000000000000000000, 0.9510565162951535312, 1.000000000000000000, 0.9510565162951535312, 1.000000000000000000, 0.9510565162951535312, 1.000000000000000000, 0.9510565162951535312, 1.000000000000000000, 0.9510565162951535312, 1.000000000000000000, 0.9510565162951535312, 1.000000000000000000, 0.9510565162951535312, 1.000000000000000000, 0.9510565162951535312, 1.000000000000000000, 0.9510565162951535312, 1.000000000000000000, 0.9510565162951535312, 1.000000000000000000, 0.9510565162951535312, 1.000000000000000000, 0.9510565162951535312, 1.000000000000000000, 0.9510565162951535312, 1.000000000000000000, 0.9510565162951535312, 1.000000000000000000, 0.9510565162951535312, 1.000000000000000000, 0.9510565162951535312, 1.000000000000000000, 0.9510565162951535312, 1.000000000000000000, 0.9510565162951535312, 1.000000000000000000, 0.9510565162951535312, 1.000000000000000000, 0.9510565162951535312, 1.000000000000000000, 0.9510565162951535312, 1.000000000000000000, 0.9510565162951535312, 1.000000000000000000, 0.9510565162951535312, 1.000000000000000000, 0.9510565162951535312, 1.000000000000000000, 0.9510565162951535312, 1.000000000000000000, 0.9510565162951535312, 1.000000000000000000, 0.9510565162951535312, 1.000000000000000000, 0.9510565162951535312, 1.000000000000000000, 0.9510565162951535312, 1.000000000000000000, 0.9510565162951535312, 1.000000000000000000, 0.9510565162951535312, 1.000000000000000000, 0.9510565162951535312, 1.000000000000000000, 0.9510565162951535312, 1.000000000000000000, 0.9510565162951535312, 1.000000000000000000, 0.9510565162951535312, 1.000000000000000000, 0.9510565162951535312, 1.000000000000000000, 0.9510565162951535312, 1.000000000000000000, 0.9510565162951535312, 1.000000000000000000, 0.9510565162951535312, 1.000000000000000000, 0.9510565162951535312, 1.000000000000000000, 0.9510565162951535312, 1.000000000000000000, 0.9510565162951535312, 1.000000000000000000, 0.9510565162951535312, 1.000000000000000000, 0.9510565162951535312, 1.000000000000000000, 0.9510565162951535312, 1.000000000000000000, 0.9510565162951535312, 1.000000000000000000, 0.9510565162951535312, 1.000000000000000000, 0.9510565162951535312, 1.000000000000000000, 0.9510565162951535312, 1.000000000000000000, 0.9510565162951535312, 1.000000000000000000, 0.9510565162951535312, 1.000000000000000000, 0.9510565162951535312, 1.000000000000000000, 0.9510565162951535312, 1.000000000000000000, 0.9510565162951535312, 1.000000000000000000, 0.9510565162951535312, 1.000000000000000000, 0.9510565162951535312, 1.000000000000000000, 0.9510565162951535312, 1.000000000000000000, 0.9510565162951535312, 1.000000000000000000, 0.9510565162951535312, 1.000000000000000000, 0.9510565162951535312, 1.000000000000000000, 0.9510565162951535312, 1.000000000000000000, 0.9510565162951535312, 1.000000000000000000, 0.9510565162951535312, 1.000000000000000000, 0.9510565162951535312, 1.000000000000000000, 0.9510565162951535312, 1.000000000000000000, 0.9510565162951535312, 1.000000000000000000, 0.9510565162951535312, 1.000000000000000000, 0.9510565162951535312, 1.000000000000000000, 0.9510565162951535312, 1.000000000000000000, 0.9510565162951535312, 1.000000000000000000, 0.9510565162951535312, 1.000000000000000000, 0.9510565162951535312, 1.000000000000000000, 0.9510565162951535312, 1.000000000000000000, 0.9510565162951535312, 1.000000000000000000, 0.9510565162951535312, 1.000000000000000000, 0.9510565162951535312, 1.000000000000000000, 0.9510565162951535312, 1.000000000000000000, 0.9510565162951535312, 1.000000000000000000, 0.9510565162951535312, 1.000000000000000000, 0.9510565162951535312, 1.000000000000000000, 0.9510565162951535312, 1.000000000000000000, 0.9510565162951535312, 1.000000000000000000, 0.9510565162951535312, 1.000000000000000000, 0.9510565162951535312, 1.000000000000000000, 0.9510565162951535312, 1.000000000000000000, 0.9510565162951535312, 1.000000000000000000, 0.9510565162951535312, 1.000000000000000000, 0.9510565162951535312, 1.000000000000000000, 0.9510565162951535312, 1.000000000000000000, 0.9510565162951535312, 1.000000000000000000, 0.9510565162951535312, 1.000000000000000000, 0.9510565162951535312, 1.000000000000000000, 0.9510565162951535312, 1.000000000000000000, 0.9510565162951535312, 1.000000000000000000, 0.9510565162951535312, 1.000000000000000000, 0.9510565162951535312, 1.000000000000000000, 0.9510565162951535312, 1.000000000000000000, 0.9510565162951535312, 1.000000000000000000, 0.9510565162951535312, 1.000000000000000000, 0.9510565162951535312, 1.000000000000000000, 0.9510565162951535312, 1.000000000000000000, 0.9510565162951535312, 1.000000000000000000, 0.9510565162951535312, 1.000000000000000000, 0.9510565162951535312, 1.000000000000000000, 0.9510565162951535312, 1.000000000000000000, 0.9510565162951535312, 1.000000000000000000, 0.9510565162951535312, 1.000000000000000000, 0.9510565162951535312, 1.000000000000000000, 0.9510565162951535312, 1.000000000000000000, 0.9510565162951535312, 1.000000000000000000, 0.9510565162951535312, 1.000000000000000000, 0.9510565162951535312, 1.000000000000000000, 0.9510565162951535312, 1.000000000000000000, 0.9510565162951535312, 1.000000000000000000, 0.9510565162951535312, 1.000000000000000000, 0.9510565162951535312, 1.000000000000000000, 0.9510565162951535312, 1.000000000000000000, 0.9510565162951535312, 1.000000000000000000, 0.9510565162951535312, 1.000000000000000000, 0.9510565162951535312, 1.000000000000000000, 0.9510565162951535312, 1.000000000000000000, 0.9510565162951535312, 1.000000000000000000, 0.9510565162951535312, 1.000000000000000000, 0.9510565162951535312, 1.000000000000000000, 0.9510565162951535312, 1.000000000000000000, 0.9510565162951535312, 1.000000000000000000, 0.9510565162951535312, 1.000000000000000000, 0.9510565162951535312, 1.000000000000000000, 0.9510565162951535312, 1.000000000000000000, 0.9510565162951535312, 1.000000000000000000, 0.9510565162951535312, 1.000000000000000000, 0.9510565162951535312, 1.000000000000000000, 0.9510565162951535312, 1.000000000000000000, 0.9510565162951535312, 1.000000000000000000, 0.9510565162951535312, 1.000000000000000000, 0.9510565162951535312, 1.000000000000000000, 0.9510565162951535312, 1.000000000000000000, 0.9510565162951535312, 1.000000000000000000, 0.9510565162951535312, 1.000000000000000000),
 ( 0.3333333333333333703, 0.3170188387650512141, 0.3333333333333333703, 0.3170188387650512141, 0.3333333333333333703, 0.3170188387650512141, 0.3333333333333333703, 0.3170188387650512141, 0.3333333333333333703, 0.3170188387650512141, 0.3333333333333333703, 0.3170188387650512141, 0.3333333333333333703, 0.3170188387650512141, 0.3333333333333333703, 0.3170188387650512141, 0.3333333333333333703, 0.3170188387650512141, 0.3333333333333333703, 0.3170188387650512141, 0.3333333333333333703, 0.3170188387650512141, 0.3333333333333333703, 0.3170188387650512141, 0.3333333333333333703, 0.3170188387650512141, 0.3333333333333333703, 0.3170188387650512141, 0.3333333333333333703, 0.3170188387650512141, 0.3333333333333333703, 0.3170188387650512141, 0.3333333333333333703, 0.3170188387650512141, 0.3333333333333333703, 0.3170188387650512141, 0.3333333333333333703, 0.3170188387650512141, 0.3333333333333333703, 0.3170188387650512141, 0.3333333333333333703, 0.3170188387650512141, 0.3333333333333333703, 0.3170188387650512141, 0.3333333333333333703, 0.3170188387650512141, 0.3333333333333333703, 0.3170188387650512141, 0.3333333333333333703, 0.3170188387650512141, 0.3333333333333333703, 0.3170188387650512141, 0.3333333333333333703, 0.3170188387650512141, 0.3333333333333333703, 0.3170188387650512141, 0.3333333333333333703, 0.3170188387650512141, 0.3333333333333333703, 0.3170188387650512141, 0.3333333333333333703, 0.3170188387650512141, 0.3333333333333333703, 0.3170188387650512141, 0.3333333333333333703, 0.3170188387650512141, 0.3333333333333333703, 0.3170188387650512141, 0.3333333333333333703, 0.3170188387650512141, 0.3333333333333333703, 0.3170188387650512141, 0.3333333333333333703, 0.3170188387650512141, 0.3333333333333333703, 0.3170188387650512141, 0.3333333333333333703, 0.3170188387650512141, 0.3333333333333333703, 0.3170188387650512141, 0.3333333333333333703, 0.3170188387650512141, 0.3333333333333333703, 0.3170188387650512141, 0.3333333333333333703, 0.3170188387650512141, 0.3333333333333333703, 0.3170188387650512141, 0.3333333333333333703, 0.3170188387650512141, 0.3333333333333333703, 0.3170188387650512141, 0.3333333333333333703, 0.3170188387650512141, 0.3333333333333333703, 0.3170188387650512141, 0.3333333333333333703, 0.3170188387650512141, 0.3333333333333333703, 0.3170188387650512141, 0.3333333333333333703, 0.3170188387650512141, 0.3333333333333333703, 0.3170188387650512141, 0.3333333333333333703, 0.3170188387650512141, 0.3333333333333333703, 0.3170188387650512141, 0.3333333333333333703, 0.3170188387650512141, 0.3333333333333333703, 0.3170188387650512141, 0.3333333333333333703, 0.3170188387650512141, 0.3333333333333333703, 0.3170188387650512141, 0.3333333333333333703, 0.3170188387650512141, 0.3333333333333333703, 0.3170188387650512141, 0.3333333333333333703, 0.3170188387650512141, 0.3333333333333333703, 0.3170188387650512141, 0.3333333333333333703, 0.3170188387650512141, 0.3333333333333333703, 0.3170188387650512141, 0.3333333333333333703, 0.3170188387650512141, 0.3333333333333333703, 0.3170188387650512141, 0.3333333333333333703, 0.3170188387650512141, 0.3333333333333333703, 0.3170188387650512141, 0.3333333333333333703, 0.3170188387650512141, 0.3333333333333333703, 0.3170188387650512141, 0.3333333333333333703, 0.3170188387650512141, 0.3333333333333333703, 0.3170188387650512141, 0.3333333333333333703, 0.3170188387650512141, 0.3333333333333333703, 0.3170188387650512141, 0.3333333333333333703, 0.3170188387650512141, 0.3333333333333333703, 0.3170188387650512141, 0.3333333333333333703, 0.3170188387650512141, 0.3333333333333333703, 0.3170188387650512141, 0.3333333333333333703, 0.3170188387650512141, 0.3333333333333333703, 0.3170188387650512141, 0.3333333333333333703, 0.3170188387650512141, 0.3333333333333333703, 0.3170188387650512141, 0.3333333333333333703, 0.3170188387650512141, 0.3333333333333333703, 0.3170188387650512141, 0.3333333333333333703, 0.3170188387650512141, 0.3333333333333333703, 0.3170188387650512141, 0.3333333333333333703, 0.3170188387650512141, 0.3333333333333333703, 0.3170188387650512141, 0.3333333333333333703, 0.3170188387650512141, 0.3333333333333333703, 0.3170188387650512141, 0.3333333333333333703, 0.3170188387650512141, 0.3333333333333333703, 0.3170188387650512141, 0.3333333333333333703, 0.3170188387650512141, 0.3333333333333333703, 0.3170188387650512141, 0.3333333333333333703, 0.3170188387650512141, 0.3333333333333333703, 0.3170188387650512141, 0.3333333333333333703, 0.3170188387650512141, 0.3333333333333333703, 0.3170188387650512141, 0.3333333333333333703, 0.3170188387650512141, 0.3333333333333333703, 0.3170188387650512141, 0.3333333333333333703, 0.3170188387650512141, 0.3333333333333333703, 0.3170188387650512141, 0.3333333333333333703, 0.3170188387650512141, 0.3333333333333333703, 0.3170188387650512141, 0.3333333333333333703, 0.3170188387650512141, 0.3333333333333333703, 0.3170188387650512141, 0.3333333333333333703, 0.3170188387650512141, 0.3333333333333333703, 0.3170188387650512141, 0.3333333333333333703, 0.3170188387650512141, 0.3333333333333333703, 0.3170188387650512141, 0.3333333333333333703, 0.3170188387650512141, 0.3333333333333333703, 0.3170188387650512141, 0.3333333333333333703, 0.3170188387650512141, 0.3333333333333333703, 0.3170188387650512141, 0.3333333333333333703, 0.3170188387650512141, 0.3333333333333333703, 0.3170188387650512141, 0.3333333333333333703, 0.3170188387650512141, 0.3333333333333333703, 0.3170188387650512141, 0.3333333333333333703, 0.3170188387650512141, 0.3333333333333333703, 0.3170188387650512141, 0.3333333333333333703, 0.3170188387650512141, 0.3333333333333333703, 0.3170188387650512141, 0.3333333333333333703, 0.3170188387650512141, 0.3333333333333333703, 0.3170188387650512141, 0.3333333333333333703, 0.3170188387650512141, 0.3333333333333333703, 0.3170188387650512141, 0.3333333333333333703, 0.3170188387650512141, 0.3333333333333333703, 0.3170188387650512141, 0.3333333333333333703, 0.3170188387650512141, 0.3333333333333333703, 0.3170188387650512141, 0.3333333333333333703, 0.3170188387650512141, 0.3333333333333333703, 0.3170188387650512141, 0.3333333333333333703, 0.3170188387650512141, 0.3333333333333333703, 0.3170188387650512141, 0.3333333333333333703, 0.3170188387650512141, 0.3333333333333333703, 0.3170188387650512141, 0.3333333333333333703, 0.3170188387650512141, 0.3333333333333333703, 0.3170188387650512141, 0.3333333333333333703, 0.3170188387650512141, 0.3333333333333333703, 0.3170188387650512141, 0.3333333333333333703, 0.3170188387650512141, 0.3333333333333333703, 0.3170188387650512141, 0.3333333333333333703, 0.3170188387650512141, 0.3333333333333333703, 0.3170188387650512141, 0.3333333333333333703, 0.3170188387650512141, 0.3333333333333333703, 0.3170188387650512141, 0.3333333333333333703, 0.3170188387650512141, 0.3333333333333333703, 0.3170188387650512141, 0.3333333333333333703, 0.3170188387650512141, 0.3333333333333333703, 0.3170188387650512141, 0.3333333333333333703, 0.3170188387650512141, 0.3333333333333333703, 0.3170188387650512141, 0.3333333333333333703, 0.3170188387650512141, 0.3333333333333333703, 0.3170188387650512141, 0.3333333333333333703, 0.3170188387650512141, 0.3333333333333333703, 0.3170188387650512141, 0.3333333333333333703, 0.3170188387650512141, 0.3333333333333333703, 0.3170188387650512141, 0.3333333333333333703, 0.3170188387650512141, 0.3333333333333333703, 0.3170188387650512141, 0.3333333333333333703, 0.3170188387650512141, 0.3333333333333333703, 0.3170188387650512141, 0.3333333333333333703, 0.3170188387650512141, 0.3333333333333333703, 0.3170188387650512141, 0.3333333333333333703, 0.3170188387650512141, 0.3333333333333333703),
 ( 0.3333333333333333703, 0.3170188387650512141, 0.3333333333333333703, 0.3170188387650512141, 0.3333333333333333703, 0.3170188387650512141, 0.3333333333333333703, 0.3170188387650512141, 0.3333333333333333703, 0.3170188387650512141, 0.3333333333333333703, 0.3170188387650512141, 0.3333333333333333703, 0.3170188387650512141, 0.3333333333333333703, 0.3170188387650512141, 0.3333333333333333703, 0.3170188387650512141, 0.3333333333333333703, 0.3170188387650512141, 0.3333333333333333703, 0.3170188387650512141, 0.3333333333333333703, 0.3170188387650512141, 0.3333333333333333703, 0.3170188387650512141, 0.3333333333333333703, 0.3170188387650512141, 0.3333333333333333703, 0.3170188387650512141, 0.3333333333333333703, 0.3170188387650512141, 0.3333333333333333703, 0.3170188387650512141, 0.3333333333333333703, 0.3170188387650512141, 0.3333333333333333703, 0.3170188387650512141, 0.3333333333333333703, 0.3170188387650512141, 0.3333333333333333703, 0.3170188387650512141, 0.3333333333333333703, 0.3170188387650512141, 0.3333333333333333703, 0.3170188387650512141, 0.3333333333333333703, 0.3170188387650512141, 0.3333333333333333703, 0.3170188387650512141, 0.3333333333333333703, 0.3170188387650512141, 0.3333333333333333703, 0.3170188387650512141, 0.3333333333333333703, 0.3170188387650512141, 0.3333333333333333703, 0.3170188387650512141, 0.3333333333333333703, 0.3170188387650512141, 0.3333333333333333703, 0.3170188387650512141, 0.3333333333333333703, 0.3170188387650512141, 0.3333333333333333703, 0.3170188387650512141, 0.3333333333333333703, 0.3170188387650512141, 0.3333333333333333703, 0.3170188387650512141, 0.3333333333333333703, 0.3170188387650512141, 0.3333333333333333703, 0.3170188387650512141, 0.3333333333333333703, 0.3170188387650512141, 0.3333333333333333703, 0.3170188387650512141, 0.3333333333333333703, 0.3170188387650512141, 0.3333333333333333703, 0.3170188387650512141, 0.3333333333333333703, 0.3170188387650512141, 0.3333333333333333703, 0.3170188387650512141, 0.3333333333333333703, 0.3170188387650512141, 0.3333333333333333703, 0.3170188387650512141, 0.3333333333333333703, 0.3170188387650512141, 0.3333333333333333703, 0.3170188387650512141, 0.3333333333333333703, 0.3170188387650512141, 0.3333333333333333703, 0.3170188387650512141, 0.3333333333333333703, 0.3170188387650512141, 0.3333333333333333703, 0.3170188387650512141, 0.3333333333333333703, 0.3170188387650512141, 0.3333333333333333703, 0.3170188387650512141, 0.3333333333333333703, 0.3170188387650512141, 0.3333333333333333703, 0.3170188387650512141, 0.3333333333333333703, 0.3170188387650512141, 0.3333333333333333703, 0.3170188387650512141, 0.3333333333333333703, 0.3170188387650512141, 0.3333333333333333703, 0.3170188387650512141, 0.3333333333333333703, 0.3170188387650512141, 0.3333333333333333703, 0.3170188387650512141, 0.3333333333333333703, 0.3170188387650512141, 0.3333333333333333703, 0.3170188387650512141, 0.3333333333333333703, 0.3170188387650512141, 0.3333333333333333703, 0.3170188387650512141, 0.3333333333333333703, 0.3170188387650512141, 0.3333333333333333703, 0.3170188387650512141, 0.3333333333333333703, 0.3170188387650512141, 0.3333333333333333703, 0.3170188387650512141, 0.3333333333333333703, 0.3170188387650512141, 0.3333333333333333703, 0.3170188387650512141, 0.3333333333333333703, 0.3170188387650512141, 0.3333333333333333703, 0.3170188387650512141, 0.3333333333333333703, 0.3170188387650512141, 0.3333333333333333703, 0.3170188387650512141, 0.3333333333333333703, 0.3170188387650512141, 0.3333333333333333703, 0.3170188387650512141, 0.3333333333333333703, 0.3170188387650512141, 0.3333333333333333703, 0.3170188387650512141, 0.3333333333333333703, 0.3170188387650512141, 0.3333333333333333703, 0.3170188387650512141, 0.3333333333333333703, 0.3170188387650512141, 0.3333333333333333703, 0.3170188387650512141, 0.3333333333333333703, 0.3170188387650512141, 0.3333333333333333703, 0.3170188387650512141, 0.3333333333333333703, 0.3170188387650512141, 0.3333333333333333703, 0.3170188387650512141, 0.3333333333333333703, 0.3170188387650512141, 0.3333333333333333703, 0.3170188387650512141, 0.3333333333333333703, 0.3170188387650512141, 0.3333333333333333703, 0.3170188387650512141, 0.3333333333333333703, 0.3170188387650512141, 0.3333333333333333703, 0.3170188387650512141, 0.3333333333333333703, 0.3170188387650512141, 0.3333333333333333703, 0.3170188387650512141, 0.3333333333333333703, 0.3170188387650512141, 0.3333333333333333703, 0.3170188387650512141, 0.3333333333333333703, 0.3170188387650512141, 0.3333333333333333703, 0.3170188387650512141, 0.3333333333333333703, 0.3170188387650512141, 0.3333333333333333703, 0.3170188387650512141, 0.3333333333333333703, 0.3170188387650512141, 0.3333333333333333703, 0.3170188387650512141, 0.3333333333333333703, 0.3170188387650512141, 0.3333333333333333703, 0.3170188387650512141, 0.3333333333333333703, 0.3170188387650512141, 0.3333333333333333703, 0.3170188387650512141, 0.3333333333333333703, 0.3170188387650512141, 0.3333333333333333703, 0.3170188387650512141, 0.3333333333333333703, 0.3170188387650512141, 0.3333333333333333703, 0.3170188387650512141, 0.3333333333333333703, 0.3170188387650512141, 0.3333333333333333703, 0.3170188387650512141, 0.3333333333333333703, 0.3170188387650512141, 0.3333333333333333703, 0.3170188387650512141, 0.3333333333333333703, 0.3170188387650512141, 0.3333333333333333703, 0.3170188387650512141, 0.3333333333333333703, 0.3170188387650512141, 0.3333333333333333703, 0.3170188387650512141, 0.3333333333333333703, 0.3170188387650512141, 0.3333333333333333703, 0.3170188387650512141, 0.3333333333333333703, 0.3170188387650512141, 0.3333333333333333703, 0.3170188387650512141, 0.3333333333333333703, 0.3170188387650512141, 0.3333333333333333703, 0.3170188387650512141, 0.3333333333333333703, 0.3170188387650512141, 0.3333333333333333703, 0.3170188387650512141, 0.3333333333333333703, 0.3170188387650512141, 0.3333333333333333703, 0.3170188387650512141, 0.3333333333333333703, 0.3170188387650512141, 0.3333333333333333703, 0.3170188387650512141, 0.3333333333333333703, 0.3170188387650512141, 0.3333333333333333703, 0.3170188387650512141, 0.3333333333333333703, 0.3170188387650512141, 0.3333333333333333703, 0.3170188387650512141, 0.3333333333333333703, 0.3170188387650512141, 0.3333333333333333703, 0.3170188387650512141, 0.3333333333333333703, 0.3170188387650512141, 0.3333333333333333703, 0.3170188387650512141, 0.3333333333333333703, 0.3170188387650512141, 0.3333333333333333703, 0.3170188387650512141, 0.3333333333333333703, 0.3170188387650512141, 0.3333333333333333703, 0.3170188387650512141, 0.3333333333333333703, 0.3170188387650512141, 0.3333333333333333703, 0.3170188387650512141, 0.3333333333333333703, 0.3170188387650512141, 0.3333333333333333703, 0.3170188387650512141, 0.3333333333333333703, 0.3170188387650512141, 0.3333333333333333703, 0.3170188387650512141, 0.3333333333333333703, 0.3170188387650512141, 0.3333333333333333703, 0.3170188387650512141, 0.3333333333333333703, 0.3170188387650512141, 0.3333333333333333703, 0.3170188387650512141, 0.3333333333333333703, 0.3170188387650512141, 0.3333333333333333703, 0.3170188387650512141, 0.3333333333333333703, 0.3170188387650512141, 0.3333333333333333703, 0.3170188387650512141, 0.3333333333333333703, 0.3170188387650512141, 0.3333333333333333703, 0.3170188387650512141, 0.3333333333333333703, 0.3170188387650512141, 0.3333333333333333703, 0.3170188387650512141, 0.3333333333333333703, 0.3170188387650512141, 0.3333333333333333703, 0.3170188387650512141, 0.3333333333333333703, 0.3170188387650512141, 0.3333333333333333703, 0.3170188387650512141, 0.3333333333333333703),
 ( 1.000000000000000000, 0.9510565162951535312, 1.000000000000000000, 0.9510565162951535312, 1.000000000000000000, 0.9510565162951535312, 1.000000000000000000, 0.9510565162951535312, 1.000000000000000000, 0.9510565162951535312, 1.000000000000000000, 0.9510565162951535312, 1.000000000000000000, 0.9510565162951535312, 1.000000000000000000, 0.9510565162951535312, 1.000000000000000000, 0.9510565162951535312, 1.000000000000000000, 0.9510565162951535312, 1.000000000000000000, 0.9510565162951535312, 1.000000000000000000, 0.9510565162951535312, 1.000000000000000000, 0.9510565162951535312, 1.000000000000000000, 0.9510565162951535312, 1.000000000000000000, 0.9510565162951535312, 1.000000000000000000, 0.9510565162951535312, 1.000000000000000000, 0.9510565162951535312, 1.000000000000000000, 0.9510565162951535312, 1.000000000000000000, 0.9510565162951535312, 1.000000000000000000, 0.9510565162951535312, 1.000000000000000000, 0.9510565162951535312, 1.000000000000000000, 0.9510565162951535312, 1.000000000000000000, 0.9510565162951535312, 1.000000000000000000, 0.9510565162951535312, 1.000000000000000000, 0.9510565162951535312, 1.000000000000000000, 0.9510565162951535312, 1.000000000000000000, 0.9510565162951535312, 1.000000000000000000, 0.9510565162951535312, 1.000000000000000000, 0.9510565162951535312, 1.000000000000000000, 0.9510565162951535312, 1.000000000000000000, 0.9510565162951535312, 1.000000000000000000, 0.9510565162951535312, 1.000000000000000000, 0.9510565162951535312, 1.000000000000000000, 0.9510565162951535312, 1.000000000000000000, 0.9510565162951535312, 1.000000000000000000, 0.9510565162951535312, 1.000000000000000000, 0.9510565162951535312, 1.000000000000000000, 0.9510565162951535312, 1.000000000000000000, 0.9510565162951535312, 1.000000000000000000, 0.9510565162951535312, 1.000000000000000000, 0.9510565162951535312, 1.000000000000000000, 0.9510565162951535312, 1.000000000000000000, 0.9510565162951535312, 1.000000000000000000, 0.9510565162951535312, 1.000000000000000000, 0.9510565162951535312, 1.000000000000000000, 0.9510565162951535312, 1.000000000000000000, 0.9510565162951535312, 1.000000000000000000, 0.9510565162951535312, 1.000000000000000000, 0.9510565162951535312, 1.000000000000000000, 0.9510565162951535312, 1.000000000000000000, 0.9510565162951535312, 1.000000000000000000, 0.9510565162951535312, 1.000000000000000000, 0.9510565162951535312, 1.000000000000000000, 0.9510565162951535312, 1.000000000000000000, 0.9510565162951535312, 1.000000000000000000, 0.9510565162951535312, 1.000000000000000000, 0.9510565162951535312, 1.000000000000000000, 0.9510565162951535312, 1.000000000000000000, 0.9510565162951535312, 1.000000000000000000, 0.9510565162951535312, 1.000000000000000000, 0.9510565162951535312, 1.000000000000000000, 0.9510565162951535312, 1.000000000000000000, 0.9510565162951535312, 1.000000000000000000, 0.9510565162951535312, 1.000000000000000000, 0.9510565162951535312, 1.000000000000000000, 0.9510565162951535312, 1.000000000000000000, 0.9510565162951535312, 1.000000000000000000, 0.9510565162951535312, 1.000000000000000000, 0.9510565162951535312, 1.000000000000000000, 0.9510565162951535312, 1.000000000000000000, 0.9510565162951535312, 1.000000000000000000, 0.9510565162951535312, 1.000000000000000000, 0.9510565162951535312, 1.000000000000000000, 0.9510565162951535312, 1.000000000000000000, 0.9510565162951535312, 1.000000000000000000, 0.9510565162951535312, 1.000000000000000000, 0.9510565162951535312, 1.000000000000000000, 0.9510565162951535312, 1.000000000000000000, 0.9510565162951535312, 1.000000000000000000, 0.9510565162951535312, 1.000000000000000000, 0.9510565162951535312, 1.000000000000000000, 0.9510565162951535312, 1.000000000000000000, 0.9510565162951535312, 1.000000000000000000, 0.9510565162951535312, 1.000000000000000000, 0.9510565162951535312, 1.000000000000000000, 0.9510565162951535312, 1.000000000000000000, 0.9510565162951535312, 1.000000000000000000, 0.9510565162951535312, 1.000000000000000000, 0.9510565162951535312, 1.000000000000000000, 0.9510565162951535312, 1.000000000000000000, 0.9510565162951535312, 1.000000000000000000, 0.9510565162951535312, 1.000000000000000000, 0.9510565162951535312, 1.000000000000000000, 0.9510565162951535312, 1.000000000000000000, 0.9510565162951535312, 1.000000000000000000, 0.9510565162951535312, 1.000000000000000000, 0.9510565162951535312, 1.000000000000000000, 0.9510565162951535312, 1.000000000000000000, 0.9510565162951535312, 1.000000000000000000, 0.9510565162951535312, 1.000000000000000000, 0.9510565162951535312, 1.000000000000000000, 0.9510565162951535312, 1.000000000000000000, 0.9510565162951535312, 1.000000000000000000, 0.9510565162951535312, 1.000000000000000000, 0.9510565162951535312, 1.000000000000000000, 0.9510565162951535312, 1.000000000000000000, 0.9510565162951535312, 1.000000000000000000, 0.9510565162951535312, 1.000000000000000000, 0.9510565162951535312, 1.000000000000000000, 0.9510565162951535312, 1.000000000000000000, 0.9510565162951535312, 1.000000000000000000, 0.9510565162951535312, 1.000000000000000000, 0.9510565162951535312, 1.000000000000000000, 0.9510565162951535312, 1.000000000000000000, 0.9510565162951535312, 1.000000000000000000, 0.9510565162951535312, 1.000000000000000000, 0.9510565162951535312, 1.000000000000000000, 0.9510565162951535312, 1.000000000000000000, 0.9510565162951535312, 1.000000000000000000, 0.9510565162951535312, 1.000000000000000000, 0.9510565162951535312, 1.000000000000000000, 0.9510565162951535312, 1.000000000000000000, 0.9510565162951535312, 1.000000000000000000, 0.9510565162951535312, 1.000000000000000000, 0.9510565162951535312, 1.000000000000000000, 0.9510565162951535312, 1.000000000000000000, 0.9510565162951535312, 1.000000000000000000, 0.9510565162951535312, 1.000000000000000000, 0.9510565162951535312, 1.000000000000000000, 0.9510565162951535312, 1.000000000000000000, 0.9510565162951535312, 1.000000000000000000, 0.9510565162951535312, 1.000000000000000000, 0.9510565162951535312, 1.000000000000000000, 0.9510565162951535312, 1.000000000000000000, 0.9510565162951535312, 1.000000000000000000, 0.9510565162951535312, 1.000000000000000000, 0.9510565162951535312, 1.000000000000000000, 0.9510565162951535312, 1.000000000000000000, 0.9510565162951535312, 1.000000000000000000, 0.9510565162951535312, 1.000000000000000000, 0.9510565162951535312, 1.000000000000000000, 0.9510565162951535312, 1.000000000000000000, 0.9510565162951535312, 1.000000000000000000, 0.9510565162951535312, 1.000000000000000000, 0.9510565162951535312, 1.000000000000000000, 0.9510565162951535312, 1.000000000000000000, 0.9510565162951535312, 1.000000000000000000, 0.9510565162951535312, 1.000000000000000000, 0.9510565162951535312, 1.000000000000000000, 0.9510565162951535312, 1.000000000000000000, 0.9510565162951535312, 1.000000000000000000, 0.9510565162951535312, 1.000000000000000000, 0.9510565162951535312, 1.000000000000000000, 0.9510565162951535312, 1.000000000000000000, 0.9510565162951535312, 1.000000000000000000, 0.9510565162951535312, 1.000000000000000000, 0.9510565162951535312, 1.000000000000000000, 0.9510565162951535312, 1.000000000000000000, 0.9510565162951535312, 1.000000000000000000, 0.9510565162951535312, 1.000000000000000000, 0.9510565162951535312, 1.000000000000000000, 0.9510565162951535312, 1.000000000000000000, 0.9510565162951535312, 1.000000000000000000, 0.9510565162951535312, 1.000000000000000000, 0.9510565162951535312, 1.000000000000000000) ) ) 
 REPRESENTATION_ITEM ( '' )  SURFACE ( )  );
#31985=CARTESIAN_POINT ( 'NONE',  ( -0.8851648821498765418, 11.91128888458923285, -40.19999999999996732 ) ) ;
#31990=CARTESIAN_POINT ( 'NONE',  ( -4.129897239856814117, 16.99292663369196177, -66.30704692567387326 ) ) ;
#31991=CARTESIAN_POINT ( 'NONE',  ( -3.705139346311794313, 19.38786279086902198, -53.09999999999996589 ) ) ;
#31999=CARTESIAN_POINT ( 'NONE',  ( 1.985016409143818272, 21.39581405818570303, -68.84999999999996589 ) ) ;
#32001=CARTESIAN_POINT ( 'NONE',  ( 3.043106805520193525, 20.33772366180932067, -52.50704692567387610 ) ) ;
#32004=CARTESIAN_POINT ( 'NONE',  ( -2.017261720333081598, 21.13920729861251857, -30.89295307432606208 ) ) ;
#32007=CARTESIAN_POINT ( 'NONE',  ( 3.771071394011080269, 15.74153613859503764, -41.09295307432606137 ) ) ;
#32022=CARTESIAN_POINT ( 'NONE',  ( 5.301103610786608300, 20.20104720010253985, -48.14999999999997726 ) ) ;
#32037=CARTESIAN_POINT ( 'NONE',  ( -5.370428668309080500, 14.93501088608579153, -24.15704692567387468 ) ) ;
#32042=CARTESIAN_POINT ( 'NONE',  ( -4.318543150850367773, 18.18399003996480801, -40.94999999999996732 ) ) ;
#32043=CARTESIAN_POINT ( 'NONE',  ( -2.564989113914250662, 12.12957133169093282, -44.84295307432606137 ) ) ;
#32051=CARTESIAN_POINT ( 'NONE',  ( 4.342430937695320736, 16.96683151040971538, -58.94295307432605568 ) ) ;
#32066=CARTESIAN_POINT ( 'NONE',  ( 1.887862790868997109, 13.79486065368817194, -36.89999999999997016 ) ) ;
#32093=CARTESIAN_POINT ( 'NONE',  ( 4.294655364005415699, 16.66518840966061887, -37.95704692567387184 ) ) ;
#32094=CARTESIAN_POINT ( 'NONE',  ( 3.705139346311793869, 15.61213720913094960, -33.59999999999996589 ) ) ;
#32097=CARTESIAN_POINT ( 'NONE',  ( 3.898383833589191383, 21.60376697729997275, -31.49295307432605995 ) ) ;
#32099=CARTESIAN_POINT ( 'NONE',  ( 3.705139346311793869, 15.61213720913094960, -30.59999999999996589 ) ) ;
#32108=CARTESIAN_POINT ( 'NONE',  ( -3.091735541773221296, 20.59173554177323950, -47.24999999999995026 ) ) ;
#32111=CARTESIAN_POINT ( 'NONE',  ( -1.028604700431329233, 11.93400751992799513, -35.70704692567387184 ) ) ;
#32113=CARTESIAN_POINT ( 'NONE',  ( -3.091735541773221296, 20.59173554177323950, -62.24999999999995737 ) ) ;
#32119=( LENGTH_UNIT ( ) NAMED_UNIT ( * ) SI_UNIT ( .MILLI., .METRE. ) );
#32124=CARTESIAN_POINT ( 'NONE',  ( 5.588711115410763597, 18.38516488214980882, -72.29999999999996874 ) ) ;
#32128=CARTESIAN_POINT ( 'NONE',  ( 5.107581180293630396, 15.06055038898570686, -41.09295307432606137 ) ) ;
#32147=CARTESIAN_POINT ( 'NONE',  ( 2.564989113914249330, 22.87042866830903876, -67.34295307432606137 ) ) ;
#32153=CARTESIAN_POINT ( 'NONE',  ( 3.895814058185739448, 19.48501640914375344, -57.14999999999995595 ) ) ;
#32164=CARTESIAN_POINT ( 'NONE',  ( -2.439449611014227859, 22.60758118029364283, -66.90704692567388179 ) ) ;
#32165=CARTESIAN_POINT ( 'NONE',  ( -4.206979645153769098, 21.70697964515380107, -56.24999999999995737 ) ) ;
#32178=CARTESIAN_POINT ( 'NONE',  ( 4.975717084895059372, 14.80175253005754143, -53.10704692567387752 ) ) ;
#32181=CARTESIAN_POINT ( 'NONE',  ( 5.107581180293630396, 15.06055038898570686, -68.09295307432604716 ) ) ;
#32199=CARTESIAN_POINT ( 'NONE',  ( 4.001075405444606048, 21.50107540544455276, -44.99999999999997158 ) ) ;
#32203=CARTESIAN_POINT ( 'NONE',  ( 0.5331684895902240040, 13.15756906230466328, -59.55704692567387326 ) ) ;
#32204=CARTESIAN_POINT ( 'NONE',  ( -1.985016409143819605, 13.60418594181426855, -46.34999999999997300 ) ) ;
#32214=CARTESIAN_POINT ( 'NONE',  ( -0.6505131845895224529, 13.39282139548194195, -67.19999999999997442 ) ) ;
#32216=CARTESIAN_POINT ( 'NONE',  ( -2.121074495332175847, 13.67351099933674341, -44.85704692567387752 ) ) ;
#32220=CARTESIAN_POINT ( 'NONE',  ( -0.5070733663080690956, 13.37010276014318144, -44.69295307432606279 ) ) ;
#32233=CARTESIAN_POINT ( 'NONE',  ( -5.876318620034919782, 18.43071743580290089, -49.94999999999994600 ) ) ;
#32251=CARTESIAN_POINT ( 'NONE',  ( -5.611429750749524992, 16.75827493613162034, -24.30704692567386971 ) ) ;
#32256=CARTESIAN_POINT ( 'NONE',  ( 2.940415233664778416, 20.44041523366473712, -38.99999999999996447 ) ) ;
#32268=CARTESIAN_POINT ( 'NONE',  ( 2.837723661809363307, 20.54310680552015356, -58.49295307432606705 ) ) ;
#32284=CARTESIAN_POINT ( 'NONE',  ( -3.895814058185739448, 15.51498359085620571, -34.64999999999997016 ) ) ;
#32306=CARTESIAN_POINT ( 'NONE',  ( 3.639207298612508801, 15.48273827966686866, -32.10704692567387042 ) ) ;
#32307=CARTESIAN_POINT ( 'NONE',  ( -4.107178604518053611, 16.84948681541050775, -28.79999999999996518 ) ) ;
#32312=CARTESIAN_POINT ( 'NONE',  ( -3.898383833589191827, 13.39623302270000771, -38.99295307432604574 ) ) ;
#32313=CARTESIAN_POINT ( 'NONE',  ( 3.043106805520193525, 20.33772366180932067, -70.50704692567386189 ) ) ;
#32320=CARTESIAN_POINT ( 'NONE',  ( -3.705139346311794313, 19.38786279086902198, -44.09999999999996589 ) ) ;
#32323=CARTESIAN_POINT ( 'NONE',  ( -5.370428668309080500, 14.93501088608579153, -36.15704692567386758 ) ) ;
#32324=CARTESIAN_POINT ( 'NONE',  ( -5.876318620034919782, 18.43071743580290089, -28.94999999999996021 ) ) ;
#32326=CARTESIAN_POINT ( 'NONE',  ( 0.6505131845895220088, 21.60717860451803674, -65.69999999999996021 ) ) ;
#32339=CARTESIAN_POINT ( 'NONE',  ( 4.314955953707388936, 13.40099666339979123, -41.24295307432605284 ) ) ;
#32359=CARTESIAN_POINT ( 'NONE',  ( 3.705139346311793869, 15.61213720913094960, -27.59999999999996589 ) ) ;
#32360=CARTESIAN_POINT ( 'NONE',  ( 2.940415233664778416, 20.44041523366473712, -56.99999999999996447 ) ) ;
#32371=CARTESIAN_POINT ( 'NONE',  ( -2.837105286290963146, 12.26822144673588255, -62.85704692567387042 ) ) ;
#32372=CARTESIAN_POINT ( 'NONE',  ( 0.8851648821498760977, 23.08871111541074228, -56.69999999999997442 ) ) ;
#32385=CARTESIAN_POINT ( 'NONE',  ( 5.370428668309080500, 20.06498911391418360, -58.65704692567388179 ) ) ;
#32388=CARTESIAN_POINT ( 'NONE',  ( 5.231778553264135212, 20.33710528629089254, -73.64295307432605853 ) ) ;
#32402=CARTESIAN_POINT ( 'NONE',  ( -2.568848540478311904, 22.54164913259435465, -44.39999999999997016 ) ) ;
#32407=CARTESIAN_POINT ( 'NONE',  ( 3.965139115708213868, 19.34895832295540430, -64.65704692567386758 ) ) ;
#32408=CARTESIAN_POINT ( 'NONE',  ( 4.107178604518054499, 18.15051318458946383, -48.29999999999996874 ) ) ;
#32416=CARTESIAN_POINT ( 'NONE',  ( 1.985016409143818272, 21.39581405818570303, -62.84999999999995879 ) ) ;
#32418=CARTESIAN_POINT ( 'NONE',  ( 0.5331684895902240040, 13.15756906230466328, -44.55704692567387326 ) ) ;
#32423=CARTESIAN_POINT ( 'NONE',  ( 2.837723661809363307, 20.54310680552015356, -49.49295307432605995 ) ) ;
#32439=CARTESIAN_POINT ( 'NONE',  ( -5.876318620034919782, 18.43071743580290089, -43.94999999999995310 ) ) ;
#32453=CARTESIAN_POINT ( 'NONE',  ( -5.301103610786608300, 14.79895279989743706, -73.64999999999993463 ) ) ;
#32459=CARTESIAN_POINT ( 'NONE',  ( 1.887862790868997109, 13.79486065368817194, -45.89999999999997016 ) ) ;
#32460=CARTESIAN_POINT ( 'NONE',  ( -4.107178604518053611, 16.84948681541050775, -73.79999999999996874 ) ) ;
#32472=CARTESIAN_POINT ( 'NONE',  ( -2.017261720333081598, 21.13920729861251857, -57.89295307432605853 ) ) ;
#32487=CARTESIAN_POINT ( 'NONE',  ( -1.887862790868997553, 21.20513934631180319, -35.39999999999996305 ) ) ;
#32510=CARTESIAN_POINT ( 'NONE',  ( -4.129897239856814117, 16.99292663369196177, -30.30704692567387326 ) ) ;
#32515=CARTESIAN_POINT ( 'NONE',  ( -3.898383833589191827, 13.39623302270000771, -35.99295307432605995 ) ) ;
#32516=CARTESIAN_POINT ( 'NONE',  ( -4.129897239856814117, 16.99292663369196177, -72.30704692567387326 ) ) ;
#32523=CARTESIAN_POINT ( 'NONE',  ( 3.895814058185739448, 19.48501640914375344, -42.14999999999996305 ) ) ;
#32526=CARTESIAN_POINT ( 'NONE',  ( -4.103766977300021601, 13.60161616641083704, -33.00704692567387610 ) ) ;
#32527=CARTESIAN_POINT ( 'NONE',  ( 4.001075405444606048, 21.50107540544455276, -26.99999999999996803 ) ) ;
#32528=CARTESIAN_POINT ( 'NONE',  ( -3.895814058185739448, 15.51498359085620571, -67.64999999999997726 ) ) ;
#32540=CARTESIAN_POINT ( 'NONE',  ( -4.314955953707389824, 21.59900333660018390, -27.74295307432605995 ) ) ;
#32557=CARTESIAN_POINT ( 'NONE',  ( -2.940415233664778860, 14.55958476633523802, -28.49999999999996447 ) ) ;
#32558=CARTESIAN_POINT ( 'NONE',  ( 4.318543150850367773, 16.81600996003516357, -57.44999999999996732 ) ) ;
#32568=CARTESIAN_POINT ( 'NONE',  ( -0.7798958854283041253, 23.40020640687986386, -64.05704692567387326 ) ) ;
#32569=CARTESIAN_POINT ( 'NONE',  ( 5.588711115410763597, 18.38516488214980882, -57.29999999999996874 ) ) ;
#32584=CARTESIAN_POINT ( 'NONE',  ( 2.439449611014226971, 12.39241881970633230, -41.40704692567386758 ) ) ;
#32588=CARTESIAN_POINT ( 'NONE',  ( 5.231778553264135212, 20.33710528629089254, -58.64295307432606563 ) ) ;
#32606=CARTESIAN_POINT ( 'NONE',  ( 0.8851648821498760977, 23.08871111541074228, -44.69999999999996021 ) ) ;
#32609=CARTESIAN_POINT ( 'NONE',  ( 0.5331684895902240040, 13.15756906230466328, -62.55704692567387326 ) ) ;
#32610=CARTESIAN_POINT ( 'NONE',  ( 2.940415233664778416, 20.44041523366473712, -50.99999999999997158 ) ) ;
#32618=CARTESIAN_POINT ( 'NONE',  ( -1.887862790868997553, 21.20513934631180319, -68.39999999999997726 ) ) ;
#32620=CARTESIAN_POINT ( 'NONE',  ( 4.294655364005415699, 16.66518840966061887, -43.95704692567387184 ) ) ;
#32626=CARTESIAN_POINT ( 'NONE',  ( -3.771071394011080269, 19.25846386140493394, -36.59295307432605426 ) ) ;
#32633=CARTESIAN_POINT ( 'NONE',  ( 2.121074495332174958, 21.32648900066323350, -28.35704692567387397 ) ) ;
#32640=CARTESIAN_POINT ( 'NONE',  ( 5.876318620034919782, 16.56928256419707068, -45.44999999999996021 ) ) ;
#32657=CARTESIAN_POINT ( 'NONE',  ( 4.206979645153767322, 13.29302035484617051, -69.74999999999997158 ) ) ;
#32662=CARTESIAN_POINT ( 'NONE',  ( -4.318543150850367773, 18.18399003996480801, -43.94999999999995310 ) ) ;
#32675=CARTESIAN_POINT ( 'NONE',  ( 4.084459969179292216, 18.29395300287091430, -49.79295307432606421 ) ) ;
#32680=CARTESIAN_POINT ( 'NONE',  ( 4.342430937695320736, 16.96683151040971538, -61.94295307432605568 ) ) ;
#32691=CARTESIAN_POINT ( 'NONE',  ( -4.107178604518053611, 16.84948681541050775, -34.79999999999996163 ) ) ;
#32716=CARTESIAN_POINT ( 'NONE',  ( -0.5331684895902242260, 21.84243093769531185, -31.05704692567387681 ) ) ;
#32720=CARTESIAN_POINT ( 'NONE',  ( -5.231778553264134324, 14.66289471370907727, -33.14295307432605853 ) ) ;
#32721=CARTESIAN_POINT ( 'NONE',  ( -4.294655364005415699, 18.33481159033935626, -60.45704692567387895 ) ) ;
#32729=CARTESIAN_POINT ( 'NONE',  ( 1.985016409143818272, 21.39581405818570303, -41.84999999999995879 ) ) ;
#32732=CARTESIAN_POINT ( 'NONE',  ( 4.975717084895059372, 14.80175253005754143, -38.10704692567387752 ) ) ;
#32734=CARTESIAN_POINT ( 'NONE',  ( 3.091735541773220852, 14.40826445822673563, -60.74999999999995737 ) ) ;
#32746=CARTESIAN_POINT ( 'NONE',  ( -3.898383833589191827, 13.39623302270000771, -35.99295307432605995 ) ) ;
#32767=CARTESIAN_POINT ( 'NONE',  ( 3.895814058185739448, 19.48501640914375344, -54.14999999999997726 ) ) ;
#32775=CARTESIAN_POINT ( 'NONE',  ( -3.895814058185739448, 15.51498359085620571, -73.64999999999993463 ) ) ;
#32777=CARTESIAN_POINT ( 'NONE',  ( 2.439449611014226971, 12.39241881970633230, -68.40704692567388179 ) ) ;
#32778=CARTESIAN_POINT ( 'NONE',  ( -4.206979645153769098, 21.70697964515380107, -53.24999999999996447 ) ) ;
#32789=CARTESIAN_POINT ( 'NONE',  ( 5.370428668309080500, 20.06498911391418360, -43.65704692567387468 ) ) ;
#32793=CARTESIAN_POINT ( 'NONE',  ( 0.7417250638684235176, 23.11142975074950101, -61.19295307432605568 ) ) ;
#32810=CARTESIAN_POINT ( 'NONE',  ( -4.206979645153768210, 21.70697964515380107, -29.24999999999996447 ) ) ;
#32813=CARTESIAN_POINT ( 'NONE',  ( 4.294655364005415699, 16.66518840966061887, -55.95704692567386473 ) ) ;
#32815=CARTESIAN_POINT ( 'NONE',  ( -3.091735541773221296, 20.59173554177323950, -44.24999999999997868 ) ) ;
#32825=CARTESIAN_POINT ( 'NONE',  ( -4.107178604518053611, 16.84948681541050775, -58.79999999999996163 ) ) ;
#32827=CARTESIAN_POINT ( 'NONE',  ( 1.758463861404912620, 13.72892860598888731, -44.40704692567387468 ) ) ;
#32831=CARTESIAN_POINT ( 'NONE',  ( -1.848958322955462474, 13.53486088429179546, -38.84295307432606137 ) ) ;
#32838=CARTESIAN_POINT ( 'NONE',  ( 1.758463861404912620, 13.72892860598888731, -26.40704692567387823 ) ) ;
#32847=CARTESIAN_POINT ( 'NONE',  ( -0.8851648821498765418, 11.91128888458923285, -34.19999999999996732 ) ) ;
#32868=CARTESIAN_POINT ( 'NONE',  ( -5.588711115410763597, 16.61483511785016987, -73.79999999999996874 ) ) ;
#32873=CARTESIAN_POINT ( 'NONE',  ( 1.985016409143818272, 21.39581405818570303, -35.84999999999996589 ) ) ;
#32884=CARTESIAN_POINT ( 'NONE',  ( 3.826489000663266360, 19.62107449533211678, -46.64295307432605853 ) ) ;
#32890=CARTESIAN_POINT ( 'NONE',  ( 3.826489000663266360, 19.62107449533211678, -61.64295307432606563 ) ) ;
#32901=CARTESIAN_POINT ( 'NONE',  ( 4.318543150850367773, 16.81600996003516357, -27.44999999999996021 ) ) ;
#32910=CARTESIAN_POINT ( 'NONE',  ( -2.701047200102606016, 12.19889638921340413, -70.34999999999993747 ) ) ;
#32926=CARTESIAN_POINT ( 'NONE',  ( 2.698247469942395949, 12.52428291510489977, -68.39295307432607274 ) ) ;
#32931=CARTESIAN_POINT ( 'NONE',  ( 0.7939530028709752552, 21.58445996917927445, -37.20704692567387184 ) ) ;
#32937=CARTESIAN_POINT ( 'NONE',  ( 0.7417250638684235176, 23.11142975074950101, -28.19295307432605568 ) ) ;
#32938=CARTESIAN_POINT ( 'NONE',  ( 3.639207298612508801, 15.48273827966686866, -68.10704692567387042 ) ) ;
#32945=CARTESIAN_POINT ( 'NONE',  ( -2.940415233664778860, 14.55958476633523802, -40.49999999999996447 ) ) ;
#32948=CARTESIAN_POINT ( 'NONE',  ( 4.099003336600150149, 13.18504404629255689, -29.25704692567387255 ) ) ;
#32950=CARTESIAN_POINT ( 'NONE',  ( 0.6505131845895220088, 21.60717860451803674, -56.69999999999997442 ) ) ;
#32964=CARTESIAN_POINT ( 'NONE',  ( -5.565992480072003978, 16.47139529956871229, -33.29295307432605711 ) ) ;
#32982=CARTESIAN_POINT ( 'NONE',  ( -0.6505131845895224529, 13.39282139548194195, -49.19999999999996732 ) ) ;
#32991=CARTESIAN_POINT ( 'NONE',  ( 4.084459969179292216, 18.29395300287091430, -28.79295307432605355 ) ) ;
#32994=CARTESIAN_POINT ( 'NONE',  ( -5.852430833189966819, 18.58153898617744915, -57.45704692567387895 ) ) ;
#32995=CARTESIAN_POINT ( 'NONE',  ( 5.301103610786608300, 20.20104720010254340, -48.14999999999997016 ) ) ;
#33008=CARTESIAN_POINT ( 'NONE',  ( 5.611429750749524992, 18.24172506386835479, -43.80704692567387326 ) ) ;
#33012=CARTESIAN_POINT ( 'NONE',  ( 3.898383833589191383, 21.60376697729997275, -58.49295307432606705 ) ) ;
#33027=CARTESIAN_POINT ( 'NONE',  ( 2.701047200102605572, 22.80110361078655856, -35.84999999999996589 ) ) ;
#33030=CARTESIAN_POINT ( 'NONE',  ( 2.983759233219601459, 14.30028814967311668, -56.25704692567388321 ) ) ;
#33031=CARTESIAN_POINT ( 'NONE',  ( -0.6839900399647738105, 21.81854315085035623, -41.54999999999996874 ) ) ;
#33032=CARTESIAN_POINT ( 'NONE',  ( 0.6839900399647733664, 13.18145684914961357, -70.04999999999996874 ) ) ;
#33040=CARTESIAN_POINT ( 'NONE',  ( -0.6839900399647736995, 21.81854315085035623, -50.54999999999996163 ) ) ;
#33043=CARTESIAN_POINT ( 'NONE',  ( -4.129897239856814117, 16.99292663369196177, -42.30704692567387326 ) ) ;
#33044=CARTESIAN_POINT ( 'NONE',  ( -4.001075405444606936, 13.49892459455542060, -73.49999999999997158 ) ) ;
#33047=CARTESIAN_POINT ( 'NONE',  ( 4.084459969179292216, 18.29395300287091430, -37.79295307432605711 ) ) ;
#33053=CARTESIAN_POINT ( 'NONE',  ( -0.5331684895902242260, 21.84243093769531185, -28.05704692567386971 ) ) ;
#33059=CARTESIAN_POINT ( 'NONE',  ( -0.9307174358028533767, 23.37631862003491889, -41.54999999999996874 ) ) ;
#33077=CARTESIAN_POINT ( 'NONE',  ( -4.206979645153768210, 21.70697964515380107, -65.24999999999995737 ) ) ;
#33082=CARTESIAN_POINT ( 'NONE',  ( -0.6839900399647736995, 21.81854315085035623, -35.54999999999994742 ) ) ;
#33093=CARTESIAN_POINT ( 'NONE',  ( 3.199711850326839357, 14.51624076678035635, -47.24295307432605995 ) ) ;
#33098=CARTESIAN_POINT ( 'NONE',  ( 3.199711850326839357, 14.51624076678035635, -68.24295307432605284 ) ) ;
#33110=CARTESIAN_POINT ( 'NONE',  ( -3.705139346311794313, 19.38786279086902198, -29.09999999999996589 ) ) ;
#33120=CARTESIAN_POINT ( 'NONE',  ( 2.701047200102605572, 22.80110361078655856, -71.84999999999998010 ) ) ;
#33136=CARTESIAN_POINT ( 'NONE',  ( 2.564989113914249330, 22.87042866830903876, -64.34295307432606137 ) ) ;
#33145=CARTESIAN_POINT ( 'NONE',  ( -0.8348115903393239501, 21.79465536400541126, -73.04295307432606421 ) ) ;
#33146=CARTESIAN_POINT ( 'NONE',  ( -4.129897239856814117, 16.99292663369196177, -66.30704692567387326 ) ) ;
#33157=CARTESIAN_POINT ( 'NONE',  ( 4.975717084895059372, 14.80175253005754143, -26.10704692567387397 ) ) ;
#33159=CARTESIAN_POINT ( 'NONE',  ( 4.318543150850367773, 16.81600996003516357, -57.44999999999996732 ) ) ;
#33171=CARTESIAN_POINT ( 'NONE',  ( 1.081538986177402295, 11.64756916681001186, -35.54295307432605711 ) ) ;
#33191=CARTESIAN_POINT ( 'NONE',  ( -0.6505131845895224529, 13.39282139548194195, -43.19999999999996732 ) ) ;
#33200=CARTESIAN_POINT ( 'NONE',  ( -0.6505131845895224529, 13.39282139548194195, -70.19999999999997442 ) ) ;
#33202=CARTESIAN_POINT ( 'NONE',  ( 1.028604700431328567, 23.06599248007198355, -58.20704692567387184 ) ) ;
#33203=CARTESIAN_POINT ( 'NONE',  ( -0.9307174358028534877, 23.37631862003491889, -41.54999999999996874 ) ) ;
#33216=CARTESIAN_POINT ( 'NONE',  ( 4.103766977300021601, 21.39838383358913987, -43.50704692567387610 ) ) ;
#33222=CARTESIAN_POINT ( 'NONE',  ( -5.900206406879871857, 18.27989588542834554, -57.44295307432606990 ) ) ;
#33238=CARTESIAN_POINT ( 'NONE',  ( 4.001075405444606048, 21.50107540544455276, -32.99999999999996447 ) ) ;
#33241=CARTESIAN_POINT ( 'NONE',  ( 2.121074495332174958, 21.32648900066323350, -55.35704692567387752 ) ) ;
#33250=CARTESIAN_POINT ( 'NONE',  ( 3.091735541773220852, 14.40826445822673563, -51.74999999999994316 ) ) ;
#33252=CARTESIAN_POINT ( 'NONE',  ( -3.043106805520194413, 14.66227633819065623, -33.00704692567387610 ) ) ;
#33256=CARTESIAN_POINT ( 'NONE',  ( 0.5070733663080689846, 21.62989723985679902, -34.19295307432605568 ) ) ;
#33265=CARTESIAN_POINT ( 'NONE',  ( -1.758463861404912842, 21.27107139401109137, -27.90704692567387823 ) ) ;
#33272=CARTESIAN_POINT ( 'NONE',  ( 0.8851648821498760977, 23.08871111541074228, -38.69999999999996021 ) ) ;
#33288=CARTESIAN_POINT ( 'NONE',  ( 2.568848540478311460, 12.45835086740561692, -63.89999999999997016 ) ) ;
#33293=CARTESIAN_POINT ( 'NONE',  ( 3.091735541773220852, 14.40826445822673563, -30.74999999999995737 ) ) ;
#33294=CARTESIAN_POINT ( 'NONE',  ( 3.895814058185739892, 19.48501640914376054, -72.14999999999996305 ) ) ;
#33306=CARTESIAN_POINT ( 'NONE',  ( 0.5070733663080689846, 21.62989723985679902, -46.19295307432605568 ) ) ;
#33311=CARTESIAN_POINT ( 'NONE',  ( 0.5070733663080689846, 21.62989723985679902, -61.19295307432605568 ) ) ;
#33330=CARTESIAN_POINT ( 'NONE',  ( 5.301103610786608300, 20.20104720010253985, -72.14999999999996305 ) ) ;
#33349=CARTESIAN_POINT ( 'NONE',  ( 1.081538986177402295, 11.64756916681001186, -50.54295307432606421 ) ) ;
#33358=CARTESIAN_POINT ( 'NONE',  ( -5.565992480072003978, 16.47139529956871229, -27.29295307432605355 ) ) ;
#33359=CARTESIAN_POINT ( 'NONE',  ( 2.983759233219601459, 14.30028814967311668, -62.25704692567386900 ) ) ;
#33372=CARTESIAN_POINT ( 'NONE',  ( -4.099003336600151925, 21.81495595370741469, -30.75704692567387610 ) ) ;
#33375=CARTESIAN_POINT ( 'NONE',  ( -0.6505131845895224529, 13.39282139548194195, -55.19999999999997442 ) ) ;
#33388=CARTESIAN_POINT ( 'NONE',  ( -5.900206406879871857, 18.27989588542834554, -33.44295307432605568 ) ) ;
#33409=CARTESIAN_POINT ( 'NONE',  ( -4.107178604518053611, 16.84948681541050775, -40.79999999999996874 ) ) ;
#33418=CARTESIAN_POINT ( 'NONE',  ( -3.091735541773221296, 20.59173554177323950, -65.24999999999995737 ) ) ;
#33421=CARTESIAN_POINT ( 'NONE',  ( 5.852430833189966819, 16.41846101382252243, -55.95704692567386473 ) ) ;
#33422=CARTESIAN_POINT ( 'NONE',  ( -0.9307174358028534877, 23.37631862003491889, -50.54999999999996163 ) ) ;
#33434=CARTESIAN_POINT ( 'NONE',  ( -5.611429750749524992, 16.75827493613162034, -45.30704692567388037 ) ) ;
#33442=CARTESIAN_POINT ( 'NONE',  ( -5.231778553264134324, 14.66289471370907727, -57.14295307432605142 ) ) ;
#33457=CARTESIAN_POINT ( 'NONE',  ( 2.701047200102605572, 22.80110361078655856, -32.84999999999996589 ) ) ;
#33460=CARTESIAN_POINT ( 'NONE',  ( 3.043106805520193525, 20.33772366180932067, -55.50704692567387610 ) ) ;
#33461=CARTESIAN_POINT ( 'NONE',  ( -4.107178604518053611, 16.84948681541050775, -70.79999999999996874 ) ) ;
#33468=CARTESIAN_POINT ( 'NONE',  ( 0.6505131845895220088, 21.60717860451803674, -53.69999999999996732 ) ) ;
#33471=CARTESIAN_POINT ( 'NONE',  ( 0.5331684895902240040, 13.15756906230466328, -35.55704692567386616 ) ) ;
#33472=CARTESIAN_POINT ( 'NONE',  ( 2.568848540478311460, 12.45835086740561692, -69.89999999999996305 ) ) ;
#33476=CARTESIAN_POINT ( 'NONE',  ( 0.8348115903393232839, 13.20534463599456387, -32.54295307432605711 ) ) ;
#33484=CARTESIAN_POINT ( 'NONE',  ( -0.7798958854283041253, 23.40020640687986386, -70.05704692567387326 ) ) ;
#33492=CARTESIAN_POINT ( 'NONE',  ( -5.876318620034919782, 18.43071743580290089, -40.94999999999996732 ) ) ;
#33508=CARTESIAN_POINT ( 'NONE',  ( 0.9307174358028528216, 11.62368137996505801, -61.04999999999995453 ) ) ;
#33514=CARTESIAN_POINT ( 'NONE',  ( 0.6505131845895220088, 21.60717860451803674, -29.69999999999996376 ) ) ;
#33515=CARTESIAN_POINT ( 'NONE',  ( 3.091735541773220852, 14.40826445822673740, -69.74999999999997158 ) ) ;
#33529=CARTESIAN_POINT ( 'NONE',  ( 4.084459969179292216, 18.29395300287091430, -46.79295307432605711 ) ) ;
#33534=CARTESIAN_POINT ( 'NONE',  ( -2.017261720333081598, 21.13920729861251857, -63.89295307432605853 ) ) ;
#33545=CARTESIAN_POINT ( 'NONE',  ( 3.091735541773220852, 14.40826445822673563, -27.74999999999995381 ) ) ;
#33554=CARTESIAN_POINT ( 'NONE',  ( -4.206979645153768210, 21.70697964515380107, -65.24999999999995737 ) ) ;
#33574=CARTESIAN_POINT ( 'NONE',  ( -3.898383833589191827, 13.39623302270000771, -56.99295307432605995 ) ) ;
#33584=CARTESIAN_POINT ( 'NONE',  ( -5.900206406879871857, 18.27989588542834554, -27.44295307432605568 ) ) ;
#33586=CARTESIAN_POINT ( 'NONE',  ( 1.758463861404912620, 13.72892860598888731, -68.40704692567388179 ) ) ;
#33599=CARTESIAN_POINT ( 'NONE',  ( -5.611429750749524992, 16.75827493613162034, -27.30704692567386971 ) ) ;
#33601=CARTESIAN_POINT ( 'NONE',  ( -3.705139346311794313, 19.38786279086902198, -56.09999999999996589 ) ) ;
#33612=CARTESIAN_POINT ( 'NONE',  ( -2.837723661809363751, 14.45689319447982335, -71.99295307432603863 ) ) ;
#33633=CARTESIAN_POINT ( 'NONE',  ( 3.705139346311793869, 15.61213720913094960, -42.59999999999996589 ) ) ;
#33643=CARTESIAN_POINT ( 'NONE',  ( 3.895814058185739448, 19.48501640914375344, -69.14999999999994884 ) ) ;
#33645=CARTESIAN_POINT ( 'NONE',  ( -2.837105286290963146, 12.26822144673588255, -56.85704692567387042 ) ) ;
#33646=CARTESIAN_POINT ( 'NONE',  ( -5.301103610786608300, 14.79895279989743528, -49.64999999999995595 ) ) ;
#33653=( GEOMETRIC_REPRESENTATION_CONTEXT ( 3 ) GLOBAL_UNCERTAINTY_ASSIGNED_CONTEXT ( ( #10553 ) ) GLOBAL_UNIT_ASSIGNED_CONTEXT ( ( #31515, #15374, #28321 ) ) REPRESENTATION_CONTEXT ( 'NONE', 'WORKASPACE' ) );
#33659=CARTESIAN_POINT ( 'NONE',  ( 1.028604700431328567, 23.06599248007198355, -37.20704692567387184 ) ) ;
#33664=CARTESIAN_POINT ( 'NONE',  ( 5.107581180293630396, 15.06055038898570686, -53.09295307432605426 ) ) ;
#33679=CARTESIAN_POINT ( 'NONE',  ( -2.568848540478311904, 22.54164913259435465, -32.39999999999996305 ) ) ;
#33683=CARTESIAN_POINT ( 'NONE',  ( -1.758463861404912842, 21.27107139401109137, -48.90704692567388179 ) ) ;
#33692=CARTESIAN_POINT ( 'NONE',  ( 3.895814058185739448, 19.48501640914375344, -57.14999999999995595 ) ) ;
#33694=CARTESIAN_POINT ( 'NONE',  ( -2.121074495332175847, 13.67351099933674341, -32.85704692567387752 ) ) ;
#33706=CARTESIAN_POINT ( 'NONE',  ( -2.837105286290963146, 12.26822144673588255, -62.85704692567387042 ) ) ;
#33712=CARTESIAN_POINT ( 'NONE',  ( 5.041649132594343996, 14.93115145952162415, -39.59999999999996589 ) ) ;
#33726=CARTESIAN_POINT ( 'NONE',  ( 0.8851648821498760977, 23.08871111541074228, -65.69999999999996021 ) ) ;
#33731=CARTESIAN_POINT ( 'NONE',  ( -1.985016409143819605, 13.60418594181426855, -31.34999999999996945 ) ) ;
#33732=CARTESIAN_POINT ( 'NONE',  ( -1.985016409143819605, 13.60418594181426855, -67.34999999999996589 ) ) ;
#33742=CARTESIAN_POINT ( 'NONE',  ( -2.837723661809363751, 14.45689319447982335, -32.99295307432605995 ) ) ;
#33747=CARTESIAN_POINT ( 'NONE',  ( 0.8348115903393232839, 13.20534463599456387, -50.54295307432606421 ) ) ;
#33765=CARTESIAN_POINT ( 'NONE',  ( -2.701047200102606016, 12.19889638921340413, -67.34999999999996589 ) ) ;
#33785=CARTESIAN_POINT ( 'NONE',  ( -5.565992480072003978, 16.47139529956871229, -54.29295307432607132 ) ) ;
#33793=CARTESIAN_POINT ( 'NONE',  ( 0.5070733663080689846, 21.62989723985679902, -70.19295307432605568 ) ) ;
#33795=CARTESIAN_POINT ( 'NONE',  ( -0.7939530028709754772, 13.41554003082070246, -50.70704692567387184 ) ) ;
#33807=CARTESIAN_POINT ( 'NONE',  ( -2.940415233664778860, 14.55958476633523802, -55.49999999999996447 ) ) ;
#33818=CARTESIAN_POINT ( 'NONE',  ( 1.848958322955461808, 21.46513911570817612, -70.34295307432606137 ) ) ;
#33830=CARTESIAN_POINT ( 'NONE',  ( 3.091735541773220852, 14.40826445822673740, -36.74999999999995737 ) ) ;
#33835=CARTESIAN_POINT ( 'NONE',  ( 4.318543150850367773, 16.81600996003516357, -45.44999999999996021 ) ) ;
#33842=CARTESIAN_POINT ( 'NONE',  ( -3.705139346311794313, 19.38786279086902198, -62.09999999999996589 ) ) ;
#33844=CARTESIAN_POINT ( 'NONE',  ( 4.099003336600150149, 13.18504404629255689, -56.25704692567388321 ) ) ;
#33845=CARTESIAN_POINT ( 'NONE',  ( -5.588711115410763597, 16.61483511785016987, -43.79999999999996163 ) ) ;
#33858=CARTESIAN_POINT ( 'NONE',  ( -2.837105286290963146, 12.26822144673588255, -38.85704692567387752 ) ) ;
#33863=CARTESIAN_POINT ( 'NONE',  ( -5.900206406879871857, 18.27989588542834554, -51.44295307432605568 ) ) ;
#33878=CARTESIAN_POINT ( 'NONE',  ( -2.564989113914250662, 12.12957133169093282, -74.84295307432606137 ) ) ;
#33881=CARTESIAN_POINT ( 'NONE',  ( -3.043106805520194413, 14.66227633819065623, -45.00704692567388321 ) ) ;
#33882=CARTESIAN_POINT ( 'NONE',  ( -2.940415233664778860, 14.55958476633523802, -70.49999999999997158 ) ) ;
#33891=CARTESIAN_POINT ( 'NONE',  ( -0.6505131845895224529, 13.39282139548194195, -49.19999999999996732 ) ) ;
#33894=CARTESIAN_POINT ( 'NONE',  ( 2.983759233219601459, 14.30028814967311668, -38.25704692567386900 ) ) ;
#33904=CARTESIAN_POINT ( 'NONE',  ( 2.439449611014226971, 12.39241881970633230, -68.40704692567388179 ) ) ;
#33908=CARTESIAN_POINT ( 'NONE',  ( 4.206979645153767322, 13.29302035484617051, -30.74999999999995737 ) ) ;
#33927=CARTESIAN_POINT ( 'NONE',  ( 4.206979645153767322, 13.29302035484617051, -60.74999999999995737 ) ) ;
#33931=CARTESIAN_POINT ( 'NONE',  ( -3.639207298612509689, 19.51726172033310647, -69.60704692567387042 ) ) ;
#33932=CARTESIAN_POINT ( 'NONE',  ( 4.107178604518054499, 18.15051318458946383, -66.29999999999996874 ) ) ;
#33944=CARTESIAN_POINT ( 'NONE',  ( 3.771071394011080269, 15.74153613859503764, -32.09295307432605426 ) ) ;
#33949=CARTESIAN_POINT ( 'NONE',  ( 1.848958322955461808, 21.46513911570817612, -55.34295307432606137 ) ) ;
#33964=CARTESIAN_POINT ( 'NONE',  ( 0.8851648821498760977, 23.08871111541074228, -53.69999999999996732 ) ) ;
#33986=CARTESIAN_POINT ( 'NONE',  ( 1.081538986177402295, 11.64756916681001186, -56.54295307432606421 ) ) ;
#33997=CARTESIAN_POINT ( 'NONE',  ( -4.342430937695320736, 18.03316848959025620, -69.44295307432605568 ) ) ;
#33999=CARTESIAN_POINT ( 'NONE',  ( 1.758463861404912620, 13.72892860598888731, -50.40704692567388179 ) ) ;
#34013=CARTESIAN_POINT ( 'NONE',  ( 1.985016409143818272, 21.39581405818570303, -41.84999999999995879 ) ) ;
#34026=CARTESIAN_POINT ( 'NONE',  ( 1.848958322955461808, 21.46513911570817612, -76.34295307432604716 ) ) ;
#34038=CARTESIAN_POINT ( 'NONE',  ( 1.887862790868997109, 13.79486065368817194, -36.89999999999997016 ) ) ;
#34041=CARTESIAN_POINT ( 'NONE',  ( -2.940415233664778860, 14.55958476633523802, -37.49999999999996447 ) ) ;
#34050=CARTESIAN_POINT ( 'NONE',  ( 0.6839900399647733664, 13.18145684914961357, -61.04999999999995453 ) ) ;
#34052=CARTESIAN_POINT ( 'NONE',  ( -2.837105286290963146, 12.26822144673588255, -47.85704692567386331 ) ) ;
#34053=CARTESIAN_POINT ( 'NONE',  ( 5.876318620034919782, 16.56928256419707068, -36.44999999999996732 ) ) ;
#34067=CARTESIAN_POINT ( 'NONE',  ( -2.837105286290963146, 12.26822144673588255, -32.85704692567387752 ) ) ;
#34070=CARTESIAN_POINT ( 'NONE',  ( 0.7417250638684235176, 23.11142975074950101, -52.19295307432606279 ) ) ;
#34086=CARTESIAN_POINT ( 'NONE',  ( 5.231778553264135212, 20.33710528629089254, -73.64295307432605853 ) ) ;
#34089=CARTESIAN_POINT ( 'NONE',  ( -3.639207298612509689, 19.51726172033310647, -42.60704692567387752 ) ) ;
#34090=CARTESIAN_POINT ( 'NONE',  ( 0.6505131845895220088, 21.60717860451803674, -65.69999999999996021 ) ) ;
#34099=CARTESIAN_POINT ( 'NONE',  ( -3.965139115708213868, 15.65104167704456906, -33.15704692567386047 ) ) ;
#34100=CARTESIAN_POINT ( 'NONE',  ( -0.9307174358028534877, 23.37631862003491889, -62.54999999999996874 ) ) ;
#34113=CARTESIAN_POINT ( 'NONE',  ( 5.852430833189966819, 16.41846101382252243, -64.95704692567387895 ) ) ;
#34116=CARTESIAN_POINT ( 'NONE',  ( -2.568848540478311904, 22.54164913259435465, -29.39999999999996660 ) ) ;
#34132=CARTESIAN_POINT ( 'NONE',  ( -5.041649132594344884, 20.06884854047834921, -53.09999999999996589 ) ) ;
#34135=CARTESIAN_POINT ( 'NONE',  ( 3.043106805520193525, 20.33772366180932067, -67.50704692567386189 ) ) ;
#34136=CARTESIAN_POINT ( 'NONE',  ( 4.107178604518054499, 18.15051318458946383, -63.29999999999996874 ) ) ;
#34150=CARTESIAN_POINT ( 'NONE',  ( 4.342430937695320736, 16.96683151040971538, -31.94295307432605568 ) ) ;
#34153=CARTESIAN_POINT ( 'NONE',  ( 3.199711850326839357, 14.51624076678035635, -53.24295307432605995 ) ) ;
#34167=CARTESIAN_POINT ( 'NONE',  ( -2.701047200102606016, 12.19889638921340413, -61.34999999999996589 ) ) ;
#34191=CARTESIAN_POINT ( 'NONE',  ( -1.081538986177402961, 23.35243083318996327, -55.04295307432606421 ) ) ;
#34199=CARTESIAN_POINT ( 'NONE',  ( 3.199711850326839357, 14.51624076678035635, -68.24295307432605284 ) ) ;
#34201=CARTESIAN_POINT ( 'NONE',  ( 3.965139115708213868, 19.34895832295540430, -58.65704692567388179 ) ) ;
#34214=CARTESIAN_POINT ( 'NONE',  ( -4.318543150850367773, 18.18399003996480801, -49.94999999999994600 ) ) ;
#34225=CARTESIAN_POINT ( 'NONE',  ( -3.199711850326840246, 20.48375923321962233, -72.74295307432603863 ) ) ;
#34240=CARTESIAN_POINT ( 'NONE',  ( -4.107178604518053611, 16.84948681541050775, -40.79999999999996874 ) ) ;
#34245=CARTESIAN_POINT ( 'NONE',  ( 3.705139346311793869, 15.61213720913094960, -33.59999999999996589 ) ) ;
#34255=CARTESIAN_POINT ( 'NONE',  ( -4.107178604518053611, 16.84948681541050775, -52.79999999999996874 ) ) ;
#34257=CARTESIAN_POINT ( 'NONE',  ( 2.439449611014226971, 12.39241881970633230, -44.40704692567387468 ) ) ;
#34258=CARTESIAN_POINT ( 'NONE',  ( 4.001075405444606048, 21.50107540544455276, -32.99999999999996447 ) ) ;
#34261=CARTESIAN_POINT ( 'NONE',  ( 2.940415233664778416, 20.44041523366473712, -74.99999999999997158 ) ) ;
#34272=CARTESIAN_POINT ( 'NONE',  ( 4.103766977300021601, 21.39838383358913987, -37.50704692567386189 ) ) ;
#34276=CARTESIAN_POINT ( 'NONE',  ( 2.698247469942395949, 12.52428291510489977, -47.39295307432605853 ) ) ;
#34294=CARTESIAN_POINT ( 'NONE',  ( 5.900206406879871857, 16.72010411457162604, -73.94295307432606990 ) ) ;
#34298=CARTESIAN_POINT ( 'NONE',  ( 4.129897239856814117, 18.00707336630801336, -40.80704692567388037 ) ) ;
#34300=CARTESIAN_POINT ( 'NONE',  ( -4.107178604518053611, 16.84948681541050775, -31.79999999999996874 ) ) ;
#34301=CARTESIAN_POINT ( 'NONE',  ( 0.6839900399647733664, 13.18145684914961357, -64.04999999999994031 ) ) ;
#34311=CARTESIAN_POINT ( 'NONE',  ( -1.758463861404912842, 21.27107139401109137, -24.90704692567387823 ) ) ;
#34312=CARTESIAN_POINT ( 'NONE',  ( -5.876318620034919782, 18.43071743580290089, -64.94999999999996021 ) ) ;
#34323=CARTESIAN_POINT ( 'NONE',  ( -0.7798958854283041253, 23.40020640687986386, -67.05704692567387326 ) ) ;
#34328=CARTESIAN_POINT ( 'NONE',  ( -5.041649132594344884, 20.06884854047834921, -26.09999999999996234 ) ) ;
#34345=CARTESIAN_POINT ( 'NONE',  ( 4.206979645153767322, 13.29302035484617051, -51.74999999999994316 ) ) ;
#34350=CARTESIAN_POINT ( 'NONE',  ( -2.121074495332175847, 13.67351099933674341, -71.85704692567388463 ) ) ;
#34351=CARTESIAN_POINT ( 'NONE',  ( 3.705139346311793869, 15.61213720913094960, -57.59999999999997300 ) ) ;
#34358=CARTESIAN_POINT ( 'NONE',  ( -3.091735541773221296, 20.59173554177323950, -74.24999999999997158 ) ) ;
#34363=CARTESIAN_POINT ( 'NONE',  ( -2.017261720333081598, 21.13920729861251857, -36.89295307432605142 ) ) ;
#34366=CARTESIAN_POINT ( 'NONE',  ( 2.017261720333081598, 13.86079270138745834, -50.39295307432605853 ) ) ;
#34380=CARTESIAN_POINT ( 'NONE',  ( 0.8851648821498760977, 23.08871111541074228, -56.69999999999997442 ) ) ;
#34400=CARTESIAN_POINT ( 'NONE',  ( -2.698247469942396837, 22.47571708489507358, -45.89295307432605853 ) ) ;
#34406=CARTESIAN_POINT ( 'NONE',  ( -2.940415233664778860, 14.55958476633523802, -25.49999999999996803 ) ) ;
#34409=CARTESIAN_POINT ( 'NONE',  ( 3.199711850326839357, 14.51624076678035635, -62.24295307432607416 ) ) ;
#34424=CARTESIAN_POINT ( 'NONE',  ( 3.895814058185739448, 19.48501640914375344, -48.14999999999997726 ) ) ;
#34447=CARTESIAN_POINT ( 'NONE',  ( 4.318543150850366885, 16.81600996003516713, -42.44999999999996732 ) ) ;
#34451=CARTESIAN_POINT ( 'NONE',  ( -3.895814058185739448, 15.51498359085620571, -34.64999999999997016 ) ) ;
#34460=CARTESIAN_POINT ( 'NONE',  ( -3.705139346311794313, 19.38786279086902198, -59.09999999999997300 ) ) ;
#34462=CARTESIAN_POINT ( 'NONE',  ( 0.7798958854283032371, 11.59979359312010772, -47.55704692567388037 ) ) ;
#34463=CARTESIAN_POINT ( 'NONE',  ( -0.8851648821498765418, 11.91128888458923285, -40.19999999999996732 ) ) ;
#34466=CARTESIAN_POINT ( 'NONE',  ( 0.6505131845895220088, 21.60717860451803674, -74.69999999999997442 ) ) ;
#34477=CARTESIAN_POINT ( 'NONE',  ( -2.439449611014227859, 22.60758118029364283, -30.90704692567387113 ) ) ;
#34482=CARTESIAN_POINT ( 'NONE',  ( 3.898383833589191383, 21.60376697729997275, -49.49295307432605995 ) ) ;
#34499=CARTESIAN_POINT ( 'NONE',  ( 2.698247469942395949, 12.52428291510489977, -71.39295307432605853 ) ) ;
#34503=CARTESIAN_POINT ( 'NONE',  ( -0.5331684895902242260, 21.84243093769531185, -40.05704692567387326 ) ) ;
#34504=CARTESIAN_POINT ( 'NONE',  ( 3.705139346311793869, 15.61213720913094960, -30.59999999999996589 ) ) ;
#34505=CARTESIAN_POINT ( 'NONE',  ( 2.940415233664778416, 20.44041523366473712, -65.99999999999997158 ) ) ;
#34515=CARTESIAN_POINT ( 'NONE',  ( 2.121074495332174958, 21.32648900066323350, -25.35704692567387042 ) ) ;
#34516=CARTESIAN_POINT ( 'NONE',  ( 5.588711115410763597, 18.38516488214980882, -60.29999999999996163 ) ) ;
#34530=CARTESIAN_POINT ( 'NONE',  ( -5.611429750749524992, 16.75827493613162034, -63.30704692567387326 ) ) ;
#34533=CARTESIAN_POINT ( 'NONE',  ( 5.301103610786608300, 20.20104720010253985, -30.14999999999997016 ) ) ;
#34550=CARTESIAN_POINT ( 'NONE',  ( 5.876318620034919782, 16.56928256419707068, -48.44999999999994600 ) ) ;
#34554=CARTESIAN_POINT ( 'NONE',  ( -4.294655364005415699, 18.33481159033935626, -72.45704692567387895 ) ) ;
#34555=CARTESIAN_POINT ( 'NONE',  ( -1.887862790868997553, 21.20513934631180319, -59.39999999999997016 ) ) ;
#34561=CARTESIAN_POINT ( 'NONE',  ( -3.705139346311794313, 19.38786279086902198, -71.09999999999996589 ) ) ;
#34565=CARTESIAN_POINT ( 'NONE',  ( -4.342430937695320736, 18.03316848959025620, -36.44295307432606279 ) ) ;
#34568=CARTESIAN_POINT ( 'NONE',  ( -4.084459969179292216, 16.70604699712905372, -51.29295307432606421 ) ) ;
#34583=CARTESIAN_POINT ( 'NONE',  ( 2.568848540478311460, 12.45835086740561692, -54.89999999999996305 ) ) ;
#34605=CARTESIAN_POINT ( 'NONE',  ( -1.081538986177402961, 23.35243083318996327, -49.04295307432606421 ) ) ;
#34614=CARTESIAN_POINT ( 'NONE',  ( -3.199711850326840246, 20.48375923321962233, -63.74295307432605995 ) ) ;
#34628=CARTESIAN_POINT ( 'NONE',  ( 2.940415233664778416, 20.44041523366473712, -41.99999999999996447 ) ) ;
#34653=CARTESIAN_POINT ( 'NONE',  ( -0.6839900399647738105, 21.81854315085035623, -26.54999999999996163 ) ) ;
#34657=CARTESIAN_POINT ( 'NONE',  ( -0.6505131845895224529, 13.39282139548194195, -40.19999999999996732 ) ) ;
#34666=CARTESIAN_POINT ( 'NONE',  ( -2.940415233664778860, 14.55958476633523802, -58.49999999999997158 ) ) ;
#34668=CARTESIAN_POINT ( 'NONE',  ( -0.7798958854283041253, 23.40020640687986386, -43.05704692567387326 ) ) ;
#34669=CARTESIAN_POINT ( 'NONE',  ( -4.001075405444606936, 13.49892459455542060, -37.49999999999996447 ) ) ;
#34670=CARTESIAN_POINT ( 'NONE',  ( 0.7417250638684235176, 23.11142975074950101, -40.19295307432605568 ) ) ;
#34673=CARTESIAN_POINT ( 'NONE',  ( 0.6839900399647733664, 13.18145684914961357, -73.04999999999998295 ) ) ;
#34685=CARTESIAN_POINT ( 'NONE',  ( 5.370428668309080500, 20.06498911391418360, -28.65704692567387468 ) ) ;
#34689=CARTESIAN_POINT ( 'NONE',  ( -1.081538986177402961, 23.35243083318996327, -43.04295307432605711 ) ) ;
#34708=CARTESIAN_POINT ( 'NONE',  ( 4.314955953707388936, 13.40099666339979123, -71.24295307432605284 ) ) ;
#34712=CARTESIAN_POINT ( 'NONE',  ( -0.6505131845895224529, 13.39282139548194195, -34.19999999999996732 ) ) ;
#34713=CARTESIAN_POINT ( 'NONE',  ( -3.705139346311794313, 19.38786279086902198, -65.09999999999996589 ) ) ;
#34723=CARTESIAN_POINT ( 'NONE',  ( -2.439449611014227859, 22.60758118029364283, -72.90704692567388179 ) ) ;
#34724=CARTESIAN_POINT ( 'NONE',  ( 4.001075405444606048, 21.50107540544455276, -62.99999999999997158 ) ) ;
#34737=CARTESIAN_POINT ( 'NONE',  ( 4.103766977300021601, 21.39838383358913987, -52.50704692567387610 ) ) ;
#34741=CARTESIAN_POINT ( 'NONE',  ( -5.301103610786608300, 14.79895279989743706, -25.64999999999996305 ) ) ;
#34757=CARTESIAN_POINT ( 'NONE',  ( -4.001075405444606936, 13.49892459455542060, -52.49999999999996447 ) ) ;
#34762=CARTESIAN_POINT ( 'NONE',  ( 2.983759233219601459, 14.30028814967311668, -71.25704692567387610 ) ) ;
#34763=CARTESIAN_POINT ( 'NONE',  ( -3.895814058185739892, 15.51498359085620748, -61.64999999999996305 ) ) ;
#34774=CARTESIAN_POINT ( 'NONE',  ( 2.940415233664778416, 20.44041523366473712, -71.99999999999997158 ) ) ;
#34777=CARTESIAN_POINT ( 'NONE',  ( 3.199711850326839357, 14.51624076678035635, -41.24295307432605284 ) ) ;
#34795=CARTESIAN_POINT ( 'NONE',  ( -4.206979645153768210, 21.70697964515380107, -59.24999999999997158 ) ) ;
#34818=CARTESIAN_POINT ( 'NONE',  ( 3.898383833589191383, 21.60376697729997275, -49.49295307432605995 ) ) ;
#34826=CARTESIAN_POINT ( 'NONE',  ( -0.8348115903393239501, 21.79465536400541126, -64.04295307432605000 ) ) ;
#34839=CARTESIAN_POINT ( 'NONE',  ( -3.091735541773221296, 20.59173554177323950, -50.24999999999997158 ) ) ;
#34863=CARTESIAN_POINT ( 'NONE',  ( 3.091735541773220852, 14.40826445822673740, -33.74999999999996447 ) ) ;
#34871=CARTESIAN_POINT ( 'NONE',  ( -2.983759233219601903, 20.69971185032686023, -69.75704692567386189 ) ) ;
#34880=CARTESIAN_POINT ( 'NONE',  ( 4.318543150850367773, 16.81600996003516357, -60.44999999999997442 ) ) ;
#34882=CARTESIAN_POINT ( 'NONE',  ( -4.103766977300021601, 13.60161616641083704, -51.00704692567387610 ) ) ;
#34883=CARTESIAN_POINT ( 'NONE',  ( -5.301103610786608300, 14.79895279989743528, -28.64999999999995950 ) ) ;
#34884=CARTESIAN_POINT ( 'NONE',  ( 4.107178604518054499, 18.15051318458946383, -72.29999999999996874 ) ) ;
#34894=CARTESIAN_POINT ( 'NONE',  ( -5.370428668309080500, 14.93501088608579153, -30.15704692567386758 ) ) ;
#34899=CARTESIAN_POINT ( 'NONE',  ( -5.107581180293630396, 19.93944961101426827, -39.59295307432606137 ) ) ;
#34917=CARTESIAN_POINT ( 'NONE',  ( -5.900206406879871857, 18.27989588542834554, -60.44295307432605568 ) ) ;
#34922=CARTESIAN_POINT ( 'NONE',  ( -3.705139346311794313, 19.38786279086902198, -38.09999999999996589 ) ) ;
#34923=CARTESIAN_POINT ( 'NONE',  ( 3.091735541773220852, 14.40826445822673563, -63.74999999999997868 ) ) ;
#34933=CARTESIAN_POINT ( 'NONE',  ( -3.639207298612509689, 19.51726172033310647, -24.60704692567387397 ) ) ;
#34934=CARTESIAN_POINT ( 'NONE',  ( 5.041649132594343996, 14.93115145952162415, -60.59999999999996589 ) ) ;
#34936=DIRECTION ( 'NONE',  ( -0.7071067811865510144, -0.7071067811865440200, 0.000000000000000000 ) ) ;
#34947=CARTESIAN_POINT ( 'NONE',  ( 4.099003336600150149, 13.18504404629255689, -56.25704692567388321 ) ) ;
#34950=CARTESIAN_POINT ( 'NONE',  ( 2.564989113914249330, 22.87042866830903876, -67.34295307432606137 ) ) ;
#34973=CARTESIAN_POINT ( 'NONE',  ( 5.041649132594343996, 14.93115145952162415, -48.59999999999996589 ) ) ;
#34977=CARTESIAN_POINT ( 'NONE',  ( 0.7939530028709752552, 21.58445996917927445, -58.20704692567387184 ) ) ;
#34978=CARTESIAN_POINT ( 'NONE',  ( -3.705139346311794313, 19.38786279086902198, -59.09999999999997300 ) ) ;
#34985=CARTESIAN_POINT ( 'NONE',  ( 1.887862790868997109, 13.79486065368817194, -69.89999999999996305 ) ) ;
#34987=CARTESIAN_POINT ( 'NONE',  ( 4.294655364005415699, 16.66518840966061887, -52.95704692567387895 ) ) ;
#34990=CARTESIAN_POINT ( 'NONE',  ( -4.318543150850367773, 18.18399003996480801, -70.94999999999997442 ) ) ;
#34993=CARTESIAN_POINT ( 'NONE',  ( 1.848958322955461808, 21.46513911570817612, -46.34295307432606137 ) ) ;
#35009=CARTESIAN_POINT ( 'NONE',  ( 5.876318620034919782, 16.56928256419707068, -48.44999999999994600 ) ) ;
#35028=CARTESIAN_POINT ( 'NONE',  ( -0.6839900399647736995, 21.81854315085035623, -47.54999999999997584 ) ) ;
#35029=CARTESIAN_POINT ( 'NONE',  ( 2.564989113914249330, 22.87042866830903876, -46.34295307432606137 ) ) ;
#35038=CARTESIAN_POINT ( 'NONE',  ( -0.5070733663080690956, 13.37010276014318144, -59.69295307432605568 ) ) ;
#35052=CARTESIAN_POINT ( 'NONE',  ( -3.705139346311794313, 19.38786279086902198, -32.09999999999996589 ) ) ;
#35078=CARTESIAN_POINT ( 'NONE',  ( -2.940415233664778860, 14.55958476633523802, -28.49999999999996447 ) ) ;
#35081=CARTESIAN_POINT ( 'NONE',  ( -5.565992480072003978, 16.47139529956871229, -33.29295307432605711 ) ) ;
#35082=CARTESIAN_POINT ( 'NONE',  ( 1.985016409143818272, 21.39581405818570303, -26.84999999999995524 ) ) ;
#35090=CARTESIAN_POINT ( 'NONE',  ( -4.107178604518053611, 16.84948681541050775, -58.79999999999996163 ) ) ;
#35093=CARTESIAN_POINT ( 'NONE',  ( 2.837105286290961370, 22.73177855326409613, -40.35704692567387752 ) ) ;
#35094=CARTESIAN_POINT ( 'NONE',  ( 4.206979645153768210, 13.29302035484617406, -30.74999999999996092 ) ) ;
#35095=CARTESIAN_POINT ( 'NONE',  ( 2.940415233664778416, 20.44041523366473712, -71.99999999999997158 ) ) ;
#35106=CARTESIAN_POINT ( 'NONE',  ( -5.876318620034919782, 18.43071743580290089, -73.94999999999997442 ) ) ;
#35110=CARTESIAN_POINT ( 'NONE',  ( 0.7417250638684235176, 23.11142975074950101, -43.19295307432606279 ) ) ;
#35127=CARTESIAN_POINT ( 'NONE',  ( -5.231778553264134324, 14.66289471370907727, -63.14295307432606563 ) ) ;
#35132=CARTESIAN_POINT ( 'NONE',  ( 0.6505131845895220088, 21.60717860451803674, -32.69999999999996732 ) ) ;
#35133=CARTESIAN_POINT ( 'NONE',  ( -0.6505131845895224529, 13.39282139548194195, -55.19999999999997442 ) ) ;
#35144=CARTESIAN_POINT ( 'NONE',  ( -4.294655364005415699, 18.33481159033935626, -30.45704692567387184 ) ) ;
#35145=CARTESIAN_POINT ( 'NONE',  ( 2.701047200102605128, 22.80110361078656211, -50.84999999999996589 ) ) ;
#35156=CARTESIAN_POINT ( 'NONE',  ( 2.837105286290961370, 22.73177855326409613, -58.35704692567387752 ) ) ;
#35159=CARTESIAN_POINT ( 'NONE',  ( 2.698247469942395949, 12.52428291510489977, -71.39295307432605853 ) ) ;
#35174=CARTESIAN_POINT ( 'NONE',  ( 5.588711115410763597, 18.38516488214980882, -45.29999999999996874 ) ) ;
#35178=CARTESIAN_POINT ( 'NONE',  ( 3.043106805520193525, 20.33772366180932067, -64.50704692567389031 ) ) ;
#35179=CARTESIAN_POINT ( 'NONE',  ( 4.318543150850366885, 16.81600996003516713, -54.44999999999996021 ) ) ;
#35186=CARTESIAN_POINT ( 'NONE',  ( -3.091735541773221296, 20.59173554177323950, -68.24999999999995737 ) ) ;
#35188=CARTESIAN_POINT ( 'NONE',  ( -0.7939530028709754772, 13.41554003082070246, -53.70704692567388605 ) ) ;
#35191=CARTESIAN_POINT ( 'NONE',  ( -3.826489000663265472, 15.37892550466785480, -27.14295307432605853 ) ) ;
#35194=CARTESIAN_POINT ( 'NONE',  ( -1.848958322955462474, 13.53486088429179546, -44.84295307432606137 ) ) ;
#35211=CARTESIAN_POINT ( 'NONE',  ( -5.301103610786608300, 14.79895279989743706, -52.64999999999997016 ) ) ;
#35228=CARTESIAN_POINT ( 'NONE',  ( 4.001075405444606048, 21.50107540544455276, -68.99999999999995737 ) ) ;
#35233=CARTESIAN_POINT ( 'NONE',  ( -1.985016409143819605, 13.60418594181426855, -40.34999999999996589 ) ) ;
#35234=CARTESIAN_POINT ( 'NONE',  ( -5.900206406879871857, 18.27989588542834554, -42.44295307432605568 ) ) ;
#35242=CARTESIAN_POINT ( 'NONE',  ( -0.8348115903393239501, 21.79465536400541126, -55.04295307432606421 ) ) ;
#35258=CARTESIAN_POINT ( 'NONE',  ( -1.985016409143819605, 13.60418594181426855, -40.34999999999996589 ) ) ;
#35285=CARTESIAN_POINT ( 'NONE',  ( 2.983759233219601459, 14.30028814967311668, -44.25704692567387610 ) ) ;
#35287=CARTESIAN_POINT ( 'NONE',  ( -1.887862790868997553, 21.20513934631180319, -29.39999999999996660 ) ) ;
#35291=CARTESIAN_POINT ( 'NONE',  ( -3.898383833589191827, 13.39623302270000771, -32.99295307432605995 ) ) ;
#35292=CARTESIAN_POINT ( 'NONE',  ( -2.121074495332175847, 13.67351099933674341, -71.85704692567388463 ) ) ;
#35299=CARTESIAN_POINT ( 'NONE',  ( 3.705139346311793869, 15.61213720913094960, -42.59999999999996589 ) ) ;
#35303=CARTESIAN_POINT ( 'NONE',  ( -5.370428668309080500, 14.93501088608579153, -33.15704692567386047 ) ) ;
#35305=CARTESIAN_POINT ( 'NONE',  ( 4.107178604518054499, 18.15051318458946383, -69.29999999999996874 ) ) ;
#35315=CARTESIAN_POINT ( 'NONE',  ( -1.028604700431329233, 11.93400751992799513, -26.70704692567387539 ) ) ;
#35320=CARTESIAN_POINT ( 'NONE',  ( -5.231778553264134324, 14.66289471370907727, -45.14295307432605853 ) ) ;
#35335=CARTESIAN_POINT ( 'NONE',  ( -2.698247469942396837, 22.47571708489507358, -60.89295307432605853 ) ) ;
#35340=CARTESIAN_POINT ( 'NONE',  ( -3.091735541773221296, 20.59173554177323950, -26.24999999999996803 ) ) ;
#35341=CARTESIAN_POINT ( 'NONE',  ( -1.985016409143819605, 13.60418594181426855, -58.34999999999995879 ) ) ;
#35355=CARTESIAN_POINT ( 'NONE',  ( -5.611429750749524992, 16.75827493613162034, -66.30704692567387326 ) ) ;
#35356=CARTESIAN_POINT ( 'NONE',  ( -4.001075405444606936, 13.49892459455542060, -58.49999999999997158 ) ) ;
#35367=CARTESIAN_POINT ( 'NONE',  ( -0.7798958854283041253, 23.40020640687986386, -58.05704692567386616 ) ) ;
#35371=CARTESIAN_POINT ( 'NONE',  ( -4.314955953707389824, 21.59900333660018390, -72.74295307432603863 ) ) ;
#35387=CARTESIAN_POINT ( 'NONE',  ( -5.041649132594344884, 20.06884854047834921, -41.09999999999996589 ) ) ;
#35391=CARTESIAN_POINT ( 'NONE',  ( -0.7939530028709754772, 13.41554003082070246, -59.70704692567387184 ) ) ;
#35392=CARTESIAN_POINT ( 'NONE',  ( -0.6839900399647738105, 21.81854315085035623, -47.54999999999996874 ) ) ;
#35402=CARTESIAN_POINT ( 'NONE',  ( -4.318543150850367773, 18.18399003996480801, -64.94999999999996021 ) ) ;
#35405=CARTESIAN_POINT ( 'NONE',  ( 3.043106805520193525, 20.33772366180932067, -40.50704692567387610 ) ) ;
#35410=CARTESIAN_POINT ( 'NONE',  ( 0.5070733663080689846, 21.62989723985679902, -49.19295307432605568 ) ) ;
#35425=CARTESIAN_POINT ( 'NONE',  ( -2.568848540478311904, 22.54164913259435465, -50.39999999999996305 ) ) ;
#35441=CARTESIAN_POINT ( 'NONE',  ( 5.588711115410763597, 18.38516488214980882, -66.29999999999996874 ) ) ;
#35446=CARTESIAN_POINT ( 'NONE',  ( -0.6505131845895224529, 13.39282139548194195, -43.19999999999996732 ) ) ;
#35457=CARTESIAN_POINT ( 'NONE',  ( 4.342430937695320736, 16.96683151040971538, -52.94295307432605568 ) ) ;
#35474=CARTESIAN_POINT ( 'NONE',  ( 2.940415233664778416, 20.44041523366473712, -38.99999999999996447 ) ) ;
#35501=CARTESIAN_POINT ( 'NONE',  ( -1.758463861404912842, 21.27107139401109137, -36.90704692567386758 ) ) ;
#35505=CARTESIAN_POINT ( 'NONE',  ( -5.231778553264134324, 14.66289471370907727, -36.14295307432605142 ) ) ;
#35506=CARTESIAN_POINT ( 'NONE',  ( -3.091735541773221296, 20.59173554177323950, -26.24999999999996803 ) ) ;
#35514=CARTESIAN_POINT ( 'NONE',  ( -3.895814058185739448, 15.51498359085620571, -46.64999999999994884 ) ) ;
#35518=CARTESIAN_POINT ( 'NONE',  ( -4.103766977300021601, 13.60161616641083704, -39.00704692567386900 ) ) ;
#35520=CARTESIAN_POINT ( 'NONE',  ( -4.107178604518053611, 16.84948681541050775, -61.79999999999996874 ) ) ;
#35532=CARTESIAN_POINT ( 'NONE',  ( 5.565992480072003978, 18.52860470043125574, -37.79295307432605711 ) ) ;
#35548=CARTESIAN_POINT ( 'NONE',  ( -2.698247469942396837, 22.47571708489507358, -66.89295307432607274 ) ) ;
#35554=CARTESIAN_POINT ( 'NONE',  ( -4.107178604518053611, 16.84948681541050775, -58.79999999999996163 ) ) ;
#35565=CARTESIAN_POINT ( 'NONE',  ( 5.852430833189966819, 16.41846101382252243, -64.95704692567387895 ) ) ;
#35566=CARTESIAN_POINT ( 'NONE',  ( -5.876318620034919782, 18.43071743580290089, -52.94999999999996021 ) ) ;
#35579=CARTESIAN_POINT ( 'NONE',  ( 1.028604700431328567, 23.06599248007198355, -55.20704692567388605 ) ) ;
#35583=CARTESIAN_POINT ( 'NONE',  ( 1.081538986177402295, 11.64756916681001186, -74.54295307432605000 ) ) ;
#35603=CARTESIAN_POINT ( 'NONE',  ( -5.588711115410763597, 16.61483511785016987, -46.79999999999996874 ) ) ;
#35606=CARTESIAN_POINT ( 'NONE',  ( -2.121074495332175847, 13.67351099933674341, -65.85704692567387042 ) ) ;
#35607=CARTESIAN_POINT ( 'NONE',  ( -4.318543150850366885, 18.18399003996480801, -52.94999999999996021 ) ) ;
#35616=CARTESIAN_POINT ( 'NONE',  ( 0.6839900399647733664, 13.18145684914961357, -61.04999999999995453 ) ) ;
#35618=CARTESIAN_POINT ( 'NONE',  ( 2.983759233219601459, 14.30028814967311668, -44.25704692567387610 ) ) ;
#35623=CARTESIAN_POINT ( 'NONE',  ( 4.084459969179292216, 18.29395300287091430, -43.79295307432606421 ) ) ;
#35638=CARTESIAN_POINT ( 'NONE',  ( 5.588711115410763597, 18.38516488214980882, -51.29999999999996874 ) ) ;
#35654=CARTESIAN_POINT ( 'NONE',  ( 5.301103610786608300, 20.20104720010253985, -69.14999999999994884 ) ) ;
#35659=CARTESIAN_POINT ( 'NONE',  ( 2.940415233664778416, 20.44041523366473712, -47.99999999999996447 ) ) ;
#35672=CARTESIAN_POINT ( 'NONE',  ( 1.848958322955461808, 21.46513911570817612, -55.34295307432606137 ) ) ;
#35680=CARTESIAN_POINT ( 'NONE',  ( -2.837105286290963146, 12.26822144673588255, -38.85704692567387752 ) ) ;
#35689=CARTESIAN_POINT ( 'NONE',  ( 3.091735541773220852, 14.40826445822673563, -39.74999999999996447 ) ) ;
#35712=CARTESIAN_POINT ( 'NONE',  ( -3.639207298612509689, 19.51726172033310647, -30.60704692567387752 ) ) ;
#35716=CARTESIAN_POINT ( 'NONE',  ( 5.231778553264135212, 20.33710528629089254, -37.64295307432604432 ) ) ;
#35717=CARTESIAN_POINT ( 'NONE',  ( -0.6839900399647736995, 21.81854315085035623, -26.54999999999996163 ) ) ;
#35724=CARTESIAN_POINT ( 'NONE',  ( 3.091735541773220852, 14.40826445822673563, -42.74999999999996447 ) ) ;
#35727=CARTESIAN_POINT ( 'NONE',  ( -0.7798958854283041253, 23.40020640687986386, -37.05704692567387326 ) ) ;
#35729=CARTESIAN_POINT ( 'NONE',  ( -1.887862790868997553, 21.20513934631180319, -65.39999999999997726 ) ) ;
#35743=CARTESIAN_POINT ( 'NONE',  ( 4.314955953707388936, 13.40099666339979123, -29.24295307432605640 ) ) ;
#35762=CARTESIAN_POINT ( 'NONE',  ( -3.895814058185739448, 15.51498359085620571, -55.64999999999994174 ) ) ;
#35771=CARTESIAN_POINT ( 'NONE',  ( 2.837105286290961370, 22.73177855326409613, -64.35704692567387042 ) ) ;
#35772=CARTESIAN_POINT ( 'NONE',  ( 2.568848540478311460, 12.45835086740561692, -57.89999999999996305 ) ) ;
#35784=CARTESIAN_POINT ( 'NONE',  ( -1.028604700431329233, 11.93400751992799513, -44.70704692567387184 ) ) ;
#35789=CARTESIAN_POINT ( 'NONE',  ( -5.900206406879871857, 18.27989588542834554, -69.44295307432605568 ) ) ;
#35802=CARTESIAN_POINT ( 'NONE',  ( -5.876318620034919782, 18.43071743580290089, -40.94999999999996732 ) ) ;
#35805=CARTESIAN_POINT ( 'NONE',  ( 3.043106805520193525, 20.33772366180932067, -58.50704692567387610 ) ) ;
#35806=CARTESIAN_POINT ( 'NONE',  ( 2.940415233664778416, 20.44041523366473712, -44.99999999999997158 ) ) ;
#35816=CARTESIAN_POINT ( 'NONE',  ( -3.091735541773221296, 20.59173554177323950, -65.24999999999995737 ) ) ;
#35819=CARTESIAN_POINT ( 'NONE',  ( 4.294655364005415699, 16.66518840966061887, -49.95704692567387184 ) ) ;
#35823=CARTESIAN_POINT ( 'NONE',  ( -0.5070733663080690956, 13.37010276014318144, -32.69295307432605568 ) ) ;
#35837=CARTESIAN_POINT ( 'NONE',  ( -2.701047200102606016, 12.19889638921340413, -49.34999999999996589 ) ) ;
#35851=CARTESIAN_POINT ( 'NONE',  ( 4.206979645153767322, 13.29302035484617051, -72.74999999999995737 ) ) ;
#35856=CARTESIAN_POINT ( 'NONE',  ( -3.091735541773221296, 20.59173554177323950, -41.24999999999995026 ) ) ;
#35867=CARTESIAN_POINT ( 'NONE',  ( 0.5070733663080689846, 21.62989723985679902, -58.19295307432606279 ) ) ;
#35873=CARTESIAN_POINT ( 'NONE',  ( -3.826489000663265472, 15.37892550466785480, -60.14295307432605142 ) ) ;
#35885=CARTESIAN_POINT ( 'NONE',  ( 3.091735541773220852, 14.40826445822673563, -36.74999999999994316 ) ) ;
#35910=CARTESIAN_POINT ( 'NONE',  ( -4.294655364005415699, 18.33481159033935626, -33.45704692567387895 ) ) ;
#35914=CARTESIAN_POINT ( 'NONE',  ( 5.107581180293630396, 15.06055038898570686, -35.09295307432605426 ) ) ;
#35915=CARTESIAN_POINT ( 'NONE',  ( 3.965139115708213868, 19.34895832295540430, -61.65704692567387468 ) ) ;
#35922=CARTESIAN_POINT ( 'NONE',  ( -2.940415233664778860, 14.55958476633523802, -46.49999999999997158 ) ) ;
#35926=CARTESIAN_POINT ( 'NONE',  ( -4.103766977300021601, 13.60161616641083704, -42.00704692567387610 ) ) ;
#35929=CARTESIAN_POINT ( 'NONE',  ( 0.6839900399647733664, 13.18145684914961357, -61.04999999999995453 ) ) ;
#35941=CARTESIAN_POINT ( 'NONE',  ( -5.900206406879871857, 18.27989588542834554, -27.44295307432605568 ) ) ;
#35961=CARTESIAN_POINT ( 'NONE',  ( 3.091735541773220852, 14.40826445822673563, -51.74999999999994316 ) ) ;
#35969=CARTESIAN_POINT ( 'NONE',  ( -3.705139346311794313, 19.38786279086902198, -74.09999999999996589 ) ) ;
#35971=CARTESIAN_POINT ( 'NONE',  ( 5.611429750749524992, 18.24172506386835479, -67.80704692567387326 ) ) ;
#35972=CARTESIAN_POINT ( 'NONE',  ( 2.701047200102605128, 22.80110361078656211, -53.84999999999995879 ) ) ;
#35983=CARTESIAN_POINT ( 'NONE',  ( -5.370428668309080500, 14.93501088608579153, -48.15704692567388179 ) ) ;
#35989=CARTESIAN_POINT ( 'NONE',  ( 4.314955953707388936, 13.40099666339979123, -62.24295307432607416 ) ) ;
#36005=CARTESIAN_POINT ( 'NONE',  ( -2.701047200102606016, 12.19889638921340413, -40.34999999999996589 ) ) ;
#36008=CARTESIAN_POINT ( 'NONE',  ( 4.129897239856814117, 18.00707336630801336, -49.80704692567388037 ) ) ;
#36010=CARTESIAN_POINT ( 'NONE',  ( -4.107178604518053611, 16.84948681541050775, -49.79999999999996874 ) ) ;
#36020=CARTESIAN_POINT ( 'NONE',  ( -0.6839900399647736995, 21.81854315085035623, -62.54999999999996874 ) ) ;
#36022=CARTESIAN_POINT ( 'NONE',  ( -3.639207298612509689, 19.51726172033310647, -45.60704692567387752 ) ) ;
#36027=CARTESIAN_POINT ( 'NONE',  ( 3.199711850326839357, 14.51624076678035635, -38.24295307432604574 ) ) ;
#36033=CARTESIAN_POINT ( 'NONE',  ( -0.7939530028709754772, 13.41554003082070246, -26.70704692567387539 ) ) ;
#36038=CARTESIAN_POINT ( 'NONE',  ( -5.588711115410763597, 16.61483511785016987, -34.79999999999996163 ) ) ;
#36057=CARTESIAN_POINT ( 'NONE',  ( -5.876318620034919782, 18.43071743580290089, -70.94999999999997442 ) ) ;
#36063=CARTESIAN_POINT ( 'NONE',  ( 3.091735541773220852, 14.40826445822673563, -33.74999999999996447 ) ) ;
#36075=CARTESIAN_POINT ( 'NONE',  ( 2.837723661809363307, 20.54310680552015356, -49.49295307432605995 ) ) ;
#36080=CARTESIAN_POINT ( 'NONE',  ( -0.8348115903393239501, 21.79465536400541126, -64.04295307432605000 ) ) ;
#36098=CARTESIAN_POINT ( 'NONE',  ( 4.001075405444606048, 21.50107540544455276, -74.99999999999997158 ) ) ;
#36118=CARTESIAN_POINT ( 'NONE',  ( -4.129897239856814117, 16.99292663369196177, -36.30704692567387326 ) ) ;
#36122=CARTESIAN_POINT ( 'NONE',  ( 5.231778553264135212, 20.33710528629089254, -28.64295307432606208 ) ) ;
#36123=CARTESIAN_POINT ( 'NONE',  ( 3.639207298612508801, 15.48273827966686866, -62.10704692567388463 ) ) ;
#36130=CARTESIAN_POINT ( 'NONE',  ( 4.318543150850367773, 16.81600996003516357, -48.44999999999994600 ) ) ;
#36133=CARTESIAN_POINT ( 'NONE',  ( 4.099003336600150149, 13.18504404629255689, -32.25704692567387610 ) ) ;
#36135=CARTESIAN_POINT ( 'NONE',  ( -4.107178604518053611, 16.84948681541050775, -55.79999999999996874 ) ) ;
#36148=CARTESIAN_POINT ( 'NONE',  ( 5.107581180293630396, 15.06055038898570686, -29.09295307432605782 ) ) ;
#36168=CARTESIAN_POINT ( 'NONE',  ( 4.318543150850367773, 16.81600996003516357, -48.44999999999994600 ) ) ;
#36176=CARTESIAN_POINT ( 'NONE',  ( 0.6505131845895220088, 21.60717860451803674, -74.69999999999997442 ) ) ;
#36178=CARTESIAN_POINT ( 'NONE',  ( 0.7798958854283032371, 11.59979359312010772, -56.55704692567387326 ) ) ;
#36179=CARTESIAN_POINT ( 'NONE',  ( -5.041649132594344884, 20.06884854047834921, -50.09999999999996589 ) ) ;
#36193=CARTESIAN_POINT ( 'NONE',  ( 5.852430833189966819, 16.41846101382252243, -40.95704692567387184 ) ) ;
#36197=CARTESIAN_POINT ( 'NONE',  ( -5.231778553264134324, 14.66289471370907727, -63.14295307432606563 ) ) ;
#36213=CARTESIAN_POINT ( 'NONE',  ( -4.206979645153768210, 21.70697964515380107, -32.24999999999996447 ) ) ;
#36216=CARTESIAN_POINT ( 'NONE',  ( -0.5331684895902242260, 21.84243093769531185, -52.05704692567388747 ) ) ;
#36217=CARTESIAN_POINT ( 'NONE',  ( -0.6505131845895224529, 13.39282139548194195, -37.19999999999996732 ) ) ;
#36229=CARTESIAN_POINT ( 'NONE',  ( 1.985016409143818272, 21.39581405818570303, -56.84999999999995879 ) ) ;
#36231=CARTESIAN_POINT ( 'NONE',  ( -1.758463861404912842, 21.27107139401109137, -48.90704692567388179 ) ) ;
#36235=CARTESIAN_POINT ( 'NONE',  ( -3.826489000663265472, 15.37892550466785480, -36.14295307432605142 ) ) ;
#36243=CARTESIAN_POINT ( 'NONE',  ( -3.043106805520194413, 14.66227633819065623, -24.00704692567387610 ) ) ;
#36250=CARTESIAN_POINT ( 'NONE',  ( -4.001075405444606936, 13.49892459455542060, -34.49999999999997158 ) ) ;
#36271=CARTESIAN_POINT ( 'NONE',  ( 4.001075405444606048, 21.50107540544455276, -56.99999999999996447 ) ) ;
#36276=CARTESIAN_POINT ( 'NONE',  ( -4.318543150850367773, 18.18399003996480801, -37.94999999999996021 ) ) ;
#36288=CARTESIAN_POINT ( 'NONE',  ( -2.837723661809363751, 14.45689319447982335, -44.99295307432606705 ) ) ;
#36293=CARTESIAN_POINT ( 'NONE',  ( 2.017261720333081598, 13.86079270138745834, -62.39295307432605853 ) ) ;
#36305=CARTESIAN_POINT ( 'NONE',  ( -1.887862790868997553, 21.20513934631180319, -29.39999999999996660 ) ) ;
#36314=CARTESIAN_POINT ( 'NONE',  ( -4.206979645153768210, 21.70697964515380107, -68.24999999999995737 ) ) ;
#36331=CARTESIAN_POINT ( 'NONE',  ( -3.898383833589191827, 13.39623302270000771, -68.99295307432605284 ) ) ;
#36341=CARTESIAN_POINT ( 'NONE',  ( 5.565992480072003978, 18.52860470043125574, -28.79295307432605355 ) ) ;
#36342=CARTESIAN_POINT ( 'NONE',  ( 2.983759233219601459, 14.30028814967311668, -68.25704692567387610 ) ) ;
#36352=CARTESIAN_POINT ( 'NONE',  ( -4.318543150850367773, 18.18399003996480801, -40.94999999999996732 ) ) ;
#36355=CARTESIAN_POINT ( 'NONE',  ( -1.028604700431329233, 11.93400751992799513, -26.70704692567387539 ) ) ;
#36357=CARTESIAN_POINT ( 'NONE',  ( 0.6839900399647733664, 13.18145684914961357, -55.04999999999995453 ) ) ;
#36372=CARTESIAN_POINT ( 'NONE',  ( 2.698247469942395949, 12.52428291510489977, -32.39295307432605142 ) ) ;
#36390=CARTESIAN_POINT ( 'NONE',  ( -3.091735541773221296, 20.59173554177323950, -44.24999999999997868 ) ) ;
#36400=CARTESIAN_POINT ( 'NONE',  ( 3.091735541773220852, 14.40826445822673563, -69.74999999999997158 ) ) ;
#36402=CARTESIAN_POINT ( 'NONE',  ( 5.611429750749524992, 18.24172506386835479, -55.80704692567388037 ) ) ;
#36403=CARTESIAN_POINT ( 'NONE',  ( 4.001075405444606048, 21.50107540544455276, -41.99999999999996447 ) ) ;
#36417=CARTESIAN_POINT ( 'NONE',  ( 0.7798958854283032371, 11.59979359312010772, -47.55704692567388037 ) ) ;
#36422=CARTESIAN_POINT ( 'NONE',  ( 5.900206406879871857, 16.72010411457162604, -61.94295307432605568 ) ) ;
#36436=CARTESIAN_POINT ( 'NONE',  ( -4.001075405444606936, 13.49892459455542060, -34.49999999999997158 ) ) ;
#36440=CARTESIAN_POINT ( 'NONE',  ( -3.965139115708213868, 15.65104167704456906, -57.15704692567387468 ) ) ;
#36441=CARTESIAN_POINT ( 'NONE',  ( -0.6505131845895224529, 13.39282139548194195, -40.19999999999996732 ) ) ;
#36442=CARTESIAN_POINT ( 'NONE',  ( 3.470745319554692454, 20.97074531955464494, -74.99999999999997158 ) ) ;
#36450=CARTESIAN_POINT ( 'NONE',  ( -4.318543150850367773, 18.18399003996480801, -49.94999999999994600 ) ) ;
#36452=CARTESIAN_POINT ( 'NONE',  ( -0.5331684895902242260, 21.84243093769531185, -31.05704692567387681 ) ) ;
#36456=CARTESIAN_POINT ( 'NONE',  ( -3.199711850326840246, 20.48375923321962233, -33.74295307432605995 ) ) ;
#36463=CARTESIAN_POINT ( 'NONE',  ( 4.099003336600150149, 13.18504404629255689, -71.25704692567387610 ) ) ;
#36470=CARTESIAN_POINT ( 'NONE',  ( -2.701047200102606016, 12.19889638921340413, -43.34999999999994458 ) ) ;
#36487=CARTESIAN_POINT ( 'NONE',  ( -4.206979645153768210, 21.70697964515380107, -59.24999999999997158 ) ) ;
#36492=CARTESIAN_POINT ( 'NONE',  ( 4.107178604518054499, 18.15051318458946383, -36.29999999999996163 ) ) ;
#36493=CARTESIAN_POINT ( 'NONE',  ( 3.705139346311793869, 15.61213720913094960, -66.59999999999996589 ) ) ;
#36495=PRODUCT_DEFINITION_CONTEXT ( 'detailed design', #21196, 'design' ) ;
#36505=CARTESIAN_POINT ( 'NONE',  ( -2.837723661809363751, 14.45689319447982335, -41.99295307432605995 ) ) ;
#36509=CARTESIAN_POINT ( 'NONE',  ( 2.017261720333081598, 13.86079270138745834, -68.39295307432607274 ) ) ;
#36519=CARTESIAN_POINT ( 'NONE',  ( 1.887862790868997109, 13.79486065368817194, -27.89999999999996660 ) ) ;
#36527=CARTESIAN_POINT ( 'NONE',  ( -0.9307174358028533767, 23.37631862003491889, -65.54999999999996874 ) ) ;
#36540=CARTESIAN_POINT ( 'NONE',  ( -4.001075405444606936, 13.49892459455542060, -25.49999999999996803 ) ) ;
#36545=CARTESIAN_POINT ( 'NONE',  ( -5.565992480072003978, 16.47139529956871229, -51.29295307432606421 ) ) ;
#36554=CARTESIAN_POINT ( 'NONE',  ( 5.107581180293630396, 15.06055038898570686, -29.09295307432605782 ) ) ;
#36556=CARTESIAN_POINT ( 'NONE',  ( -4.294655364005415699, 18.33481159033935626, -66.45704692567387895 ) ) ;
#36568=CARTESIAN_POINT ( 'NONE',  ( 2.837105286290961370, 22.73177855326409613, -31.35704692567387042 ) ) ;
#36570=CARTESIAN_POINT ( 'NONE',  ( -0.6505131845895224529, 13.39282139548194195, -52.19999999999996732 ) ) ;
#36580=CARTESIAN_POINT ( 'NONE',  ( 5.900206406879871857, 16.72010411457162604, -31.94295307432605568 ) ) ;
#36603=DIRECTION ( 'NONE',  ( 0.7071067811865513475, 0.7071067811865437980, 0.000000000000000000 ) ) ;
#36604=CARTESIAN_POINT ( 'NONE',  ( -4.318543150850367773, 18.18399003996480801, -40.94999999999996732 ) ) ;
#36614=CARTESIAN_POINT ( 'NONE',  ( 4.318543150850367773, 16.81600996003516357, -69.44999999999997442 ) ) ;
#36616=CARTESIAN_POINT ( 'NONE',  ( 1.028604700431328567, 23.06599248007198355, -55.20704692567388605 ) ) ;
#36617=CARTESIAN_POINT ( 'NONE',  ( 5.041649132594343996, 14.93115145952162415, -45.59999999999996589 ) ) ;
#36629=CARTESIAN_POINT ( 'NONE',  ( -4.314955953707389824, 21.59900333660018390, -39.74295307432605995 ) ) ;
#36631=CARTESIAN_POINT ( 'NONE',  ( -0.7798958854283041253, 23.40020640687986386, -46.05704692567387326 ) ) ;
#36635=CARTESIAN_POINT ( 'NONE',  ( 4.314955953707388936, 13.40099666339979123, -65.24295307432606705 ) ) ;
#36650=DIRECTION ( 'NONE',  ( 1.000000000000000000, 0.000000000000000000, 0.000000000000000000 ) ) ;
#36651=CARTESIAN_POINT ( 'NONE',  ( -5.301103610786608300, 14.79895279989743706, -31.64999999999995950 ) ) ;
#36655=CARTESIAN_POINT ( 'NONE',  ( -3.043106805520194413, 14.66227633819065623, -51.00704692567387610 ) ) ;
#36663=CARTESIAN_POINT ( 'NONE',  ( -3.895814058185739448, 15.51498359085620571, -52.64999999999997016 ) ) ;
#36665=CARTESIAN_POINT ( 'NONE',  ( -2.121074495332175847, 13.67351099933674341, -38.85704692567387752 ) ) ;
#36666=CARTESIAN_POINT ( 'NONE',  ( 0.9307174358028527106, 11.62368137996505801, -70.04999999999996874 ) ) ;
#36670=CARTESIAN_POINT ( 'NONE',  ( -3.826489000663265472, 15.37892550466785480, -39.14295307432606563 ) ) ;
#36675=CARTESIAN_POINT ( 'NONE',  ( 4.103766977300021601, 21.39838383358913987, -70.50704692567386189 ) ) ;
#36680=CARTESIAN_POINT ( 'NONE',  ( -5.876318620034919782, 18.43071743580290089, -34.94999999999996732 ) ) ;
#36697=CARTESIAN_POINT ( 'NONE',  ( 5.876318620034919782, 16.56928256419707068, -63.44999999999996732 ) ) ;
#36703=CARTESIAN_POINT ( 'NONE',  ( -3.705139346311794313, 19.38786279086902198, -38.09999999999996589 ) ) ;
#36704=CARTESIAN_POINT ( 'NONE',  ( -3.705139346311794313, 19.38786279086902198, -71.09999999999996589 ) ) ;
#36715=CARTESIAN_POINT ( 'NONE',  ( -1.848958322955462474, 13.53486088429179546, -44.84295307432606137 ) ) ;
#36719=CARTESIAN_POINT ( 'NONE',  ( 0.8348115903393232839, 13.20534463599456387, -68.54295307432605000 ) ) ;
#36739=CARTESIAN_POINT ( 'NONE',  ( -5.301103610786608300, 14.79895279989743706, -64.64999999999994884 ) ) ;
#36760=CARTESIAN_POINT ( 'NONE',  ( -4.314955953707389824, 21.59900333660018390, -51.74295307432605995 ) ) ;
#36768=CARTESIAN_POINT ( 'NONE',  ( 2.017261720333081598, 13.86079270138745834, -71.39295307432605853 ) ) ;
#36771=CARTESIAN_POINT ( 'NONE',  ( 0.5331684895902240040, 13.15756906230466328, -68.55704692567387326 ) ) ;
#36785=CARTESIAN_POINT ( 'NONE',  ( 0.7798958854283032371, 11.59979359312010772, -29.55704692567387681 ) ) ;
#36787=CARTESIAN_POINT ( 'NONE',  ( 0.6839900399647733664, 13.18145684914961357, -52.04999999999997584 ) ) ;
#36800=ORIENTED_EDGE ( 'NONE', *, *, #28003, .F. ) ;
#36801=CARTESIAN_POINT ( 'NONE',  ( -2.017261720333081598, 21.13920729861251857, -72.89295307432605853 ) ) ;
#36821=CARTESIAN_POINT ( 'NONE',  ( 1.887862790868997109, 13.79486065368817194, -42.89999999999996305 ) ) ;
#36830=CARTESIAN_POINT ( 'NONE',  ( -4.107178604518053611, 16.84948681541050775, -67.79999999999996874 ) ) ;
#36833=CARTESIAN_POINT ( 'NONE',  ( 5.611429750749524992, 18.24172506386835479, -52.80704692567387326 ) ) ;
#36834=CARTESIAN_POINT ( 'NONE',  ( 2.568848540478311460, 12.45835086740561692, -42.89999999999996305 ) ) ;
#36848=CARTESIAN_POINT ( 'NONE',  ( -5.852430833189966819, 18.58153898617744915, -33.45704692567387895 ) ) ;
#36852=CARTESIAN_POINT ( 'NONE',  ( 5.107581180293630396, 15.06055038898570686, -59.09295307432605426 ) ) ;
#36869=CARTESIAN_POINT ( 'NONE',  ( -5.588711115410763597, 16.61483511785016987, -34.79999999999996163 ) ) ;
#36872=CARTESIAN_POINT ( 'NONE',  ( 1.758463861404912620, 13.72892860598888731, -56.40704692567388179 ) ) ;
#36880=CARTESIAN_POINT ( 'NONE',  ( -3.091735541773221296, 20.59173554177323950, -56.24999999999995026 ) ) ;
#36882=CARTESIAN_POINT ( 'NONE',  ( 3.043106805520193525, 20.33772366180932067, -34.50704692567386900 ) ) ;
#36883=CARTESIAN_POINT ( 'NONE',  ( -2.701047200102606460, 12.19889638921340591, -73.34999999999996589 ) ) ;
#36894=CARTESIAN_POINT ( 'NONE',  ( -4.099003336600151925, 21.81495595370741469, -66.75704692567384768 ) ) ;
#36900=CARTESIAN_POINT ( 'NONE',  ( -5.041649132594344884, 20.06884854047834921, -38.09999999999996589 ) ) ;
#36915=CARTESIAN_POINT ( 'NONE',  ( -2.568848540478311904, 22.54164913259435465, -59.39999999999997016 ) ) ;
#36921=CARTESIAN_POINT ( 'NONE',  ( -2.940415233664778860, 14.55958476633523802, -37.49999999999996447 ) ) ;
#36922=CARTESIAN_POINT ( 'NONE',  ( 3.895814058185739892, 19.48501640914376054, -66.14999999999997726 ) ) ;
#36935=CARTESIAN_POINT ( 'NONE',  ( 0.5070733663080689846, 21.62989723985679902, -34.19295307432605568 ) ) ;
#36940=CARTESIAN_POINT ( 'NONE',  ( -3.771071394011080269, 19.25846386140493394, -57.59295307432605426 ) ) ;
#36960=CARTESIAN_POINT ( 'NONE',  ( -5.301103610786608300, 14.79895279989743706, -70.64999999999996305 ) ) ;
#36982=CARTESIAN_POINT ( 'NONE',  ( -0.7417250638684240727, 11.88857024925047057, -50.69295307432606279 ) ) ;
#36990=CARTESIAN_POINT ( 'NONE',  ( 4.084459969179292216, 18.29395300287091430, -70.79295307432605000 ) ) ;
#36992=CARTESIAN_POINT ( 'NONE',  ( -4.294655364005415699, 18.33481159033935626, -57.45704692567387895 ) ) ;
#37005=CARTESIAN_POINT ( 'NONE',  ( 0.6505131845895220088, 21.60717860451803674, -53.69999999999996732 ) ) ;
#37016=CARTESIAN_POINT ( 'NONE',  ( 4.342430937695320736, 16.96683151040971538, -73.94295307432606990 ) ) ;
#37034=CARTESIAN_POINT ( 'NONE',  ( -1.985016409143819605, 13.60418594181426855, -43.34999999999994458 ) ) ;
#37043=CARTESIAN_POINT ( 'NONE',  ( -4.318543150850367773, 18.18399003996480801, -64.94999999999996021 ) ) ;
#37045=CARTESIAN_POINT ( 'NONE',  ( -4.099003336600151925, 21.81495595370741469, -54.75704692567386900 ) ) ;
#37046=CARTESIAN_POINT ( 'NONE',  ( -5.041649132594344884, 20.06884854047834921, -47.09999999999996589 ) ) ;
#37055=PRODUCT_DEFINITION_FORMATION_WITH_SPECIFIED_SOURCE ( 'ANY', '', #4076, .NOT_KNOWN. ) ;
#37064=CARTESIAN_POINT ( 'NONE',  ( -5.370428668309080500, 14.93501088608579153, -39.15704692567386758 ) ) ;
#37067=CARTESIAN_POINT ( 'NONE',  ( -2.698247469942396837, 22.47571708489507358, -51.89295307432605853 ) ) ;
#37084=CARTESIAN_POINT ( 'NONE',  ( 2.701047200102605572, 22.80110361078655856, -29.84999999999996589 ) ) ;
#37087=CARTESIAN_POINT ( 'NONE',  ( -4.129897239856814117, 16.99292663369196177, -42.30704692567387326 ) ) ;
#37095=CARTESIAN_POINT ( 'NONE',  ( 1.887862790868997109, 13.79486065368817194, -48.89999999999997016 ) ) ;
#37098=CARTESIAN_POINT ( 'NONE',  ( 0.5331684895902240040, 13.15756906230466328, -38.55704692567387326 ) ) ;
#37111=CARTESIAN_POINT ( 'NONE',  ( 5.370428668309080500, 20.06498911391418360, -64.65704692567386758 ) ) ;
#37116=CARTESIAN_POINT ( 'NONE',  ( 4.001075405444606048, 21.50107540544455276, -26.99999999999996803 ) ) ;
#37131=CARTESIAN_POINT ( 'NONE',  ( -5.041649132594344884, 20.06884854047834921, -59.09999999999997300 ) ) ;
#37136=CARTESIAN_POINT ( 'NONE',  ( 3.705139346311793869, 15.61213720913094960, -27.59999999999996589 ) ) ;
#37137=CARTESIAN_POINT ( 'NONE',  ( 4.107178604518054499, 18.15051318458946383, -69.29999999999996874 ) ) ;
#37148=CARTESIAN_POINT ( 'NONE',  ( -0.8348115903393239501, 21.79465536400541126, -34.04295307432605711 ) ) ;
#37153=CARTESIAN_POINT ( 'NONE',  ( 3.199711850326839357, 14.51624076678035635, -56.24295307432605995 ) ) ;
#37167=CARTESIAN_POINT ( 'NONE',  ( -2.701047200102606016, 12.19889638921340413, -64.34999999999996589 ) ) ;
#37184=CARTESIAN_POINT ( 'NONE',  ( 2.698247469942395949, 12.52428291510489977, -53.39295307432605853 ) ) ;
#37193=CARTESIAN_POINT ( 'NONE',  ( -2.017261720333081598, 21.13920729861251857, -60.89295307432605853 ) ) ;
#37195=CARTESIAN_POINT ( 'NONE',  ( -3.639207298612509689, 19.51726172033310647, -54.60704692567387752 ) ) ;
#37207=CARTESIAN_POINT ( 'NONE',  ( -2.940415233664778860, 14.55958476633523802, -43.49999999999997158 ) ) ;
#37217=CARTESIAN_POINT ( 'NONE',  ( 2.837723661809363307, 20.54310680552015356, -76.49295307432603863 ) ) ;
#37230=CARTESIAN_POINT ( 'NONE',  ( -1.985016409143819605, 13.60418594181426855, -43.34999999999995879 ) ) ;
#37236=CARTESIAN_POINT ( 'NONE',  ( 1.887862790868997109, 13.79486065368817194, -33.89999999999996305 ) ) ;
#37245=CARTESIAN_POINT ( 'NONE',  ( -3.895814058185739448, 15.51498359085620571, -61.64999999999995595 ) ) ;
#37247=CARTESIAN_POINT ( 'NONE',  ( 4.103766977300021601, 21.39838383358913987, -43.50704692567387610 ) ) ;
#37248=CARTESIAN_POINT ( 'NONE',  ( 4.001075405444606048, 21.50107540544455276, -38.99999999999996447 ) ) ;
#37262=CARTESIAN_POINT ( 'NONE',  ( 5.370428668309080500, 20.06498911391418360, -37.65704692567386758 ) ) ;
#37267=CARTESIAN_POINT ( 'NONE',  ( -3.898383833589191827, 13.39623302270000771, -53.99295307432605995 ) ) ;
#37283=CARTESIAN_POINT ( 'NONE',  ( 4.314955953707388936, 13.40099666339979123, -74.24295307432606705 ) ) ;
#37286=CARTESIAN_POINT ( 'NONE',  ( 2.121074495332174958, 21.32648900066323350, -43.35704692567387752 ) ) ;
#37288=CARTESIAN_POINT ( 'NONE',  ( 1.887862790868997109, 13.79486065368817194, -60.89999999999997016 ) ) ;
#37298=CARTESIAN_POINT ( 'NONE',  ( 3.639207298612508801, 15.48273827966686866, -38.10704692567387752 ) ) ;
#37299=CARTESIAN_POINT ( 'NONE',  ( 5.588711115410763597, 18.38516488214980882, -69.29999999999996874 ) ) ;
#37312=CARTESIAN_POINT ( 'NONE',  ( -5.852430833189966819, 18.58153898617744915, -66.45704692567387895 ) ) ;
#37315=CARTESIAN_POINT ( 'NONE',  ( -0.8851648821498765418, 11.91128888458923285, -28.19999999999996732 ) ) ;
#37321=STYLED_ITEM('',(#42152),#24407);
#37332=CARTESIAN_POINT ( 'NONE',  ( 2.568848540478311460, 12.45835086740561692, -48.89999999999997016 ) ) ;
#37336=CARTESIAN_POINT ( 'NONE',  ( 3.965139115708213868, 19.34895832295540430, -70.65704692567386758 ) ) ;
#37337=CARTESIAN_POINT ( 'NONE',  ( 4.318543150850366885, 16.81600996003516713, -63.44999999999996732 ) ) ;
#37347=CARTESIAN_POINT ( 'NONE',  ( 1.848958322955461808, 21.46513911570817612, -34.34295307432605426 ) ) ;
#37350=CARTESIAN_POINT ( 'NONE',  ( -1.848958322955462474, 13.53486088429179546, -56.84295307432604716 ) ) ;
#37366=CARTESIAN_POINT ( 'NONE',  ( 4.206979645153767322, 13.29302035484617051, -60.74999999999995737 ) ) ;
#37386=CARTESIAN_POINT ( 'NONE',  ( 4.314955953707388936, 13.40099666339979123, -56.24295307432605995 ) ) ;
#37396=CARTESIAN_POINT ( 'NONE',  ( -3.826489000663265472, 15.37892550466785480, -69.14295307432605853 ) ) ;
#37398=CARTESIAN_POINT ( 'NONE',  ( 0.5331684895902240040, 13.15756906230466328, -53.55704692567387326 ) ) ;
#37410=CARTESIAN_POINT ( 'NONE',  ( -4.318543150850367773, 18.18399003996480801, -43.94999999999995310 ) ) ;
#37423=CARTESIAN_POINT ( 'NONE',  ( -4.084459969179292216, 16.70604699712905372, -72.29295307432605000 ) ) ;
#37437=CARTESIAN_POINT ( 'NONE',  ( 1.985016409143818272, 21.39581405818570659, -35.84999999999996589 ) ) ;
#37442=CARTESIAN_POINT ( 'NONE',  ( -4.318543150850367773, 18.18399003996480801, -37.94999999999996021 ) ) ;
#37451=CARTESIAN_POINT ( 'NONE',  ( 3.091735541773220852, 14.40826445822673563, -51.74999999999994316 ) ) ;
#37453=CARTESIAN_POINT ( 'NONE',  ( -1.028604700431329233, 11.93400751992799513, -47.70704692567387184 ) ) ;
#37454=CARTESIAN_POINT ( 'NONE',  ( 5.588711115410763597, 18.38516488214980882, -33.29999999999996874 ) ) ;
#37457=CARTESIAN_POINT ( 'NONE',  ( -0.6505131845895224529, 13.39282139548194195, -70.19999999999997442 ) ) ;
#37468=CARTESIAN_POINT ( 'NONE',  ( -1.028604700431329233, 11.93400751992799513, -32.70704692567387184 ) ) ;
#37471=CARTESIAN_POINT ( 'NONE',  ( 1.081538986177402295, 11.64756916681001186, -50.54295307432606421 ) ) ;
#37488=CARTESIAN_POINT ( 'NONE',  ( 4.001075405444606048, 21.50107540544455276, -26.99999999999996803 ) ) ;
#37491=CARTESIAN_POINT ( 'NONE',  ( 1.758463861404912620, 13.72892860598888731, -41.40704692567386758 ) ) ;
#37492=CARTESIAN_POINT ( 'NONE',  ( 0.6839900399647733664, 13.18145684914961357, -34.04999999999995453 ) ) ;
#37493=CARTESIAN_POINT ( 'NONE',  ( -0.6839900399647736995, 21.81854315085035623, -68.54999999999998295 ) ) ;
#37501=CARTESIAN_POINT ( 'NONE',  ( -3.639207298612509689, 19.51726172033310647, -30.60704692567387752 ) ) ;
#37502=CARTESIAN_POINT ( 'NONE',  ( -0.8851648821498765418, 11.91128888458923285, -61.19999999999996732 ) ) ;
#37514=CARTESIAN_POINT ( 'NONE',  ( -4.103766977300021601, 13.60161616641083704, -60.00704692567389031 ) ) ;
#37517=CARTESIAN_POINT ( 'NONE',  ( 5.876318620034919782, 16.56928256419707068, -33.44999999999994600 ) ) ;
#37534=CARTESIAN_POINT ( 'NONE',  ( -0.9307174358028533767, 23.37631862003491889, -47.54999999999997584 ) ) ;
#37538=CARTESIAN_POINT ( 'NONE',  ( 2.121074495332174958, 21.32648900066323350, -73.35704692567385621 ) ) ;
#37539=CARTESIAN_POINT ( 'NONE',  ( 3.091735541773220852, 14.40826445822673740, -54.74999999999996447 ) ) ;
#37546=CARTESIAN_POINT ( 'NONE',  ( 1.985016409143818272, 21.39581405818570303, -74.84999999999993747 ) ) ;
#37552=CARTESIAN_POINT ( 'NONE',  ( 0.8348115903393232839, 13.20534463599456387, -35.54295307432605711 ) ) ;
#37556=CARTESIAN_POINT ( 'NONE',  ( 3.199711850326839357, 14.51624076678035635, -50.24295307432605284 ) ) ;
#37571=CARTESIAN_POINT ( 'NONE',  ( -5.876318620034919782, 18.43071743580290089, -61.94999999999997442 ) ) ;
#37594=CARTESIAN_POINT ( 'NONE',  ( -5.565992480072003978, 16.47139529956871229, -45.29295307432605711 ) ) ;
#37602=CARTESIAN_POINT ( 'NONE',  ( -4.084459969179292216, 16.70604699712905372, -66.29295307432606421 ) ) ;
#37615=CARTESIAN_POINT ( 'NONE',  ( -3.705139346311794313, 19.38786279086902198, -50.09999999999996589 ) ) ;
#37642=CARTESIAN_POINT ( 'NONE',  ( -4.318543150850366885, 18.18399003996480801, -37.94999999999996021 ) ) ;
#37646=CARTESIAN_POINT ( 'NONE',  ( 4.107178604518054499, 18.15051318458946383, -39.29999999999996874 ) ) ;
#37654=CARTESIAN_POINT ( 'NONE',  ( 3.705139346311793869, 15.61213720913094960, -60.59999999999996589 ) ) ;
#37657=CARTESIAN_POINT ( 'NONE',  ( -2.837105286290963146, 12.26822144673588255, -50.85704692567387752 ) ) ;
#37658=CARTESIAN_POINT ( 'NONE',  ( 5.041649132594343996, 14.93115145952162415, -36.59999999999996589 ) ) ;
#37661=CARTESIAN_POINT ( 'NONE',  ( -4.342430937695320736, 18.03316848959025620, -27.44295307432605568 ) ) ;
#37672=CARTESIAN_POINT ( 'NONE',  ( 1.028604700431328567, 23.06599248007198355, -31.20704692567387539 ) ) ;
#37678=CARTESIAN_POINT ( 'NONE',  ( -3.898383833589191827, 13.39623302270000771, -47.99295307432606705 ) ) ;
#37697=CARTESIAN_POINT ( 'NONE',  ( 2.701047200102605572, 22.80110361078655856, -26.84999999999995524 ) ) ;
#37701=CARTESIAN_POINT ( 'NONE',  ( 2.121074495332174958, 21.32648900066323350, -40.35704692567387752 ) ) ;
#37702=CARTESIAN_POINT ( 'NONE',  ( -0.6839900399647736995, 21.81854315085035623, -32.54999999999996163 ) ) ;
#37703=CARTESIAN_POINT ( 'NONE',  ( -3.895814058185739448, 15.51498359085620571, -67.64999999999997726 ) ) ;
#37715=CARTESIAN_POINT ( 'NONE',  ( 2.983759233219601459, 14.30028814967311668, -29.25704692567387255 ) ) ;
#37716=CARTESIAN_POINT ( 'NONE',  ( 2.701047200102605128, 22.80110361078656211, -62.84999999999995879 ) ) ;
#37727=CARTESIAN_POINT ( 'NONE',  ( 0.7798958854283032371, 11.59979359312010772, -59.55704692567387326 ) ) ;
#37730=CARTESIAN_POINT ( 'NONE',  ( -4.314955953707389824, 21.59900333660018390, -75.74295307432603863 ) ) ;
#37746=CARTESIAN_POINT ( 'NONE',  ( -5.588711115410763597, 16.61483511785016987, -55.79999999999996874 ) ) ;
#37751=CARTESIAN_POINT ( 'NONE',  ( -3.043106805520194413, 14.66227633819065623, -72.00704692567386189 ) ) ;
#37752=CARTESIAN_POINT ( 'NONE',  ( -1.887862790868997553, 21.20513934631180319, -62.39999999999997016 ) ) ;
#37759=CARTESIAN_POINT ( 'NONE',  ( -1.887862790868997553, 21.20513934631180319, -71.39999999999996305 ) ) ;
#37763=CARTESIAN_POINT ( 'NONE',  ( 0.8348115903393232839, 13.20534463599456387, -38.54295307432605000 ) ) ;
#37766=CARTESIAN_POINT ( 'NONE',  ( 2.017261720333081598, 13.86079270138745834, -56.39295307432605853 ) ) ;
#37780=CARTESIAN_POINT ( 'NONE',  ( -5.588711115410763597, 16.61483511785016987, -58.79999999999996163 ) ) ;
#37801=CARTESIAN_POINT ( 'NONE',  ( 2.564989113914249330, 22.87042866830903876, -49.34295307432604716 ) ) ;
#37809=CARTESIAN_POINT ( 'NONE',  ( -3.826489000663265472, 15.37892550466785480, -63.14295307432606563 ) ) ;
#37822=CARTESIAN_POINT ( 'NONE',  ( 4.107178604518054499, 18.15051318458946383, -48.29999999999996874 ) ) ;
#37849=CARTESIAN_POINT ( 'NONE',  ( -1.985016409143819605, 13.60418594181426855, -31.34999999999996945 ) ) ;
#37853=CARTESIAN_POINT ( 'NONE',  ( -3.895814058185739448, 15.51498359085620571, -37.64999999999996305 ) ) ;
#37861=CARTESIAN_POINT ( 'NONE',  ( 1.887862790868997109, 13.79486065368817194, -57.89999999999996305 ) ) ;
#37863=CARTESIAN_POINT ( 'NONE',  ( 5.370428668309080500, 20.06498911391418360, -43.65704692567387468 ) ) ;
#37864=CARTESIAN_POINT ( 'NONE',  ( -2.568848540478311904, 22.54164913259435465, -38.39999999999997016 ) ) ;
#37866=CARTESIAN_POINT ( 'NONE',  ( -4.318543150850367773, 18.18399003996480801, -70.94999999999997442 ) ) ;
#37877=CARTESIAN_POINT ( 'NONE',  ( -4.975717084895059372, 20.19824746994243370, -24.60704692567387397 ) ) ;
#37882=CARTESIAN_POINT ( 'NONE',  ( 5.231778553264135212, 20.33710528629089254, -55.64295307432606563 ) ) ;
#37904=CARTESIAN_POINT ( 'NONE',  ( 0.7417250638684235176, 23.11142975074950101, -70.19295307432605568 ) ) ;
#37908=CARTESIAN_POINT ( 'NONE',  ( -0.6839900399647736995, 21.81854315085035623, -38.54999999999996874 ) ) ;
#37909=CARTESIAN_POINT ( 'NONE',  ( 0.6505131845895220088, 21.60717860451803674, -62.69999999999996732 ) ) ;
#37919=CARTESIAN_POINT ( 'NONE',  ( -1.028604700431329233, 11.93400751992799513, -71.70704692567387895 ) ) ;
#37920=CARTESIAN_POINT ( 'NONE',  ( 2.701047200102605128, 22.80110361078656211, -65.84999999999995168 ) ) ;
#37922=CARTESIAN_POINT ( 'NONE',  ( 3.470745319554692454, 20.97074531955464494, -74.99999999999997158 ) ) ;
#37932=CARTESIAN_POINT ( 'NONE',  ( -4.975717084895059372, 20.19824746994243370, -51.60704692567387752 ) ) ;
#37935=CARTESIAN_POINT ( 'NONE',  ( -4.206979645153768210, 21.70697964515380107, -26.24999999999996803 ) ) ;
#37954=CARTESIAN_POINT ( 'NONE',  ( -5.041649132594344884, 20.06884854047834921, -47.09999999999996589 ) ) ;
#37958=CARTESIAN_POINT ( 'NONE',  ( -3.965139115708213868, 15.65104167704456906, -72.15704692567386758 ) ) ;
#37959=CARTESIAN_POINT ( 'NONE',  ( -0.6505131845895224529, 13.39282139548194195, -58.19999999999996732 ) ) ;
#37965=CARTESIAN_POINT ( 'NONE',  ( 1.887862790868997109, 13.79486065368817194, -72.89999999999996305 ) ) ;
#37969=CARTESIAN_POINT ( 'NONE',  ( 4.107178604518054499, 18.15051318458946383, -72.29999999999996874 ) ) ;
#37972=CARTESIAN_POINT ( 'NONE',  ( 0.8348115903393232839, 13.20534463599456387, -47.54295307432606421 ) ) ;
#37986=CARTESIAN_POINT ( 'NONE',  ( -5.301103610786608300, 14.79895279989743706, -61.64999999999995595 ) ) ;
#37993=DIRECTION ( 'NONE',  ( 0.7071067811865507924, 0.7071067811865441310, 0.000000000000000000 ) ) ;
#38008=CARTESIAN_POINT ( 'NONE',  ( 1.081538986177402295, 11.64756916681001186, -44.54295307432605711 ) ) ;
#38015=CARTESIAN_POINT ( 'NONE',  ( -2.837723661809363751, 14.45689319447982335, -65.99295307432606705 ) ) ;
#38030=CARTESIAN_POINT ( 'NONE',  ( -1.887862790868997553, 21.20513934631180319, -50.39999999999996305 ) ) ;
#38056=CARTESIAN_POINT ( 'NONE',  ( 3.705139346311793869, 15.61213720913094960, -27.59999999999996589 ) ) ;
#38061=CARTESIAN_POINT ( 'NONE',  ( 2.940415233664778416, 20.44041523366473712, -35.99999999999996447 ) ) ;
#38071=CARTESIAN_POINT ( 'NONE',  ( -1.887862790868997553, 21.20513934631180319, -59.39999999999997016 ) ) ;
#38073=CARTESIAN_POINT ( 'NONE',  ( -5.370428668309080500, 14.93501088608579153, -51.15704692567387468 ) ) ;
#38074=CARTESIAN_POINT ( 'NONE',  ( 5.041649132594343996, 14.93115145952162415, -39.59999999999996589 ) ) ;
#38075=CARTESIAN_POINT ( 'NONE',  ( 1.887862790868997109, 13.79486065368817194, -72.89999999999996305 ) ) ;
#38088=CARTESIAN_POINT ( 'NONE',  ( -4.099003336600151925, 21.81495595370741469, -24.75704692567387610 ) ) ;
#38094=CARTESIAN_POINT ( 'NONE',  ( 2.698247469942395949, 12.52428291510489977, -41.39295307432605853 ) ) ;
#38112=CARTESIAN_POINT ( 'NONE',  ( -4.314955953707389824, 21.59900333660018390, -69.74295307432603863 ) ) ;
#38117=CARTESIAN_POINT ( 'NONE',  ( -3.091735541773221296, 20.59173554177323950, -32.24999999999996447 ) ) ;
#38118=CARTESIAN_POINT ( 'NONE',  ( -0.6839900399647736995, 21.81854315085035623, -65.54999999999996874 ) ) ;
#38128=CARTESIAN_POINT ( 'NONE',  ( -1.758463861404912842, 21.27107139401109137, -27.90704692567387823 ) ) ;
#38129=CARTESIAN_POINT ( 'NONE',  ( 4.206979645153768210, 13.29302035484617406, -63.74999999999997158 ) ) ;
#38139=CARTESIAN_POINT ( 'NONE',  ( 0.7798958854283032371, 11.59979359312010772, -53.55704692567387326 ) ) ;
#38145=CARTESIAN_POINT ( 'NONE',  ( -5.565992480072003978, 16.47139529956871229, -66.29295307432606421 ) ) ;
#38160=CARTESIAN_POINT ( 'NONE',  ( -5.301103610786608300, 14.79895279989743706, -49.64999999999995595 ) ) ;
#38163=CARTESIAN_POINT ( 'NONE',  ( -3.965139115708213868, 15.65104167704456906, -66.15704692567388179 ) ) ;
#38164=CARTESIAN_POINT ( 'NONE',  ( -3.091735541773221296, 20.59173554177323950, -56.24999999999995737 ) ) ;
#38172=CARTESIAN_POINT ( 'NONE',  ( -2.983759233219601903, 20.69971185032686023, -51.75704692567388321 ) ) ;
#38175=CARTESIAN_POINT ( 'NONE',  ( 3.771071394011080269, 15.74153613859503764, -29.09295307432605782 ) ) ;
#38178=CARTESIAN_POINT ( 'NONE',  ( -3.826489000663265472, 15.37892550466785480, -42.14295307432605142 ) ) ;
#38194=CARTESIAN_POINT ( 'NONE',  ( 4.001075405444606048, 21.50107540544455276, -50.99999999999997158 ) ) ;
#38218=CARTESIAN_POINT ( 'NONE',  ( 5.900206406879871857, 16.72010411457162604, -40.94295307432605568 ) ) ;
#38226=CARTESIAN_POINT ( 'NONE',  ( 1.848958322955461808, 21.46513911570817612, -58.34295307432606137 ) ) ;
#38242=CARTESIAN_POINT ( 'NONE',  ( 1.985016409143818272, 21.39581405818570303, -35.84999999999996589 ) ) ;
#38263=CARTESIAN_POINT ( 'NONE',  ( -2.940415233664778860, 14.55958476633523802, -31.49999999999996447 ) ) ;
#38267=CARTESIAN_POINT ( 'NONE',  ( -2.698247469942396837, 22.47571708489507358, -30.89295307432606208 ) ) ;
#38268=CARTESIAN_POINT ( 'NONE',  ( -4.107178604518053611, 16.84948681541050775, -28.79999999999996518 ) ) ;
#38276=CARTESIAN_POINT ( 'NONE',  ( 0.6839900399647733664, 13.18145684914961357, -58.04999999999996874 ) ) ;
#38279=CARTESIAN_POINT ( 'NONE',  ( -4.099003336600151925, 21.81495595370741469, -33.75704692567387610 ) ) ;
#38281=CARTESIAN_POINT ( 'NONE',  ( 4.318543150850367773, 16.81600996003516357, -72.44999999999994600 ) ) ;
#38291=CARTESIAN_POINT ( 'NONE',  ( -2.439449611014227859, 22.60758118029364283, -24.90704692567387823 ) ) ;
#38298=CARTESIAN_POINT ( 'NONE',  ( -5.231778553264134324, 14.66289471370907727, -39.14295307432606563 ) ) ;
#38315=CARTESIAN_POINT ( 'NONE',  ( 1.081538986177402295, 11.64756916681001186, -68.54295307432605000 ) ) ;
#38321=CARTESIAN_POINT ( 'NONE',  ( 4.107178604518054499, 18.15051318458946383, -39.29999999999996874 ) ) ;
#38322=CARTESIAN_POINT ( 'NONE',  ( 3.705139346311793869, 15.61213720913094960, -54.59999999999996589 ) ) ;
#38326=( BOUNDED_CURVE ( )  B_SPLINE_CURVE ( 2, ( #7150, #12904, #29684, #3526, #6523, #19491, #16520, #16930, #32460, #29469, #549, #26303, #13520, #10339, #3949, #41845, #12697, #25677, #27559, #33294, #27134, #23739, #7567, #17564, #1397, #11384, #36704, #4586, #17143, #20541, #10754, #40526, #20761, #27346, #11184, #33515, #30319, #39893, #37137, #4379, #17357, #7988, #40102, #24366, #20328, #4160, #8189, #14158, #24167, #1188, #10970, #33732, #23956, #26717, #39682, #17771, #36493, #26929, #33932, #36922, #4792, #30529, #14371, #4997, #21164, #7786, #40318, #30106, #29896, #20961, #982, #765, #30742, #1606, #13952, #14586, #10551, #37337, #34136, #13740, #23533, #7355, #18394, #11794, #37752, #5630, #31571, #41575, #24790, #34763, #5210, #8609, #40938, #15632, #8820, #15424, #41364, #21581, #31362, #18608, #21790, #12429, #15207, #41158, #34555, #28377, #34978, #2440, #5416, #22210, #14791, #25414, #37959, #2228, #40724, #12214, #34351, #31772, #28172, #18185, #12005, #31154, #24996, #25204, #17978, #38164, #2644, #1811, #38376, #9026, #2014, #22002, #9241, #28588, #18812, #37539, #5841, #35179, #14996, #30954, #27755, #11581, #24574, #8394, #21373, #27961, #31991, #35607, #22631, #41790, #25623, #284, #38582, #9668, #16061, #3068, #2856, #13464, #38795, #19637, #32610, #76, #19438, #16260, #9883, #29001, #15846, #28790, #36010, #12641, #41999, #10075, #6470, #23042, #12847, #29630, #9448, #6876, #32408, #25831, #22415, #6045, #3473, #35392, #19022, #26250, #3272, #19232, #13267, #6257, #13055, #32204, #26450, #39406, #26039, #495, #29199, #39001, #22838, #29414, #35806, #6669, #16464, #39198, #19847, #32815, #3685, #16672, #10281, #23252, #40419, #37230, #11475, #40617, #11682, #26661, #27647, #34447, #5100, #17668, #13681, #30635, #41043, #33031, #2115, #14689, #11277, #16878, #34240, #10493, #8497, #1499, #36441, #8085, #24260, #14478, #5308, #31253, #21475, #21062, #1707, #15100, #30846, #7304, #27451, #28061, #18281, #37642, #39622, #24680, #31051, #23478, #36217, #17871, #34038, #33830, #709, #11896, #4893, #7091, #24467, #37437, #29842, #20856, #1903, #4688, #8292, #21269, #18079, #3897, #20069, #14885, #27853, #40830, #25517, #34863, #32094, #41466, #15520, #41678, #21680, #19335, #15317, #28273, #3176, #9128, #6149, #6360, #29104, #25300, #38263, #37849, #8705, #12317, #22107, #18492, #2330, #19129, #41254, #28477, #5734, #31669, #22517, #2962, #35287, #12100, #15952, #18912, #32307, #42103, #35078, #18710, #28901, #5938, #16164, #25092, #38056, #24886, #31878, #41897, #2748, #28686, #2537, #34653, #5520, #12746, #31461, #21887, #25726, #15731, #38689 ),
 .UNSPECIFIED., .F., .T. ) 
 B_SPLINE_CURVE_WITH_KNOTS ( ( 3, 2, 2, 2, 2, 2, 2, 2, 2, 2, 2, 2, 2, 2, 2, 2, 2, 2, 2, 2, 2, 2, 2, 2, 2, 2, 2, 2, 2, 2, 2, 2, 2, 2, 2, 2, 2, 2, 2, 2, 2, 2, 2, 2, 2, 2, 2, 2, 2, 2, 2, 2, 2, 2, 2, 2, 2, 2, 2, 2, 2, 2, 2, 2, 2, 2, 2, 2, 2, 2, 2, 2, 2, 2, 2, 2, 2, 2, 2, 2, 2, 2, 2, 2, 2, 2, 2, 2, 2, 2, 2, 2, 2, 2, 2, 2, 2, 2, 2, 2, 2, 2, 2, 2, 2, 2, 2, 2, 2, 2, 2, 2, 2, 2, 2, 2, 2, 2, 2, 2, 2, 2, 2, 2, 2, 2, 2, 2, 2, 2, 2, 2, 2, 2, 2, 2, 2, 2, 2, 2, 2, 2, 2, 2, 2, 2, 2, 2, 2, 2, 2, 2, 2, 2, 2, 2, 2, 2, 2, 2, 2, 2, 2, 2, 2, 3 ),
 ( 0.000000000000000000, 0.005882352941176470507, 0.01176470588235294101, 0.01764705882352941152, 0.02352941176470588203, 0.02941176470588235253, 0.03529411764705882304, 0.04117647058823529355, 0.04705882352941176405, 0.05294117647058823456, 0.05882352941176470507, 0.06470588235294118251, 0.07058823529411764608, 0.07647058823529412352, 0.08235294117647058709, 0.08823529411764706454, 0.09411764705882352811, 0.1000000000000000056, 0.1058823529411764691, 0.1117647058823529466, 0.1176470588235294101, 0.1235294117647058876, 0.1294117647058823650, 0.1352941176470588147, 0.1411764705882352922, 0.1470588235294117696, 0.1529411764705882470, 0.1588235294117646967, 0.1647058823529411742, 0.1705882352941176516, 0.1764705882352941291, 0.1823529411764705788, 0.1882352941176470562, 0.1941176470588235337, 0.2000000000000000111, 0.2058823529411764608, 0.2117647058823529382, 0.2176470588235294157, 0.2235294117647058931, 0.2294117647058823428, 0.2352941176470588203, 0.2411764705882352977, 0.2470588235294117752, 0.2529411764705882248, 0.2588235294117647300, 0.2647058823529411797, 0.2705882352941176294, 0.2764705882352941346, 0.2823529411764705843, 0.2882352941176470340, 0.2941176470588235392, 0.2999999999999999889, 0.3058823529411764941, 0.3117647058823528883, 0.3176470588235293935, 0.3235294117647058987, 0.3294117647058823484, 0.3352941176470587981, 0.3411764705882353033, 0.3470588235294117530, 0.3529411764705882582, 0.3588235294117647078, 0.3647058823529411575, 0.3705882352941176627, 0.3764705882352941124, 0.3823529411764705621, 0.3882352941176470673, 0.3941176470588235170, 0.4000000000000000222, 0.4058823529411764719, 0.4117647058823529216, 0.4176470588235294268, 0.4235294117647058765, 0.4294117647058823262, 0.4352941176470588314, 0.4411764705882352811, 0.4470588235294117863, 0.4529411764705882359, 0.4588235294117646856, 0.4647058823529411908, 0.4705882352941176405, 0.4764705882352940902, 0.4823529411764705954, 0.4882352941176470451, 0.4941176470588235503, 0.5000000000000000000, 0.5058823529411764497, 0.5117647058823528994, 0.5176470588235294601, 0.5235294117647059098, 0.5294117647058823595, 0.5352941176470588092, 0.5411764705882352589, 0.5470588235294118196, 0.5529411764705882693, 0.5588235294117647189, 0.5647058823529411686, 0.5705882352941176183, 0.5764705882352940680, 0.5823529411764706287, 0.5882352941176470784, 0.5941176470588235281, 0.5999999999999999778, 0.6058823529411764275, 0.6117647058823529882, 0.6176470588235294379, 0.6235294117647057766, 0.6294117647058823373, 0.6352941176470587870, 0.6411764705882353477, 0.6470588235294117974, 0.6529411764705882470, 0.6588235294117646967, 0.6647058823529411464, 0.6705882352941175961, 0.6764705882352941568, 0.6823529411764706065, 0.6882352941176470562, 0.6941176470588235059, 0.6999999999999999556, 0.7058823529411765163, 0.7117647058823529660, 0.7176470588235294157, 0.7235294117647058654, 0.7294117647058823151, 0.7352941176470588758, 0.7411764705882353255, 0.7470588235294116641, 0.7529411764705882248, 0.7588235294117646745, 0.7647058823529411242, 0.7705882352941176849, 0.7764705882352941346, 0.7823529411764705843, 0.7882352941176470340, 0.7941176470588234837, 0.8000000000000000444, 0.8058823529411764941, 0.8117647058823529438, 0.8176470588235293935, 0.8235294117647058432, 0.8294117647058824039, 0.8352941176470588536, 0.8411764705882353033, 0.8470588235294117530, 0.8529411764705882026, 0.8588235294117646523, 0.8647058823529412130, 0.8705882352941176627, 0.8764705882352941124, 0.8823529411764705621, 0.8882352941176470118, 0.8941176470588235725, 0.9000000000000000222, 0.9058823529411764719, 0.9117647058823529216, 0.9176470588235293713, 0.9235294117647059320, 0.9294117647058823817, 0.9352941176470588314, 0.9411764705882352811, 0.9470588235294117307, 0.9529411764705881804, 0.9588235294117647411, 0.9647058823529411908, 0.9705882352941176405 ),
 .UNSPECIFIED. ) 
 CURVE ( )  GEOMETRIC_REPRESENTATION_ITEM ( )  RATIONAL_B_SPLINE_CURVE ( ( 1.000000000000000000, 0.9510565162951535312, 1.000000000000000000, 0.9510565162951535312, 1.000000000000000000, 0.9510565162951535312, 1.000000000000000000, 0.9510565162951535312, 1.000000000000000000, 0.9510565162951535312, 1.000000000000000000, 0.9510565162951535312, 1.000000000000000000, 0.9510565162951535312, 1.000000000000000000, 0.9510565162951535312, 1.000000000000000000, 0.9510565162951535312, 1.000000000000000000, 0.9510565162951535312, 1.000000000000000000, 0.9510565162951535312, 1.000000000000000000, 0.9510565162951535312, 1.000000000000000000, 0.9510565162951535312, 1.000000000000000000, 0.9510565162951535312, 1.000000000000000000, 0.9510565162951535312, 1.000000000000000000, 0.9510565162951535312, 1.000000000000000000, 0.9510565162951535312, 1.000000000000000000, 0.9510565162951535312, 1.000000000000000000, 0.9510565162951535312, 1.000000000000000000, 0.9510565162951535312, 1.000000000000000000, 0.9510565162951535312, 1.000000000000000000, 0.9510565162951535312, 1.000000000000000000, 0.9510565162951535312, 1.000000000000000000, 0.9510565162951535312, 1.000000000000000000, 0.9510565162951535312, 1.000000000000000000, 0.9510565162951535312, 1.000000000000000000, 0.9510565162951535312, 1.000000000000000000, 0.9510565162951535312, 1.000000000000000000, 0.9510565162951535312, 1.000000000000000000, 0.9510565162951535312, 1.000000000000000000, 0.9510565162951535312, 1.000000000000000000, 0.9510565162951535312, 1.000000000000000000, 0.9510565162951535312, 1.000000000000000000, 0.9510565162951535312, 1.000000000000000000, 0.9510565162951535312, 1.000000000000000000, 0.9510565162951535312, 1.000000000000000000, 0.9510565162951535312, 1.000000000000000000, 0.9510565162951535312, 1.000000000000000000, 0.9510565162951535312, 1.000000000000000000, 0.9510565162951535312, 1.000000000000000000, 0.9510565162951535312, 1.000000000000000000, 0.9510565162951535312, 1.000000000000000000, 0.9510565162951535312, 1.000000000000000000, 0.9510565162951535312, 1.000000000000000000, 0.9510565162951535312, 1.000000000000000000, 0.9510565162951535312, 1.000000000000000000, 0.9510565162951535312, 1.000000000000000000, 0.9510565162951535312, 1.000000000000000000, 0.9510565162951535312, 1.000000000000000000, 0.9510565162951535312, 1.000000000000000000, 0.9510565162951535312, 1.000000000000000000, 0.9510565162951535312, 1.000000000000000000, 0.9510565162951535312, 1.000000000000000000, 0.9510565162951535312, 1.000000000000000000, 0.9510565162951535312, 1.000000000000000000, 0.9510565162951535312, 1.000000000000000000, 0.9510565162951535312, 1.000000000000000000, 0.9510565162951535312, 1.000000000000000000, 0.9510565162951535312, 1.000000000000000000, 0.9510565162951535312, 1.000000000000000000, 0.9510565162951535312, 1.000000000000000000, 0.9510565162951535312, 1.000000000000000000, 0.9510565162951535312, 1.000000000000000000, 0.9510565162951535312, 1.000000000000000000, 0.9510565162951535312, 1.000000000000000000, 0.9510565162951535312, 1.000000000000000000, 0.9510565162951535312, 1.000000000000000000, 0.9510565162951535312, 1.000000000000000000, 0.9510565162951535312, 1.000000000000000000, 0.9510565162951535312, 1.000000000000000000, 0.9510565162951535312, 1.000000000000000000, 0.9510565162951535312, 1.000000000000000000, 0.9510565162951535312, 1.000000000000000000, 0.9510565162951535312, 1.000000000000000000, 0.9510565162951535312, 1.000000000000000000, 0.9510565162951535312, 1.000000000000000000, 0.9510565162951535312, 1.000000000000000000, 0.9510565162951535312, 1.000000000000000000, 0.9510565162951535312, 1.000000000000000000, 0.9510565162951535312, 1.000000000000000000, 0.9510565162951535312, 1.000000000000000000, 0.9510565162951535312, 1.000000000000000000, 0.9510565162951535312, 1.000000000000000000, 0.9510565162951535312, 1.000000000000000000, 0.9510565162951535312, 1.000000000000000000, 0.9510565162951535312, 1.000000000000000000, 0.9510565162951535312, 1.000000000000000000, 0.9510565162951535312, 1.000000000000000000, 0.9510565162951535312, 1.000000000000000000, 0.9510565162951535312, 1.000000000000000000, 0.9510565162951535312, 1.000000000000000000, 0.9510565162951535312, 1.000000000000000000, 0.9510565162951535312, 1.000000000000000000, 0.9510565162951535312, 1.000000000000000000, 0.9510565162951535312, 1.000000000000000000, 0.9510565162951535312, 1.000000000000000000, 0.9510565162951535312, 1.000000000000000000, 0.9510565162951535312, 1.000000000000000000, 0.9510565162951535312, 1.000000000000000000, 0.9510565162951535312, 1.000000000000000000, 0.9510565162951535312, 1.000000000000000000, 0.9510565162951535312, 1.000000000000000000, 0.9510565162951535312, 1.000000000000000000, 0.9510565162951535312, 1.000000000000000000, 0.9510565162951535312, 1.000000000000000000, 0.9510565162951535312, 1.000000000000000000, 0.9510565162951535312, 1.000000000000000000, 0.9510565162951535312, 1.000000000000000000, 0.9510565162951535312, 1.000000000000000000, 0.9510565162951535312, 1.000000000000000000, 0.9510565162951535312, 1.000000000000000000, 0.9510565162951535312, 1.000000000000000000, 0.9510565162951535312, 1.000000000000000000, 0.9510565162951535312, 1.000000000000000000, 0.9510565162951535312, 1.000000000000000000, 0.9510565162951535312, 1.000000000000000000, 0.9510565162951535312, 1.000000000000000000, 0.9510565162951535312, 1.000000000000000000, 0.9510565162951535312, 1.000000000000000000, 0.9510565162951535312, 1.000000000000000000, 0.9510565162951535312, 1.000000000000000000, 0.9510565162951535312, 1.000000000000000000, 0.9510565162951535312, 1.000000000000000000, 0.9510565162951535312, 1.000000000000000000, 0.9510565162951535312, 1.000000000000000000, 0.9510565162951535312, 1.000000000000000000, 0.9510565162951535312, 1.000000000000000000, 0.9510565162951535312, 1.000000000000000000, 0.9510565162951535312, 1.000000000000000000, 0.9510565162951535312, 1.000000000000000000, 0.9510565162951535312, 1.000000000000000000, 0.9510565162951535312, 1.000000000000000000, 0.9510565162951535312, 1.000000000000000000, 0.9510565162951535312, 1.000000000000000000, 0.9510565162951535312, 1.000000000000000000, 0.9510565162951535312, 1.000000000000000000, 0.9510565162951535312, 1.000000000000000000, 0.9510565162951535312, 1.000000000000000000, 0.9510565162951535312, 1.000000000000000000, 0.9510565162951535312, 1.000000000000000000, 0.9510565162951535312, 1.000000000000000000, 0.9510565162951535312, 1.000000000000000000, 0.9510565162951535312, 1.000000000000000000, 0.9510565162951535312, 1.000000000000000000, 0.9510565162951535312, 1.000000000000000000, 0.9510565162951535312, 1.000000000000000000, 0.9510565162951535312, 1.000000000000000000, 0.9510565162951535312, 1.000000000000000000, 0.9510565162951535312, 1.000000000000000000, 0.9510565162951535312, 1.000000000000000000, 0.9510565162951535312, 1.000000000000000000, 0.9510565162951535312, 1.000000000000000000, 0.9510565162951535312, 1.000000000000000000, 0.9510565162951535312, 1.000000000000000000, 0.9510565162951535312, 1.000000000000000000, 0.9510565162951535312, 1.000000000000000000, 0.9510565162951535312, 1.000000000000000000, 0.9510565162951535312, 1.000000000000000000, 0.9510565162951535312, 1.000000000000000000, 0.9510565162951535312, 1.000000000000000000, 0.9510565162951535312, 1.000000000000000000, 0.9510565162951535312, 1.000000000000000000, 0.9510565162951535312, 1.000000000000000000, 0.9510565162951535312, 1.000000000000000000, 0.9510565162951535312, 1.000000000000000000 ) ) 
 REPRESENTATION_ITEM ( '' )  );
#38336=CARTESIAN_POINT ( 'NONE',  ( 3.043106805520193525, 20.33772366180932067, -25.50704692567387610 ) ) ;
#38337=CARTESIAN_POINT ( 'NONE',  ( 5.588711115410763597, 18.38516488214980882, -51.29999999999996874 ) ) ;
#38349=CARTESIAN_POINT ( 'NONE',  ( 5.852430833189966819, 16.41846101382252243, -55.95704692567386473 ) ) ;
#38354=CARTESIAN_POINT ( 'NONE',  ( -3.898383833589191827, 13.39623302270000771, -74.99295307432603863 ) ) ;
#38371=CARTESIAN_POINT ( 'NONE',  ( -2.701047200102606016, 12.19889638921340413, -37.34999999999994458 ) ) ;
#38375=CARTESIAN_POINT ( 'NONE',  ( 4.294655364005415699, 16.66518840966061887, -61.95704692567387895 ) ) ;
#38376=CARTESIAN_POINT ( 'NONE',  ( -4.107178604518053611, 16.84948681541050775, -55.79999999999996874 ) ) ;
#38386=CARTESIAN_POINT ( 'NONE',  ( 4.107178604518054499, 18.15051318458946383, -66.29999999999996874 ) ) ;
#38388=CARTESIAN_POINT ( 'NONE',  ( -0.5331684895902242260, 21.84243093769531185, -55.05704692567387326 ) ) ;
#38391=CARTESIAN_POINT ( 'NONE',  ( -0.8348115903393239501, 21.79465536400541126, -28.04295307432605355 ) ) ;
#38394=CARTESIAN_POINT ( 'NONE',  ( -0.5070733663080690956, 13.37010276014318144, -41.69295307432606279 ) ) ;
#38408=CARTESIAN_POINT ( 'NONE',  ( -4.206979645153768210, 21.70697964515380107, -50.24999999999997158 ) ) ;
#38425=CARTESIAN_POINT ( 'NONE',  ( -0.8851648821498765418, 11.91128888458923285, -67.19999999999997442 ) ) ;
#38431=CARTESIAN_POINT ( 'NONE',  ( 0.6505131845895220088, 21.60717860451803674, -47.69999999999996732 ) ) ;
#38432=CARTESIAN_POINT ( 'NONE',  ( -4.314955953707389824, 21.59900333660018390, -42.74295307432605284 ) ) ;
#38442=CARTESIAN_POINT ( 'NONE',  ( -2.837723661809363751, 14.45689319447982335, -56.99295307432605995 ) ) ;
#38456=CARTESIAN_POINT ( 'NONE',  ( -3.895814058185739448, 15.51498359085620571, -40.64999999999994174 ) ) ;
#38482=CARTESIAN_POINT ( 'NONE',  ( -3.043106805520194413, 14.66227633819065623, -39.00704692567386900 ) ) ;
#38486=CARTESIAN_POINT ( 'NONE',  ( 5.107581180293630396, 15.06055038898570686, -32.09295307432605426 ) ) ;
#38487=CARTESIAN_POINT ( 'NONE',  ( -3.895814058185739448, 15.51498359085620571, -28.64999999999995950 ) ) ;
#38494=CARTESIAN_POINT ( 'NONE',  ( -2.940415233664778860, 14.55958476633523802, -49.49999999999996447 ) ) ;
#38497=CARTESIAN_POINT ( 'NONE',  ( 2.439449611014226971, 12.39241881970633230, -41.40704692567386758 ) ) ;
#38499=CARTESIAN_POINT ( 'NONE',  ( -1.985016409143819605, 13.60418594181426855, -64.34999999999996589 ) ) ;
#38508=CARTESIAN_POINT ( 'NONE',  ( 5.370428668309080500, 20.06498911391418360, -25.65704692567387823 ) ) ;
#38512=CARTESIAN_POINT ( 'NONE',  ( -2.698247469942396837, 22.47571708489507358, -42.89295307432605853 ) ) ;
#38529=CARTESIAN_POINT ( 'NONE',  ( 2.564989113914249330, 22.87042866830903876, -61.34295307432606137 ) ) ;
#38534=CARTESIAN_POINT ( 'NONE',  ( 3.091735541773220852, 14.40826445822673563, -27.74999999999995381 ) ) ;
#38535=CARTESIAN_POINT ( 'NONE',  ( -3.895814058185739448, 15.51498359085620571, -58.64999999999997016 ) ) ;
#38545=CARTESIAN_POINT ( 'NONE',  ( 1.028604700431328567, 23.06599248007198355, -70.20704692567387895 ) ) ;
#38546=CARTESIAN_POINT ( 'NONE',  ( 2.701047200102605128, 22.80110361078656211, -59.84999999999996589 ) ) ;
#38557=CARTESIAN_POINT ( 'NONE',  ( -2.439449611014227859, 22.60758118029364283, -57.90704692567388179 ) ) ;
#38560=CARTESIAN_POINT ( 'NONE',  ( 0.7417250638684235176, 23.11142975074950101, -70.19295307432605568 ) ) ;
#38577=CARTESIAN_POINT ( 'NONE',  ( -5.588711115410763597, 16.61483511785016987, -40.79999999999996874 ) ) ;
#38581=CARTESIAN_POINT ( 'NONE',  ( -0.7939530028709754772, 13.41554003082070246, -65.70704692567387895 ) ) ;
#38582=CARTESIAN_POINT ( 'NONE',  ( -0.6505131845895224529, 13.39282139548194195, -52.19999999999996732 ) ) ;
#38593=CARTESIAN_POINT ( 'NONE',  ( -1.985016409143819605, 13.60418594181426855, -64.34999999999996589 ) ) ;
#38595=CARTESIAN_POINT ( 'NONE',  ( -4.129897239856814117, 16.99292663369196177, -45.30704692567388037 ) ) ;
#38598=CARTESIAN_POINT ( 'NONE',  ( 3.199711850326839357, 14.51624076678035635, -29.24295307432605640 ) ) ;
#38601=CARTESIAN_POINT ( 'NONE',  ( 3.199711850326839357, 14.51624076678035635, -47.24295307432605995 ) ) ;
#38615=CARTESIAN_POINT ( 'NONE',  ( -2.568848540478311904, 22.54164913259435465, -47.39999999999997016 ) ) ;
#38631=CARTESIAN_POINT ( 'NONE',  ( 5.876318620034919782, 16.56928256419707068, -66.44999999999997442 ) ) ;
#38636=CARTESIAN_POINT ( 'NONE',  ( 1.985016409143818272, 21.39581405818570303, -44.84999999999996589 ) ) ;
#38647=CARTESIAN_POINT ( 'NONE',  ( 4.084459969179292216, 18.29395300287091430, -52.79295307432607132 ) ) ;
#38664=CARTESIAN_POINT ( 'NONE',  ( 1.887862790868997109, 13.79486065368817194, -33.89999999999996305 ) ) ;
#38688=CARTESIAN_POINT ( 'NONE',  ( 2.983759233219601459, 14.30028814967311668, -38.25704692567386900 ) ) ;
#38689=CARTESIAN_POINT ( 'NONE',  ( -2.940415233664778860, 14.55958476633523802, -25.49999999999996803 ) ) ;
#38692=CARTESIAN_POINT ( 'NONE',  ( -2.564989113914250662, 12.12957133169093282, -29.84295307432605782 ) ) ;
#38694=CARTESIAN_POINT ( 'NONE',  ( -2.940415233664778860, 14.55958476633523802, -28.49999999999996447 ) ) ;
#38703=CARTESIAN_POINT ( 'NONE',  ( 1.985016409143818272, 21.39581405818570303, -50.84999999999997300 ) ) ;
#38706=CARTESIAN_POINT ( 'NONE',  ( -4.099003336600151925, 21.81495595370741469, -36.75704692567386900 ) ) ;
#38708=CARTESIAN_POINT ( 'NONE',  ( 2.940415233664778416, 20.44041523366473712, -65.99999999999997158 ) ) ;
#38724=CARTESIAN_POINT ( 'NONE',  ( 5.107581180293630396, 15.06055038898570686, -38.09295307432605426 ) ) ;
#38737=CARTESIAN_POINT ( 'NONE',  ( 5.231778553264135212, 20.33710528629089254, -64.64295307432604432 ) ) ;
#38744=CARTESIAN_POINT ( 'NONE',  ( 1.985016409143818272, 21.39581405818570303, -53.84999999999995879 ) ) ;
#38753=EDGE_LOOP ( 'NONE', ( #18695, #27734 ) ) ;
#38756=CARTESIAN_POINT ( 'NONE',  ( -5.611429750749524992, 16.75827493613162034, -69.30704692567387326 ) ) ;
#38757=CARTESIAN_POINT ( 'NONE',  ( 0.9307174358028527106, 11.62368137996505801, -58.04999999999996163 ) ) ;
#38770=CARTESIAN_POINT ( 'NONE',  ( -2.837105286290963146, 12.26822144673588255, -50.85704692567387752 ) ) ;
#38774=CARTESIAN_POINT ( 'NONE',  ( 5.565992480072003978, 18.52860470043125574, -70.79295307432605000 ) ) ;
#38790=CARTESIAN_POINT ( 'NONE',  ( -0.9307174358028533767, 23.37631862003491889, -44.54999999999994742 ) ) ;
#38794=CARTESIAN_POINT ( 'NONE',  ( -3.639207298612509689, 19.51726172033310647, -60.60704692567387752 ) ) ;
#38795=CARTESIAN_POINT ( 'NONE',  ( 4.107178604518054499, 18.15051318458946383, -51.29999999999996874 ) ) ;
#38804=CARTESIAN_POINT ( 'NONE',  ( 3.705139346311793869, 15.61213720913094960, -66.59999999999996589 ) ) ;
#38806=CARTESIAN_POINT ( 'NONE',  ( -3.965139115708213868, 15.65104167704456906, -42.15704692567387468 ) ) ;
#38824=CARTESIAN_POINT ( 'NONE',  ( -4.206979645153768210, 21.70697964515380107, -47.24999999999995026 ) ) ;
#38839=CARTESIAN_POINT ( 'NONE',  ( -0.8851648821498765418, 11.91128888458923285, -70.19999999999997442 ) ) ;
#38844=CARTESIAN_POINT ( 'NONE',  ( -4.107178604518053611, 16.84948681541050775, -43.79999999999996163 ) ) ;
#38857=CARTESIAN_POINT ( 'NONE',  ( -3.199711850326840246, 20.48375923321962233, -57.74295307432607416 ) ) ;
#38874=CARTESIAN_POINT ( 'NONE',  ( -4.107178604518053611, 16.84948681541050775, -31.79999999999996874 ) ) ;
#38899=CARTESIAN_POINT ( 'NONE',  ( -0.5331684895902242260, 21.84243093769531185, -34.05704692567386616 ) ) ;
#38904=CARTESIAN_POINT ( 'NONE',  ( -0.7417250638684240727, 11.88857024925047057, -35.69295307432606279 ) ) ;
#38905=CARTESIAN_POINT ( 'NONE',  ( -4.318543150850367773, 18.18399003996480801, -28.94999999999996021 ) ) ;
#38913=CARTESIAN_POINT ( 'NONE',  ( 0.6839900399647733664, 13.18145684914961357, -43.04999999999996163 ) ) ;
#38917=CARTESIAN_POINT ( 'NONE',  ( -2.439449611014227859, 22.60758118029364283, -36.90704692567386758 ) ) ;
#38919=CARTESIAN_POINT ( 'NONE',  ( -1.887862790868997553, 21.20513934631180319, -68.39999999999997726 ) ) ;
#38932=CARTESIAN_POINT ( 'NONE',  ( 3.898383833589191383, 21.60376697729997275, -28.49295307432605995 ) ) ;
#38945=AXIS2_PLACEMENT_3D ( 'NONE', #8896, #2938, #19101 ) ;
#38954=CARTESIAN_POINT ( 'NONE',  ( 1.985016409143818272, 21.39581405818570303, -26.84999999999995524 ) ) ;
#38955=CARTESIAN_POINT ( 'NONE',  ( -3.705139346311794313, 19.38786279086902198, -50.09999999999996589 ) ) ;
#38964=CARTESIAN_POINT ( 'NONE',  ( -0.7798958854283041253, 23.40020640687986386, -67.05704692567387326 ) ) ;
#38965=CARTESIAN_POINT ( 'NONE',  ( -5.301103610786608300, 14.79895279989743528, -55.64999999999995595 ) ) ;
#38978=CARTESIAN_POINT ( 'NONE',  ( -4.975717084895059372, 20.19824746994243370, -45.60704692567387752 ) ) ;
#38982=CARTESIAN_POINT ( 'NONE',  ( -5.565992480072003978, 16.47139529956871229, -69.29295307432606421 ) ) ;
#38996=CARTESIAN_POINT ( 'NONE',  ( 5.301103610786608300, 20.20104720010253985, -42.14999999999996305 ) ) ;
#39000=CARTESIAN_POINT ( 'NONE',  ( -0.5331684895902242260, 21.84243093769531185, -61.05704692567386616 ) ) ;
#39001=CARTESIAN_POINT ( 'NONE',  ( 4.318543150850366885, 16.81600996003516713, -45.44999999999996021 ) ) ;
#39010=CARTESIAN_POINT ( 'NONE',  ( -3.705139346311794313, 19.38786279086902198, -62.09999999999996589 ) ) ;
#39012=CARTESIAN_POINT ( 'NONE',  ( -4.294655364005415699, 18.33481159033935626, -45.45704692567387184 ) ) ;
#39015=CARTESIAN_POINT ( 'NONE',  ( 1.848958322955461808, 21.46513911570817612, -34.34295307432605426 ) ) ;
#39027=CARTESIAN_POINT ( 'NONE',  ( -5.588711115410763597, 16.61483511785016987, -46.79999999999996874 ) ) ;
#39044=CARTESIAN_POINT ( 'NONE',  ( -2.568848540478311904, 22.54164913259435465, -71.39999999999996305 ) ) ;
#39049=CARTESIAN_POINT ( 'NONE',  ( 3.091735541773220852, 14.40826445822673563, -39.74999999999996447 ) ) ;
#39061=CARTESIAN_POINT ( 'NONE',  ( -2.837723661809363751, 14.45689319447982335, -50.99295307432605995 ) ) ;
#39078=CARTESIAN_POINT ( 'NONE',  ( -0.6505131845895224529, 13.39282139548194195, -34.19999999999996732 ) ) ;
#39099=CARTESIAN_POINT ( 'NONE',  ( -2.121074495332175847, 13.67351099933674341, -29.85704692567387397 ) ) ;
#39103=CARTESIAN_POINT ( 'NONE',  ( -5.231778553264134324, 14.66289471370907727, -39.14295307432606563 ) ) ;
#39105=CARTESIAN_POINT ( 'NONE',  ( -0.5331684895902242260, 21.84243093769531185, -70.05704692567387326 ) ) ;
#39113=CARTESIAN_POINT ( 'NONE',  ( -4.318543150850367773, 18.18399003996480801, -49.94999999999994600 ) ) ;
#39116=CARTESIAN_POINT ( 'NONE',  ( 4.099003336600150149, 13.18504404629255689, -38.25704692567386900 ) ) ;
#39117=CARTESIAN_POINT ( 'NONE',  ( -5.041649132594344884, 20.06884854047834921, -29.09999999999996589 ) ) ;
#39118=CARTESIAN_POINT ( 'NONE',  ( -3.895814058185739448, 15.51498359085620571, -64.64999999999994884 ) ) ;
#39129=CARTESIAN_POINT ( 'NONE',  ( 1.081538986177402295, 11.64756916681001186, -29.54295307432605355 ) ) ;
#39148=CARTESIAN_POINT ( 'NONE',  ( 2.940415233664778416, 20.44041523366473712, -26.99999999999996803 ) ) ;
#39149=CARTESIAN_POINT ( 'NONE',  ( 0.6839900399647733664, 13.18145684914961357, -52.04999999999997584 ) ) ;
#39158=CARTESIAN_POINT ( 'NONE',  ( -4.103766977300021601, 13.60161616641083704, -69.00704692567386189 ) ) ;
#39159=CARTESIAN_POINT ( 'NONE',  ( 4.001075405444606048, 21.50107540544455276, -59.99999999999997158 ) ) ;
#39174=CARTESIAN_POINT ( 'NONE',  ( -5.852430833189966819, 18.58153898617744915, -48.45704692567387895 ) ) ;
#39178=CARTESIAN_POINT ( 'NONE',  ( -5.231778553264134324, 14.66289471370907727, -60.14295307432605142 ) ) ;
#39194=CARTESIAN_POINT ( 'NONE',  ( 5.876318620034919782, 16.56928256419707068, -45.44999999999996021 ) ) ;
#39197=CARTESIAN_POINT ( 'NONE',  ( 4.129897239856814117, 18.00707336630801336, -52.80704692567387326 ) ) ;
#39198=CARTESIAN_POINT ( 'NONE',  ( -0.6839900399647738105, 21.81854315085035623, -44.54999999999995453 ) ) ;
#39207=CARTESIAN_POINT ( 'NONE',  ( 0.6505131845895220088, 21.60717860451803674, -59.69999999999996732 ) ) ;
#39209=CARTESIAN_POINT ( 'NONE',  ( -0.5331684895902242260, 21.84243093769531185, -49.05704692567388037 ) ) ;
#39213=CARTESIAN_POINT ( 'NONE',  ( 3.199711850326839357, 14.51624076678035635, -35.24295307432605995 ) ) ;
#39219=CARTESIAN_POINT ( 'NONE',  ( 0.7939530028709752552, 21.58445996917927445, -28.20704692567387184 ) ) ;
#39226=CARTESIAN_POINT ( 'NONE',  ( 5.041649132594343996, 14.93115145952162415, -36.59999999999996589 ) ) ;
#39242=CARTESIAN_POINT ( 'NONE',  ( -2.568848540478311904, 22.54164913259435465, -74.39999999999996305 ) ) ;
#39247=CARTESIAN_POINT ( 'NONE',  ( 1.985016409143818272, 21.39581405818570303, -38.84999999999996589 ) ) ;
#39259=CARTESIAN_POINT ( 'NONE',  ( -1.848958322955462474, 13.53486088429179546, -41.84295307432606137 ) ) ;
#39264=CARTESIAN_POINT ( 'NONE',  ( -4.342430937695320736, 18.03316848959025620, -63.44295307432605568 ) ) ;
#39275=CARTESIAN_POINT ( 'NONE',  ( 3.705139346311793869, 15.61213720913094960, -30.59999999999996589 ) ) ;
#39282=CARTESIAN_POINT ( 'NONE',  ( 5.611429750749524992, 18.24172506386835479, -25.80704692567386971 ) ) ;
#39303=CARTESIAN_POINT ( 'NONE',  ( -0.7939530028709754772, 13.41554003082070246, -32.70704692567387184 ) ) ;
#39307=CARTESIAN_POINT ( 'NONE',  ( -5.107581180293630396, 19.93944961101426827, -27.59295307432605782 ) ) ;
#39308=CARTESIAN_POINT ( 'NONE',  ( 3.043106805520193525, 20.33772366180932067, -61.50704692567389031 ) ) ;
#39315=CARTESIAN_POINT ( 'NONE',  ( 0.6839900399647733664, 13.18145684914961357, -46.04999999999996163 ) ) ;
#39318=CARTESIAN_POINT ( 'NONE',  ( -0.7798958854283041253, 23.40020640687986386, -31.05704692567387681 ) ) ;
#39321=CARTESIAN_POINT ( 'NONE',  ( 4.318543150850367773, 16.81600996003516357, -69.44999999999997442 ) ) ;
#39332=CARTESIAN_POINT ( 'NONE',  ( -2.564989113914250662, 12.12957133169093282, -29.84295307432605782 ) ) ;
#39350=CARTESIAN_POINT ( 'NONE',  ( -3.705139346311794313, 19.38786279086902198, -26.09999999999996234 ) ) ;
#39351=CARTESIAN_POINT ( 'NONE',  ( -3.705139346311794313, 19.38786279086902198, -41.09999999999996589 ) ) ;
#39362=CARTESIAN_POINT ( 'NONE',  ( 3.826489000663266360, 19.62107449533211678, -28.64295307432606208 ) ) ;
#39364=CARTESIAN_POINT ( 'NONE',  ( 2.837105286290961370, 22.73177855326409613, -67.35704692567388463 ) ) ;
#39365=CARTESIAN_POINT ( 'NONE',  ( 5.588711115410763597, 18.38516488214980882, -42.29999999999996874 ) ) ;
#39382=CARTESIAN_POINT ( 'NONE',  ( 2.837105286290961370, 22.73177855326409613, -40.35704692567387752 ) ) ;
#39386=CARTESIAN_POINT ( 'NONE',  ( -5.565992480072003978, 16.47139529956871229, -63.29295307432605000 ) ) ;
#39401=CARTESIAN_POINT ( 'NONE',  ( 0.9307174358028528216, 11.62368137996505801, -28.04999999999995453 ) ) ;
#39405=CARTESIAN_POINT ( 'NONE',  ( -4.294655364005415699, 18.33481159033935626, -54.45704692567387895 ) ) ;
#39406=CARTESIAN_POINT ( 'NONE',  ( 0.6839900399647732554, 13.18145684914961357, -46.04999999999996163 ) ) ;
#39415=CARTESIAN_POINT ( 'NONE',  ( -0.6505131845895224529, 13.39282139548194195, -58.19999999999996732 ) ) ;
#39417=CARTESIAN_POINT ( 'NONE',  ( 3.639207298612508801, 15.48273827966686866, -44.10704692567387752 ) ) ;
#39423=CARTESIAN_POINT ( 'NONE',  ( 3.826489000663266360, 19.62107449533211678, -34.64295307432605142 ) ) ;
#39430=CARTESIAN_POINT ( 'NONE',  ( -4.099003336600151925, 21.81495595370741469, -72.75704692567386189 ) ) ;
#39439=CARTESIAN_POINT ( 'NONE',  ( 2.568848540478311460, 12.45835086740561692, -36.89999999999997016 ) ) ;
#39458=CARTESIAN_POINT ( 'NONE',  ( 4.206979645153767322, 13.29302035484617051, -57.74999999999995737 ) ) ;
#39464=CARTESIAN_POINT ( 'NONE',  ( -1.985016409143819605, 13.60418594181426855, -37.34999999999994458 ) ) ;
#39477=CARTESIAN_POINT ( 'NONE',  ( -2.017261720333081598, 21.13920729861251857, -45.89295307432605853 ) ) ;
#39482=CARTESIAN_POINT ( 'NONE',  ( -4.084459969179292216, 16.70604699712905372, -66.29295307432606421 ) ) ;
#39501=CARTESIAN_POINT ( 'NONE',  ( -4.001075405444606936, 13.49892459455542060, -67.49999999999995737 ) ) ;
#39515=CARTESIAN_POINT ( 'NONE',  ( -5.107581180293630396, 19.93944961101426827, -60.59295307432606847 ) ) ;
#39519=CARTESIAN_POINT ( 'NONE',  ( 0.5331684895902240040, 13.15756906230466328, -35.55704692567386616 ) ) ;
#39525=CARTESIAN_POINT ( 'NONE',  ( -4.342430937695320736, 18.03316848959025620, -75.44295307432606990 ) ) ;
#39526=CARTESIAN_POINT ( 'NONE',  ( 2.121074495332174958, 21.32648900066323350, -64.35704692567387042 ) ) ;
#39535=CARTESIAN_POINT ( 'NONE',  ( 1.887862790868997109, 13.79486065368817194, -39.89999999999996305 ) ) ;
#39536=CARTESIAN_POINT ( 'NONE',  ( -5.611429750749524992, 16.75827493613162034, -30.30704692567387326 ) ) ;
#39538=CARTESIAN_POINT ( 'NONE',  ( -1.887862790868997553, 21.20513934631180319, -59.39999999999997016 ) ) ;
#39551=CARTESIAN_POINT ( 'NONE',  ( -1.081538986177402961, 23.35243083318996327, -31.04295307432605355 ) ) ;
#39573=CARTESIAN_POINT ( 'NONE',  ( 1.985016409143818272, 21.39581405818570303, -41.84999999999995879 ) ) ;
#39581=CARTESIAN_POINT ( 'NONE',  ( 0.6505131845895220088, 21.60717860451803674, -65.69999999999996021 ) ) ;
#39583=CARTESIAN_POINT ( 'NONE',  ( -5.370428668309080500, 14.93501088608579153, -60.15704692567387468 ) ) ;
#39584=CARTESIAN_POINT ( 'NONE',  ( 0.9307174358028527106, 11.62368137996505801, -46.04999999999996163 ) ) ;
#39597=CARTESIAN_POINT ( 'NONE',  ( 5.370428668309080500, 20.06498911391418360, -40.65704692567387468 ) ) ;
#39601=CARTESIAN_POINT ( 'NONE',  ( 5.900206406879871857, 16.72010411457162604, -64.94295307432605568 ) ) ;
#39618=CARTESIAN_POINT ( 'NONE',  ( -2.568848540478311904, 22.54164913259435465, -35.39999999999996305 ) ) ;
#39621=CARTESIAN_POINT ( 'NONE',  ( -2.121074495332175847, 13.67351099933674341, -56.85704692567387042 ) ) ;
#39622=CARTESIAN_POINT ( 'NONE',  ( -4.107178604518053611, 16.84948681541050775, -37.79999999999996874 ) ) ;
#39623=CARTESIAN_POINT ( 'NONE',  ( -1.985016409143819605, 13.60418594181426855, -73.34999999999996589 ) ) ;
#39632=CARTESIAN_POINT ( 'NONE',  ( 0.6839900399647733664, 13.18145684914961357, -52.04999999999997584 ) ) ;
#39634=CARTESIAN_POINT ( 'NONE',  ( 3.965139115708213868, 19.34895832295540430, -31.65704692567386402 ) ) ;
#39639=CARTESIAN_POINT ( 'NONE',  ( 3.826489000663266360, 19.62107449533211678, -31.64295307432605853 ) ) ;
#39648=CARTESIAN_POINT ( 'NONE',  ( -4.129897239856814117, 16.99292663369196177, -27.30704692567386971 ) ) ;
#39654=CARTESIAN_POINT ( 'NONE',  ( 4.001075405444606048, 21.50107540544455276, -35.99999999999996447 ) ) ;
#39676=CARTESIAN_POINT ( 'NONE',  ( 2.701047200102605572, 22.80110361078655856, -65.84999999999992326 ) ) ;
#39681=CARTESIAN_POINT ( 'NONE',  ( 0.6839900399647733664, 13.18145684914961357, -34.04999999999995453 ) ) ;
#39682=CARTESIAN_POINT ( 'NONE',  ( 1.887862790868997109, 13.79486065368817194, -66.89999999999997726 ) ) ;
#39692=CARTESIAN_POINT ( 'NONE',  ( -4.342430937695320736, 18.03316848959025620, -42.44295307432605568 ) ) ;
#39697=CARTESIAN_POINT ( 'NONE',  ( -3.826489000663265472, 15.37892550466785480, -66.14295307432605853 ) ) ;
#39720=CARTESIAN_POINT ( 'NONE',  ( 5.301103610786608300, 20.20104720010253985, -66.14999999999997726 ) ) ;
#39737=CARTESIAN_POINT ( 'NONE',  ( -5.107581180293630396, 19.93944961101426827, -51.59295307432605426 ) ) ;
#39748=CARTESIAN_POINT ( 'NONE',  ( -1.848958322955462474, 13.53486088429179546, -74.84295307432606137 ) ) ;
#39749=CARTESIAN_POINT ( 'NONE',  ( 2.983759233219601459, 14.30028814967311668, -65.25704692567387610 ) ) ;
#39760=CARTESIAN_POINT ( 'NONE',  ( 1.028604700431328567, 23.06599248007198355, -25.20704692567387539 ) ) ;
#39762=CARTESIAN_POINT ( 'NONE',  ( -3.091735541773221296, 20.59173554177323950, -59.24999999999997158 ) ) ;
#39776=CARTESIAN_POINT ( 'NONE',  ( -1.081538986177402961, 23.35243083318996327, -34.04295307432605711 ) ) ;
#39796=CARTESIAN_POINT ( 'NONE',  ( 0.6505131845895220088, 21.60717860451803674, -47.69999999999996732 ) ) ;
#39806=CARTESIAN_POINT ( 'NONE',  ( 3.705139346311793869, 15.61213720913094960, -66.59999999999996589 ) ) ;
#39808=CARTESIAN_POINT ( 'NONE',  ( -4.103766977300021601, 13.60161616641083704, -60.00704692567389031 ) ) ;
#39809=CARTESIAN_POINT ( 'NONE',  ( -2.701047200102606460, 12.19889638921340591, -49.34999999999996589 ) ) ;
#39821=CARTESIAN_POINT ( 'NONE',  ( 5.852430833189966819, 16.41846101382252243, -43.95704692567387184 ) ) ;
#39825=( BOUNDED_CURVE ( )  B_SPLINE_CURVE ( 2, ( #30490, #7955, #14333, #17731, #941, #40278, #20080, #23491, #7531, #4118, #33044, #36883, #27312, #20502, #10715, #7745, #1571, #13907, #11147, #13693, #26674, #10509, #20719, #16891, #7317, #23264, #4546, #3909, #20921, #14549, #39855, #23703, #27521, #36666, #33472, #24749, #11968, #14759, #37299, #31534, #31327, #5805, #2186, #11343, #2402, #5176, #24330, #27715, #40688, #31737, #15168, #41119, #41325, #8779, #4959, #24961, #17940, #15592, #8154, #12174, #5593, #37920, #15390, #40898, #18148, #28133, #30918, #34312, #8358, #25165, #1776, #11544, #24536, #21752, #21129, #38129, #21339, #2606, #18353, #8571, #34724, #37716, #31119, #34100, #5375, #28341, #21546, #11753, #18564, #18777, #1972, #8987, #37502, #14958, #27924, #21960, #34934, #40489, #34516, #244, #39159, #38546, #9628, #13226, #9842, #19193, #22377, #19596, #31950, #22801, #35356, #26212, #41, #38757, #35772, #16428, #16021, #6633, #32569, #6429, #19400, #10040, #32372, #26001, #3436, #32165, #28963, #6219, #23003, #38965, #29375, #41538, #25585, #22590, #41959, #2820, #25791, #3028, #28752, #15804, #12604, #35972, #6836, #19809, #41748, #32778, #12807, #35566, #3236, #3644, #16219, #29163, #28550, #13021, #25377, #12392, #9413, #6007, #38337, #9199, #22175, #35145, #18984, #33422, #3862, #13858, #36179, #17481, #4067, #33646, #4500, #39809, #4286, #17268, #30231, #29803, #1311, #24080, #30442, #32995, #20667, #26838, #26624, #14285, #7270, #7906, #37046, #40014, #7050, #27264, #456, #20874, #10673, #39584, #10243, #40226, #36617, #1106, #14078, #16841, #23655, #20455, #29592, #7694, #23438, #13427, #668, #13641, #33845, #27051, #10884, #11096, #23869, #23212, #36834, #20030, #16633, #26412, #39365, #10459, #36403, #20242, #17052, #33203, #30015, #888, #7481, #14706, #31480, #11293, #24277, #17890, #34463, #27468, #2347, #27664, #38074, #24696, #14900, #18296, #37248, #40635, #30654, #11698, #37864, #27869, #5118, #5323, #12116, #8309, #34669, #8102, #21080, #4910, #8722, #8515, #37658, #34053, #18511, #15334, #18098, #31269, #11493, #40434, #28078, #1519, #30863, #31068, #2132, #1725, #14497, #21694, #21491, #25110, #21904, #28288, #24485, #15116, #37454, #21289, #34258, #1920, #41272, #40845, #41059, #11911, #24905, #8932, #5537, #4705, #17685, #3192, #26165, #22122, #16179, #35094, #6378, #41913, #5955, #12761, #2977, #12334, #9996, #18727, #6589, #29560, #39117, #32324, #19144, #34883, #12548, #19555, #18929, #6167, #31896, #19350, #29328, #41694, #25534, #12973, #32527, #15749, #5750, #25742, #15967, #29118, #41486, #25319, #9146, #3395, #9577 ),
 .UNSPECIFIED., .F., .F. ) 
 B_SPLINE_CURVE_WITH_KNOTS ( ( 3, 2, 2, 2, 2, 2, 2, 2, 2, 2, 2, 2, 2, 2, 2, 2, 2, 2, 2, 2, 2, 2, 2, 2, 2, 2, 2, 2, 2, 2, 2, 2, 2, 2, 2, 2, 2, 2, 2, 2, 2, 2, 2, 2, 2, 2, 2, 2, 2, 2, 2, 2, 2, 2, 2, 2, 2, 2, 2, 2, 2, 2, 2, 2, 2, 2, 2, 2, 2, 2, 2, 2, 2, 2, 2, 2, 2, 2, 2, 2, 2, 2, 2, 2, 2, 2, 2, 2, 2, 2, 2, 2, 2, 2, 2, 2, 2, 2, 2, 2, 2, 2, 2, 2, 2, 2, 2, 2, 2, 2, 2, 2, 2, 2, 2, 2, 2, 2, 2, 2, 2, 2, 2, 2, 2, 2, 2, 2, 2, 2, 2, 2, 2, 2, 2, 2, 2, 2, 2, 2, 2, 2, 2, 2, 2, 2, 2, 2, 2, 2, 2, 2, 2, 2, 2, 2, 2, 2, 2, 2, 2, 2, 2, 2, 2, 3 ),
 ( 0.000000000000000000, 0.005882352941176470507, 0.01176470588235294101, 0.01764705882352941152, 0.02352941176470588203, 0.02941176470588235253, 0.03529411764705882304, 0.04117647058823529355, 0.04705882352941176405, 0.05294117647058823456, 0.05882352941176470507, 0.06470588235294118251, 0.07058823529411764608, 0.07647058823529412352, 0.08235294117647058709, 0.08823529411764706454, 0.09411764705882352811, 0.1000000000000000056, 0.1058823529411764691, 0.1117647058823529466, 0.1176470588235294101, 0.1235294117647058876, 0.1294117647058823650, 0.1352941176470588147, 0.1411764705882352922, 0.1470588235294117696, 0.1529411764705882470, 0.1588235294117646967, 0.1647058823529411742, 0.1705882352941176516, 0.1764705882352941291, 0.1823529411764705788, 0.1882352941176470562, 0.1941176470588235337, 0.2000000000000000111, 0.2058823529411764608, 0.2117647058823529382, 0.2176470588235294157, 0.2235294117647058931, 0.2294117647058823428, 0.2352941176470588203, 0.2411764705882352977, 0.2470588235294117752, 0.2529411764705882248, 0.2588235294117647300, 0.2647058823529411797, 0.2705882352941176294, 0.2764705882352941346, 0.2823529411764705843, 0.2882352941176470340, 0.2941176470588235392, 0.2999999999999999889, 0.3058823529411764941, 0.3117647058823528883, 0.3176470588235293935, 0.3235294117647058987, 0.3294117647058823484, 0.3352941176470587981, 0.3411764705882353033, 0.3470588235294117530, 0.3529411764705882582, 0.3588235294117647078, 0.3647058823529411575, 0.3705882352941176627, 0.3764705882352941124, 0.3823529411764705621, 0.3882352941176470673, 0.3941176470588235170, 0.4000000000000000222, 0.4058823529411764719, 0.4117647058823529216, 0.4176470588235294268, 0.4235294117647058765, 0.4294117647058823262, 0.4352941176470588314, 0.4411764705882352811, 0.4470588235294117863, 0.4529411764705882359, 0.4588235294117646856, 0.4647058823529411908, 0.4705882352941176405, 0.4764705882352940902, 0.4823529411764705954, 0.4882352941176470451, 0.4941176470588235503, 0.5000000000000000000, 0.5058823529411764497, 0.5117647058823528994, 0.5176470588235294601, 0.5235294117647059098, 0.5294117647058823595, 0.5352941176470588092, 0.5411764705882352589, 0.5470588235294118196, 0.5529411764705882693, 0.5588235294117647189, 0.5647058823529411686, 0.5705882352941176183, 0.5764705882352940680, 0.5823529411764706287, 0.5882352941176470784, 0.5941176470588235281, 0.5999999999999999778, 0.6058823529411764275, 0.6117647058823529882, 0.6176470588235294379, 0.6235294117647057766, 0.6294117647058823373, 0.6352941176470587870, 0.6411764705882353477, 0.6470588235294117974, 0.6529411764705882470, 0.6588235294117646967, 0.6647058823529411464, 0.6705882352941175961, 0.6764705882352941568, 0.6823529411764706065, 0.6882352941176470562, 0.6941176470588235059, 0.6999999999999999556, 0.7058823529411765163, 0.7117647058823529660, 0.7176470588235294157, 0.7235294117647058654, 0.7294117647058823151, 0.7352941176470588758, 0.7411764705882353255, 0.7470588235294116641, 0.7529411764705882248, 0.7588235294117646745, 0.7647058823529411242, 0.7705882352941176849, 0.7764705882352941346, 0.7823529411764705843, 0.7882352941176470340, 0.7941176470588234837, 0.8000000000000000444, 0.8058823529411764941, 0.8117647058823529438, 0.8176470588235293935, 0.8235294117647058432, 0.8294117647058824039, 0.8352941176470588536, 0.8411764705882353033, 0.8470588235294117530, 0.8529411764705882026, 0.8588235294117646523, 0.8647058823529412130, 0.8705882352941176627, 0.8764705882352941124, 0.8823529411764705621, 0.8882352941176470118, 0.8941176470588235725, 0.9000000000000000222, 0.9058823529411764719, 0.9117647058823529216, 0.9176470588235293713, 0.9235294117647059320, 0.9294117647058823817, 0.9352941176470588314, 0.9411764705882352811, 0.9470588235294117307, 0.9529411764705881804, 0.9588235294117647411, 0.9647058823529411908, 0.9705882352941176405 ),
 .UNSPECIFIED. ) 
 CURVE ( )  GEOMETRIC_REPRESENTATION_ITEM ( )  RATIONAL_B_SPLINE_CURVE ( ( 1.000000000000000000, 0.9510565162951535312, 1.000000000000000000, 0.9510565162951535312, 1.000000000000000000, 0.9510565162951535312, 1.000000000000000000, 0.9510565162951535312, 1.000000000000000000, 0.9510565162951535312, 1.000000000000000000, 0.9510565162951535312, 1.000000000000000000, 0.9510565162951535312, 1.000000000000000000, 0.9510565162951535312, 1.000000000000000000, 0.9510565162951535312, 1.000000000000000000, 0.9510565162951535312, 1.000000000000000000, 0.9510565162951535312, 1.000000000000000000, 0.9510565162951535312, 1.000000000000000000, 0.9510565162951535312, 1.000000000000000000, 0.9510565162951535312, 1.000000000000000000, 0.9510565162951535312, 1.000000000000000000, 0.9510565162951535312, 1.000000000000000000, 0.9510565162951535312, 1.000000000000000000, 0.9510565162951535312, 1.000000000000000000, 0.9510565162951535312, 1.000000000000000000, 0.9510565162951535312, 1.000000000000000000, 0.9510565162951535312, 1.000000000000000000, 0.9510565162951535312, 1.000000000000000000, 0.9510565162951535312, 1.000000000000000000, 0.9510565162951535312, 1.000000000000000000, 0.9510565162951535312, 1.000000000000000000, 0.9510565162951535312, 1.000000000000000000, 0.9510565162951535312, 1.000000000000000000, 0.9510565162951535312, 1.000000000000000000, 0.9510565162951535312, 1.000000000000000000, 0.9510565162951535312, 1.000000000000000000, 0.9510565162951535312, 1.000000000000000000, 0.9510565162951535312, 1.000000000000000000, 0.9510565162951535312, 1.000000000000000000, 0.9510565162951535312, 1.000000000000000000, 0.9510565162951535312, 1.000000000000000000, 0.9510565162951535312, 1.000000000000000000, 0.9510565162951535312, 1.000000000000000000, 0.9510565162951535312, 1.000000000000000000, 0.9510565162951535312, 1.000000000000000000, 0.9510565162951535312, 1.000000000000000000, 0.9510565162951535312, 1.000000000000000000, 0.9510565162951535312, 1.000000000000000000, 0.9510565162951535312, 1.000000000000000000, 0.9510565162951535312, 1.000000000000000000, 0.9510565162951535312, 1.000000000000000000, 0.9510565162951535312, 1.000000000000000000, 0.9510565162951535312, 1.000000000000000000, 0.9510565162951535312, 1.000000000000000000, 0.9510565162951535312, 1.000000000000000000, 0.9510565162951535312, 1.000000000000000000, 0.9510565162951535312, 1.000000000000000000, 0.9510565162951535312, 1.000000000000000000, 0.9510565162951535312, 1.000000000000000000, 0.9510565162951535312, 1.000000000000000000, 0.9510565162951535312, 1.000000000000000000, 0.9510565162951535312, 1.000000000000000000, 0.9510565162951535312, 1.000000000000000000, 0.9510565162951535312, 1.000000000000000000, 0.9510565162951535312, 1.000000000000000000, 0.9510565162951535312, 1.000000000000000000, 0.9510565162951535312, 1.000000000000000000, 0.9510565162951535312, 1.000000000000000000, 0.9510565162951535312, 1.000000000000000000, 0.9510565162951535312, 1.000000000000000000, 0.9510565162951535312, 1.000000000000000000, 0.9510565162951535312, 1.000000000000000000, 0.9510565162951535312, 1.000000000000000000, 0.9510565162951535312, 1.000000000000000000, 0.9510565162951535312, 1.000000000000000000, 0.9510565162951535312, 1.000000000000000000, 0.9510565162951535312, 1.000000000000000000, 0.9510565162951535312, 1.000000000000000000, 0.9510565162951535312, 1.000000000000000000, 0.9510565162951535312, 1.000000000000000000, 0.9510565162951535312, 1.000000000000000000, 0.9510565162951535312, 1.000000000000000000, 0.9510565162951535312, 1.000000000000000000, 0.9510565162951535312, 1.000000000000000000, 0.9510565162951535312, 1.000000000000000000, 0.9510565162951535312, 1.000000000000000000, 0.9510565162951535312, 1.000000000000000000, 0.9510565162951535312, 1.000000000000000000, 0.9510565162951535312, 1.000000000000000000, 0.9510565162951535312, 1.000000000000000000, 0.9510565162951535312, 1.000000000000000000, 0.9510565162951535312, 1.000000000000000000, 0.9510565162951535312, 1.000000000000000000, 0.9510565162951535312, 1.000000000000000000, 0.9510565162951535312, 1.000000000000000000, 0.9510565162951535312, 1.000000000000000000, 0.9510565162951535312, 1.000000000000000000, 0.9510565162951535312, 1.000000000000000000, 0.9510565162951535312, 1.000000000000000000, 0.9510565162951535312, 1.000000000000000000, 0.9510565162951535312, 1.000000000000000000, 0.9510565162951535312, 1.000000000000000000, 0.9510565162951535312, 1.000000000000000000, 0.9510565162951535312, 1.000000000000000000, 0.9510565162951535312, 1.000000000000000000, 0.9510565162951535312, 1.000000000000000000, 0.9510565162951535312, 1.000000000000000000, 0.9510565162951535312, 1.000000000000000000, 0.9510565162951535312, 1.000000000000000000, 0.9510565162951535312, 1.000000000000000000, 0.9510565162951535312, 1.000000000000000000, 0.9510565162951535312, 1.000000000000000000, 0.9510565162951535312, 1.000000000000000000, 0.9510565162951535312, 1.000000000000000000, 0.9510565162951535312, 1.000000000000000000, 0.9510565162951535312, 1.000000000000000000, 0.9510565162951535312, 1.000000000000000000, 0.9510565162951535312, 1.000000000000000000, 0.9510565162951535312, 1.000000000000000000, 0.9510565162951535312, 1.000000000000000000, 0.9510565162951535312, 1.000000000000000000, 0.9510565162951535312, 1.000000000000000000, 0.9510565162951535312, 1.000000000000000000, 0.9510565162951535312, 1.000000000000000000, 0.9510565162951535312, 1.000000000000000000, 0.9510565162951535312, 1.000000000000000000, 0.9510565162951535312, 1.000000000000000000, 0.9510565162951535312, 1.000000000000000000, 0.9510565162951535312, 1.000000000000000000, 0.9510565162951535312, 1.000000000000000000, 0.9510565162951535312, 1.000000000000000000, 0.9510565162951535312, 1.000000000000000000, 0.9510565162951535312, 1.000000000000000000, 0.9510565162951535312, 1.000000000000000000, 0.9510565162951535312, 1.000000000000000000, 0.9510565162951535312, 1.000000000000000000, 0.9510565162951535312, 1.000000000000000000, 0.9510565162951535312, 1.000000000000000000, 0.9510565162951535312, 1.000000000000000000, 0.9510565162951535312, 1.000000000000000000, 0.9510565162951535312, 1.000000000000000000, 0.9510565162951535312, 1.000000000000000000, 0.9510565162951535312, 1.000000000000000000, 0.9510565162951535312, 1.000000000000000000, 0.9510565162951535312, 1.000000000000000000, 0.9510565162951535312, 1.000000000000000000, 0.9510565162951535312, 1.000000000000000000, 0.9510565162951535312, 1.000000000000000000, 0.9510565162951535312, 1.000000000000000000, 0.9510565162951535312, 1.000000000000000000, 0.9510565162951535312, 1.000000000000000000, 0.9510565162951535312, 1.000000000000000000, 0.9510565162951535312, 1.000000000000000000, 0.9510565162951535312, 1.000000000000000000, 0.9510565162951535312, 1.000000000000000000, 0.9510565162951535312, 1.000000000000000000, 0.9510565162951535312, 1.000000000000000000, 0.9510565162951535312, 1.000000000000000000, 0.9510565162951535312, 1.000000000000000000, 0.9510565162951535312, 1.000000000000000000, 0.9510565162951535312, 1.000000000000000000, 0.9510565162951535312, 1.000000000000000000, 0.9510565162951535312, 1.000000000000000000, 0.9510565162951535312, 1.000000000000000000, 0.9510565162951535312, 1.000000000000000000, 0.9510565162951535312, 1.000000000000000000, 0.9510565162951535312, 1.000000000000000000, 0.9510565162951535312, 1.000000000000000000, 0.9510565162951535312, 1.000000000000000000, 0.9510565162951535312, 1.000000000000000000, 0.9510565162951535312, 1.000000000000000000 ) ) 
 REPRESENTATION_ITEM ( '' )  );
#39826=CARTESIAN_POINT ( 'NONE',  ( -5.107581180293630396, 19.93944961101426827, -60.59295307432606847 ) ) ;
#39841=CARTESIAN_POINT ( 'NONE',  ( 5.876318620034919782, 16.56928256419707068, -33.44999999999994600 ) ) ;
#39844=CARTESIAN_POINT ( 'NONE',  ( 2.983759233219601459, 14.30028814967311668, -53.25704692567386900 ) ) ;
#39845=CARTESIAN_POINT ( 'NONE',  ( 0.6505131845895220088, 21.60717860451803674, -71.69999999999997442 ) ) ;
#39852=CARTESIAN_POINT ( 'NONE',  ( 4.318543150850367773, 16.81600996003516357, -54.44999999999996021 ) ) ;
#39854=CARTESIAN_POINT ( 'NONE',  ( 2.121074495332174958, 21.32648900066323350, -34.35704692567387752 ) ) ;
#39855=CARTESIAN_POINT ( 'NONE',  ( -4.001075405444606936, 13.49892459455542060, -70.49999999999997158 ) ) ;
#39858=CARTESIAN_POINT ( 'NONE',  ( -2.017261720333081598, 21.13920729861251857, -36.89295307432605142 ) ) ;
#39863=CARTESIAN_POINT ( 'NONE',  ( -4.294655364005415699, 18.33481159033935626, -27.45704692567386829 ) ) ;
#39870=CARTESIAN_POINT ( 'NONE',  ( -4.206979645153768210, 21.70697964515380107, -41.24999999999995026 ) ) ;
#39887=CARTESIAN_POINT ( 'NONE',  ( -0.9307174358028533767, 23.37631862003491889, -65.54999999999996874 ) ) ;
#39892=CARTESIAN_POINT ( 'NONE',  ( 1.985016409143818272, 21.39581405818570303, -29.84999999999996589 ) ) ;
#39893=CARTESIAN_POINT ( 'NONE',  ( 4.318543150850366885, 16.81600996003516713, -69.44999999999998863 ) ) ;
#39903=CARTESIAN_POINT ( 'NONE',  ( 3.771071394011080269, 15.74153613859503764, -50.09295307432605426 ) ) ;
#39909=CARTESIAN_POINT ( 'NONE',  ( 4.342430937695320736, 16.96683151040971538, -64.94295307432605568 ) ) ;
#39919=CARTESIAN_POINT ( 'NONE',  ( -3.705139346311794313, 19.38786279086902198, -26.09999999999996234 ) ) ;
#39928=CARTESIAN_POINT ( 'NONE',  ( -5.041649132594344884, 20.06884854047834921, -65.09999999999996589 ) ) ;
#39945=CARTESIAN_POINT ( 'NONE',  ( 5.900206406879871857, 16.72010411457162604, -58.94295307432605568 ) ) ;
#39954=CARTESIAN_POINT ( 'NONE',  ( -2.698247469942396837, 22.47571708489507358, -27.89295307432605853 ) ) ;
#39956=CARTESIAN_POINT ( 'NONE',  ( -3.043106805520194413, 14.66227633819065623, -63.00704692567389031 ) ) ;
#39968=CARTESIAN_POINT ( 'NONE',  ( 4.103766977300021601, 21.39838383358913987, -25.50704692567387610 ) ) ;
#39970=CARTESIAN_POINT ( 'NONE',  ( -3.705139346311794313, 19.38786279086902198, -59.09999999999997300 ) ) ;
#39983=CARTESIAN_POINT ( 'NONE',  ( 0.5070733663080689846, 21.62989723985679902, -73.19295307432605568 ) ) ;
#40002=CARTESIAN_POINT ( 'NONE',  ( -1.887862790868997553, 21.20513934631180319, -47.39999999999997016 ) ) ;
#40010=CARTESIAN_POINT ( 'NONE',  ( 0.6505131845895220088, 21.60717860451803674, -62.69999999999996732 ) ) ;
#40013=CARTESIAN_POINT ( 'NONE',  ( -2.837105286290963146, 12.26822144673588255, -59.85704692567387752 ) ) ;
#40014=CARTESIAN_POINT ( 'NONE',  ( -5.876318620034919782, 18.43071743580290089, -46.94999999999996021 ) ) ;
#40027=CARTESIAN_POINT ( 'NONE',  ( -0.7798958854283041253, 23.40020640687986386, -34.05704692567386616 ) ) ;
#40032=CARTESIAN_POINT ( 'NONE',  ( -0.7417250638684240727, 11.88857024925047057, -65.69295307432605568 ) ) ;
#40048=CARTESIAN_POINT ( 'NONE',  ( -0.8851648821498765418, 11.91128888458923285, -37.19999999999996732 ) ) ;
#40051=CARTESIAN_POINT ( 'NONE',  ( -2.983759233219601903, 20.69971185032686023, -54.75704692567386900 ) ) ;
#40052=CARTESIAN_POINT ( 'NONE',  ( 1.887862790868997109, 13.79486065368817194, -69.89999999999996305 ) ) ;
#40060=CARTESIAN_POINT ( 'NONE',  ( 2.940415233664778416, 20.44041523366473712, -53.99999999999996447 ) ) ;
#40063=CARTESIAN_POINT ( 'NONE',  ( 3.639207298612508801, 15.48273827966686866, -35.10704692567387752 ) ) ;
#40074=CARTESIAN_POINT ( 'NONE',  ( -5.852430833189966819, 18.58153898617744915, -69.45704692567387895 ) ) ;
#40080=CARTESIAN_POINT ( 'NONE',  ( -2.568848540478311904, 22.54164913259435465, -41.39999999999996305 ) ) ;
#40096=CARTESIAN_POINT ( 'NONE',  ( -5.041649132594344884, 20.06884854047834921, -65.09999999999996589 ) ) ;
#40101=CARTESIAN_POINT ( 'NONE',  ( -1.985016409143819605, 13.60418594181426855, -34.34999999999995879 ) ) ;
#40102=CARTESIAN_POINT ( 'NONE',  ( 0.6505131845895220088, 21.60717860451803674, -68.69999999999997442 ) ) ;
#40112=CARTESIAN_POINT ( 'NONE',  ( 1.848958322955461808, 21.46513911570817612, -49.34295307432604716 ) ) ;
#40117=CARTESIAN_POINT ( 'NONE',  ( -3.199711850326840246, 20.48375923321962233, -60.74295307432605995 ) ) ;
#40128=CARTESIAN_POINT ( 'NONE',  ( 4.318543150850367773, 16.81600996003516357, -30.44999999999995310 ) ) ;
#40137=CARTESIAN_POINT ( 'NONE',  ( -5.876318620034919782, 18.43071743580290089, -64.94999999999996021 ) ) ;
#40158=CARTESIAN_POINT ( 'NONE',  ( 5.565992480072003978, 18.52860470043125574, -52.79295307432607132 ) ) ;
#40167=CARTESIAN_POINT ( 'NONE',  ( 1.848958322955461808, 21.46513911570817612, -70.34295307432606137 ) ) ;
#40169=CARTESIAN_POINT ( 'NONE',  ( 4.294655364005415699, 16.66518840966061887, -61.95704692567387895 ) ) ;
#40181=CARTESIAN_POINT ( 'NONE',  ( -0.6839900399647736995, 21.81854315085035623, -59.54999999999994742 ) ) ;
#40194=CARTESIAN_POINT ( 'NONE',  ( 4.084459969179292216, 18.29395300287091430, -73.79295307432605000 ) ) ;
#40213=CARTESIAN_POINT ( 'NONE',  ( 3.895814058185739448, 19.48501640914375344, -45.14999999999994884 ) ) ;
#40222=CARTESIAN_POINT ( 'NONE',  ( 4.318543150850367773, 16.81600996003516357, -66.44999999999997442 ) ) ;
#40225=CARTESIAN_POINT ( 'NONE',  ( -5.611429750749524992, 16.75827493613162034, -60.30704692567387326 ) ) ;
#40226=CARTESIAN_POINT ( 'NONE',  ( 4.206979645153768210, 13.29302035484617406, -45.74999999999995737 ) ) ;
#40239=CARTESIAN_POINT ( 'NONE',  ( 5.370428668309080500, 20.06498911391418360, -34.65704692567386758 ) ) ;
#40243=CARTESIAN_POINT ( 'NONE',  ( 5.900206406879871857, 16.72010411457162604, -46.94295307432605568 ) ) ;
#40262=CARTESIAN_POINT ( 'NONE',  ( -5.301103610786608300, 14.79895279989743706, -34.64999999999997016 ) ) ;
#40265=CARTESIAN_POINT ( 'NONE',  ( -2.121074495332175847, 13.67351099933674341, -44.85704692567387752 ) ) ;
#40267=CARTESIAN_POINT ( 'NONE',  ( 3.705139346311793869, 15.61213720913094960, -69.59999999999996589 ) ) ;
#40274=CARTESIAN_POINT ( 'NONE',  ( -3.895814058185739448, 15.51498359085620571, -58.64999999999997016 ) ) ;
#40277=CARTESIAN_POINT ( 'NONE',  ( -0.7939530028709754772, 13.41554003082070246, -32.70704692567387184 ) ) ;
#40278=CARTESIAN_POINT ( 'NONE',  ( -4.206979645153769098, 21.70697964515380107, -74.24999999999997158 ) ) ;
#40287=CARTESIAN_POINT ( 'NONE',  ( 4.975717084895059372, 14.80175253005754143, -65.10704692567387042 ) ) ;
#40293=CARTESIAN_POINT ( 'NONE',  ( -4.206979645153768210, 21.70697964515380107, -32.24999999999996447 ) ) ;
#40312=CARTESIAN_POINT ( 'NONE',  ( 4.206979645153767322, 13.29302035484617051, -63.74999999999997868 ) ) ;
#40317=CARTESIAN_POINT ( 'NONE',  ( -3.895814058185739448, 15.51498359085620571, -31.64999999999995950 ) ) ;
#40318=CARTESIAN_POINT ( 'NONE',  ( -3.705139346311794313, 19.38786279086902198, -65.09999999999996589 ) ) ;
#40331=CARTESIAN_POINT ( 'NONE',  ( 0.5070733663080689846, 21.62989723985679902, -40.19295307432605568 ) ) ;
#40337=CARTESIAN_POINT ( 'NONE',  ( 3.771071394011080269, 15.74153613859503764, -59.09295307432605426 ) ) ;
#40352=CARTESIAN_POINT ( 'NONE',  ( 2.701047200102605572, 22.80110361078655856, -68.84999999999996589 ) ) ;
#40372=CARTESIAN_POINT ( 'NONE',  ( 0.7417250638684235176, 23.11142975074950101, -52.19295307432606279 ) ) ;
#40380=CARTESIAN_POINT ( 'NONE',  ( 0.5070733663080689846, 21.62989723985679902, -61.19295307432605568 ) ) ;
#40382=CARTESIAN_POINT ( 'NONE',  ( -1.758463861404912842, 21.27107139401109137, -54.90704692567386758 ) ) ;
#40394=CARTESIAN_POINT ( 'NONE',  ( -3.091735541773221296, 20.59173554177323950, -56.24999999999995026 ) ) ;
#40404=CARTESIAN_POINT ( 'NONE',  ( -3.199711850326840246, 20.48375923321962233, -75.74295307432603863 ) ) ;
#40419=CARTESIAN_POINT ( 'NONE',  ( -2.940415233664778860, 14.55958476633523802, -43.49999999999997158 ) ) ;
#40422=CARTESIAN_POINT ( 'NONE',  ( 1.887862790868997109, 13.79486065368817194, -30.89999999999996305 ) ) ;
#40431=CARTESIAN_POINT ( 'NONE',  ( -1.985016409143819605, 13.60418594181426855, -61.34999999999996589 ) ) ;
#40433=CARTESIAN_POINT ( 'NONE',  ( -4.103766977300021601, 13.60161616641083704, -57.00704692567387610 ) ) ;
#40434=CARTESIAN_POINT ( 'NONE',  ( -0.9307174358028534877, 23.37631862003491889, -35.54999999999995453 ) ) ;
#40442=AXIS2_PLACEMENT_3D ( 'NONE', #11131, #24112, #36650 ) ;
#40451=CARTESIAN_POINT ( 'NONE',  ( -4.975717084895059372, 20.19824746994243370, -33.60704692567387042 ) ) ;
#40456=CARTESIAN_POINT ( 'NONE',  ( -5.565992480072003978, 16.47139529956871229, -51.29295307432606421 ) ) ;
#40473=CARTESIAN_POINT ( 'NONE',  ( -5.565992480072003978, 16.47139529956871229, -69.29295307432606421 ) ) ;
#40476=CARTESIAN_POINT ( 'NONE',  ( -2.121074495332175847, 13.67351099933674341, -47.85704692567386331 ) ) ;
#40477=CARTESIAN_POINT ( 'NONE',  ( -3.091735541773221296, 20.59173554177323950, -62.24999999999995737 ) ) ;
#40484=CARTESIAN_POINT ( 'NONE',  ( -4.107178604518053611, 16.84948681541050775, -49.79999999999996874 ) ) ;
#40488=CARTESIAN_POINT ( 'NONE',  ( -3.639207298612509689, 19.51726172033310647, -36.60704692567387752 ) ) ;
#40489=CARTESIAN_POINT ( 'NONE',  ( 5.876318620034919782, 16.56928256419707068, -60.44999999999996732 ) ) ;
#40498=CARTESIAN_POINT ( 'NONE',  ( 5.611429750749524992, 18.24172506386835479, -64.80704692567387326 ) ) ;
#40504=CARTESIAN_POINT ( 'NONE',  ( -5.041649132594344884, 20.06884854047834921, -29.09999999999996589 ) ) ;
#40521=CARTESIAN_POINT ( 'NONE',  ( 5.041649132594343996, 14.93115145952162415, -54.59999999999996589 ) ) ;
#40525=CARTESIAN_POINT ( 'NONE',  ( -3.639207298612509689, 19.51726172033310647, -72.60704692567387042 ) ) ;
#40526=CARTESIAN_POINT ( 'NONE',  ( -1.985016409143819605, 13.60418594181426855, -70.34999999999995168 ) ) ;
#40537=CARTESIAN_POINT ( 'NONE',  ( -2.837723661809363751, 14.45689319447982335, -38.99295307432604574 ) ) ;
#40540=CARTESIAN_POINT ( 'NONE',  ( 2.837723661809363307, 20.54310680552015356, -55.49295307432605995 ) ) ;
#40556=CARTESIAN_POINT ( 'NONE',  ( 0.8851648821498760977, 23.08871111541074228, -59.69999999999996732 ) ) ;
#40573=CARTESIAN_POINT ( 'NONE',  ( 5.231778553264135212, 20.33710528629089254, -55.64295307432606563 ) ) ;
#40581=CARTESIAN_POINT ( 'NONE',  ( 3.771071394011080269, 15.74153613859503764, -62.09295307432606847 ) ) ;
#40583=CARTESIAN_POINT ( 'NONE',  ( 1.758463861404912620, 13.72892860598888731, -56.40704692567388179 ) ) ;
#40596=CARTESIAN_POINT ( 'NONE',  ( -1.985016409143819605, 13.60418594181426855, -43.34999999999994458 ) ) ;
#40606=CARTESIAN_POINT ( 'NONE',  ( 3.826489000663266360, 19.62107449533211678, -70.64295307432605853 ) ) ;
#40617=CARTESIAN_POINT ( 'NONE',  ( 0.6839900399647732554, 13.18145684914961357, -43.04999999999996163 ) ) ;
#40623=CARTESIAN_POINT ( 'NONE',  ( -4.107178604518053611, 16.84948681541050775, -37.79999999999996874 ) ) ;
#40632=CARTESIAN_POINT ( 'NONE',  ( -3.091735541773221296, 20.59173554177323950, -53.24999999999996447 ) ) ;
#40634=CARTESIAN_POINT ( 'NONE',  ( -4.099003336600151925, 21.81495595370741469, -45.75704692567386900 ) ) ;
#40635=CARTESIAN_POINT ( 'NONE',  ( 2.701047200102605128, 22.80110361078656211, -38.84999999999996589 ) ) ;
#40638=CARTESIAN_POINT ( 'NONE',  ( -3.895814058185739448, 15.51498359085620571, -70.64999999999996305 ) ) ;
#40648=CARTESIAN_POINT ( 'NONE',  ( 1.028604700431328567, 23.06599248007198355, -34.20704692567387184 ) ) ;
#40654=CARTESIAN_POINT ( 'NONE',  ( -1.081538986177402961, 23.35243083318996327, -49.04295307432606421 ) ) ;
#40669=CARTESIAN_POINT ( 'NONE',  ( -4.001075405444606936, 13.49892459455542060, -25.49999999999996803 ) ) ;
#40672=CARTESIAN_POINT ( 'NONE',  ( -3.043106805520194413, 14.66227633819065623, -42.00704692567387610 ) ) ;
#40674=CARTESIAN_POINT ( 'NONE',  ( 1.985016409143818272, 21.39581405818570303, -32.84999999999996589 ) ) ;
#40675=CARTESIAN_POINT ( 'NONE',  ( 2.940415233664778416, 20.44041523366473712, -68.99999999999995737 ) ) ;
#40687=CARTESIAN_POINT ( 'NONE',  ( 1.028604700431328567, 23.06599248007198355, -73.20704692567387895 ) ) ;
#40688=CARTESIAN_POINT ( 'NONE',  ( -5.588711115410763597, 16.61483511785016987, -67.79999999999996874 ) ) ;
#40698=CARTESIAN_POINT ( 'NONE',  ( -5.852430833189966819, 18.58153898617744915, -60.45704692567387895 ) ) ;
#40702=CARTESIAN_POINT ( 'NONE',  ( 0.8851648821498760977, 23.08871111541074228, -29.69999999999996376 ) ) ;
#40719=CARTESIAN_POINT ( 'NONE',  ( 5.876318620034919782, 16.56928256419707068, -51.44999999999997442 ) ) ;
#40723=CARTESIAN_POINT ( 'NONE',  ( 1.758463861404912620, 13.72892860598888731, -71.40704692567388179 ) ) ;
#40724=CARTESIAN_POINT ( 'NONE',  ( 1.887862790868997109, 13.79486065368817194, -57.89999999999996305 ) ) ;
#40737=CARTESIAN_POINT ( 'NONE',  ( -4.084459969179292216, 16.70604699712905372, -33.29295307432605711 ) ) ;
#40741=CARTESIAN_POINT ( 'NONE',  ( -0.5070733663080690956, 13.37010276014318144, -50.69295307432606279 ) ) ;
#40757=CARTESIAN_POINT ( 'NONE',  ( 4.001075405444606048, 21.50107540544455276, -56.99999999999996447 ) ) ;
#40781=CARTESIAN_POINT ( 'NONE',  ( 1.081538986177402295, 11.64756916681001186, -47.54295307432606421 ) ) ;
#40790=CARTESIAN_POINT ( 'NONE',  ( -0.5070733663080690956, 13.37010276014318144, -68.69295307432605568 ) ) ;
#40803=CARTESIAN_POINT ( 'NONE',  ( -0.6505131845895224529, 13.39282139548194195, -46.19999999999996021 ) ) ;
#40818=CARTESIAN_POINT ( 'NONE',  ( -3.826489000663265472, 15.37892550466785480, -69.14295307432605853 ) ) ;
#40830=CARTESIAN_POINT ( 'NONE',  ( 0.6839900399647732554, 13.18145684914961357, -34.04999999999996163 ) ) ;
#40834=CARTESIAN_POINT ( 'NONE',  ( -3.705139346311794313, 19.38786279086902198, -35.09999999999996589 ) ) ;
#40842=CARTESIAN_POINT ( 'NONE',  ( 4.107178604518054499, 18.15051318458946383, -51.29999999999996874 ) ) ;
#40844=CARTESIAN_POINT ( 'NONE',  ( 1.028604700431328567, 23.06599248007198355, -46.20704692567387184 ) ) ;
#40845=CARTESIAN_POINT ( 'NONE',  ( -0.9307174358028534877, 23.37631862003491889, -32.54999999999996163 ) ) ;
#40848=CARTESIAN_POINT ( 'NONE',  ( -3.705139346311794313, 19.38786279086902198, -74.09999999999996589 ) ) ;
#40858=CARTESIAN_POINT ( 'NONE',  ( 1.028604700431328567, 23.06599248007198355, -40.20704692567387184 ) ) ;
#40863=CARTESIAN_POINT ( 'NONE',  ( -5.231778553264134324, 14.66289471370907727, -48.14295307432606563 ) ) ;
#40881=CARTESIAN_POINT ( 'NONE',  ( 1.081538986177402295, 11.64756916681001186, -74.54295307432605000 ) ) ;
#40885=CARTESIAN_POINT ( 'NONE',  ( -2.983759233219601903, 20.69971185032686023, -45.75704692567386900 ) ) ;
#40886=CARTESIAN_POINT ( 'NONE',  ( 3.091735541773220852, 14.40826445822673563, -33.74999999999996447 ) ) ;
#40888=CARTESIAN_POINT ( 'NONE',  ( 3.705139346311793869, 15.61213720913094960, -60.59999999999996589 ) ) ;
#40897=CARTESIAN_POINT ( 'NONE',  ( -4.103766977300021601, 13.60161616641083704, -72.00704692567386189 ) ) ;
#40898=CARTESIAN_POINT ( 'NONE',  ( -0.9307174358028534877, 23.37631862003491889, -65.54999999999996874 ) ) ;
#40908=CARTESIAN_POINT ( 'NONE',  ( -5.852430833189966819, 18.58153898617744915, -63.45704692567386473 ) ) ;
#40913=CARTESIAN_POINT ( 'NONE',  ( 0.7417250638684235176, 23.11142975074950101, -76.19295307432606990 ) ) ;
#40933=CARTESIAN_POINT ( 'NONE',  ( 0.9307174358028528216, 11.62368137996505801, -52.04999999999997584 ) ) ;
#40937=CARTESIAN_POINT ( 'NONE',  ( -2.983759233219601903, 20.69971185032686023, -69.75704692567386189 ) ) ;
#40938=CARTESIAN_POINT ( 'NONE',  ( -0.6505131845895224529, 13.39282139548194195, -61.19999999999996732 ) ) ;
#40947=CARTESIAN_POINT ( 'NONE',  ( 0.6839900399647733664, 13.18145684914961357, -73.04999999999998295 ) ) ;
#40952=CARTESIAN_POINT ( 'NONE',  ( 2.837723661809363307, 20.54310680552015356, -34.49295307432605995 ) ) ;
#40956=CARTESIAN_POINT ( 'NONE',  ( 2.017261720333081598, 13.86079270138745834, -53.39295307432605853 ) ) ;
#40971=CARTESIAN_POINT ( 'NONE',  ( -4.001075405444606936, 13.49892459455542060, -61.49999999999997158 ) ) ;
#40995=CARTESIAN_POINT ( 'NONE',  ( 3.898383833589191383, 21.60376697729997275, -46.49295307432606705 ) ) ;
#41003=CARTESIAN_POINT ( 'NONE',  ( -2.837723661809363751, 14.45689319447982335, -62.99295307432606705 ) ) ;
#41018=CARTESIAN_POINT ( 'NONE',  ( 0.6839900399647733664, 13.18145684914961357, -46.04999999999996163 ) ) ;
#41043=CARTESIAN_POINT ( 'NONE',  ( 0.6505131845895220088, 21.60717860451803674, -41.69999999999996732 ) ) ;
#41047=CARTESIAN_POINT ( 'NONE',  ( -1.985016409143819605, 13.60418594181426855, -37.34999999999994458 ) ) ;
#41056=CARTESIAN_POINT ( 'NONE',  ( -1.887862790868997553, 21.20513934631180319, -53.39999999999997016 ) ) ;
#41058=CARTESIAN_POINT ( 'NONE',  ( -5.611429750749524992, 16.75827493613162034, -45.30704692567388037 ) ) ;
#41059=CARTESIAN_POINT ( 'NONE',  ( -2.568848540478311904, 22.54164913259435465, -32.39999999999996305 ) ) ;
#41061=CARTESIAN_POINT ( 'NONE',  ( -4.342430937695320736, 18.03316848959025620, -30.44295307432605213 ) ) ;
#41075=CARTESIAN_POINT ( 'NONE',  ( -2.837105286290963146, 12.26822144673588255, -26.85704692567387397 ) ) ;
#41082=CARTESIAN_POINT ( 'NONE',  ( 5.900206406879871857, 16.72010411457162604, -49.94295307432606279 ) ) ;
#41099=CARTESIAN_POINT ( 'NONE',  ( 1.081538986177402295, 11.64756916681001186, -71.54295307432605000 ) ) ;
#41104=CARTESIAN_POINT ( 'NONE',  ( -2.983759233219601903, 20.69971185032686023, -39.75704692567386900 ) ) ;
#41105=CARTESIAN_POINT ( 'NONE',  ( 0.6505131845895220088, 21.60717860451803674, -35.69999999999996732 ) ) ;
#41107=CARTESIAN_POINT ( 'NONE',  ( -1.985016409143819605, 13.60418594181426855, -61.34999999999996589 ) ) ;
#41118=CARTESIAN_POINT ( 'NONE',  ( -2.837105286290963146, 12.26822144673588255, -71.85704692567388463 ) ) ;
#41119=CARTESIAN_POINT ( 'NONE',  ( -2.701047200102606460, 12.19889638921340591, -67.34999999999996589 ) ) ;
#41132=CARTESIAN_POINT ( 'NONE',  ( 1.028604700431328567, 23.06599248007198355, -67.20704692567387895 ) ) ;
#41135=CARTESIAN_POINT ( 'NONE',  ( 5.588711115410763597, 18.38516488214980882, -30.29999999999996518 ) ) ;
#41153=CARTESIAN_POINT ( 'NONE',  ( 4.001075405444606048, 21.50107540544455276, -50.99999999999997158 ) ) ;
#41157=CARTESIAN_POINT ( 'NONE',  ( -1.887862790868997553, 21.20513934631180319, -26.39999999999996660 ) ) ;
#41158=CARTESIAN_POINT ( 'NONE',  ( -0.6839900399647738105, 21.81854315085035623, -59.54999999999995453 ) ) ;
#41164=CARTESIAN_POINT ( 'NONE',  ( -3.895814058185739448, 15.51498359085620571, -70.64999999999996305 ) ) ;
#41169=CARTESIAN_POINT ( 'NONE',  ( 4.342430937695320736, 16.96683151040971538, -34.94295307432605568 ) ) ;
#41172=CARTESIAN_POINT ( 'NONE',  ( -2.017261720333081598, 21.13920729861251857, -42.89295307432605853 ) ) ;
#41188=CARTESIAN_POINT ( 'NONE',  ( -2.701047200102606016, 12.19889638921340413, -55.34999999999997300 ) ) ;
#41211=CARTESIAN_POINT ( 'NONE',  ( 5.107581180293630396, 15.06055038898570686, -50.09295307432605426 ) ) ;
#41218=CARTESIAN_POINT ( 'NONE',  ( 1.848958322955461808, 21.46513911570817612, -64.34295307432606137 ) ) ;
#41232=CARTESIAN_POINT ( 'NONE',  ( 1.985016409143818272, 21.39581405818570303, -44.84999999999996589 ) ) ;
#41254=CARTESIAN_POINT ( 'NONE',  ( 4.107178604518054499, 18.15051318458946383, -30.29999999999996518 ) ) ;
#41260=CARTESIAN_POINT ( 'NONE',  ( 1.985016409143818272, 21.39581405818570303, -35.84999999999996589 ) ) ;
#41269=CARTESIAN_POINT ( 'NONE',  ( 2.940415233664778416, 20.44041523366473712, -56.99999999999996447 ) ) ;
#41271=CARTESIAN_POINT ( 'NONE',  ( -5.852430833189966819, 18.58153898617744915, -45.45704692567387184 ) ) ;
#41272=CARTESIAN_POINT ( 'NONE',  ( 0.8851648821498760977, 23.08871111541074228, -32.69999999999996732 ) ) ;
#41274=CARTESIAN_POINT ( 'NONE',  ( -3.826489000663265472, 15.37892550466785480, -30.14295307432606208 ) ) ;
#41284=CARTESIAN_POINT ( 'NONE',  ( -5.852430833189966819, 18.58153898617744915, -27.45704692567386829 ) ) ;
#41289=CARTESIAN_POINT ( 'NONE',  ( -2.564989113914250662, 12.12957133169093282, -41.84295307432606137 ) ) ;
#41307=SHAPE_REPRESENTATION_RELATIONSHIP ( 'NONE' , 'NONE' ,  #1913, #6131 ) ;
#41308=CARTESIAN_POINT ( 'NONE',  ( 5.900206406879871857, 16.72010411457162604, -70.94295307432606990 ) ) ;
#41314=CARTESIAN_POINT ( 'NONE',  ( 3.091735541773220852, 14.40826445822673563, -36.74999999999994316 ) ) ;
#41315=CARTESIAN_POINT ( 'NONE',  ( -1.985016409143819605, 13.60418594181426855, -64.34999999999996589 ) ) ;
#41324=CARTESIAN_POINT ( 'NONE',  ( 4.099003336600150149, 13.18504404629255689, -71.25704692567387610 ) ) ;
#41325=CARTESIAN_POINT ( 'NONE',  ( -0.8851648821498765418, 11.91128888458923285, -67.19999999999997442 ) ) ;
#41338=CARTESIAN_POINT ( 'NONE',  ( -5.370428668309080500, 14.93501088608579153, -54.15704692567387468 ) ) ;
#41341=CARTESIAN_POINT ( 'NONE',  ( -5.565992480072003978, 16.47139529956871229, -75.29295307432605000 ) ) ;
#41358=CARTESIAN_POINT ( 'NONE',  ( -5.301103610786608300, 14.79895279989743706, -52.64999999999997016 ) ) ;
#41363=CARTESIAN_POINT ( 'NONE',  ( -4.129897239856814117, 16.99292663369196177, -60.30704692567387326 ) ) ;
#41364=CARTESIAN_POINT ( 'NONE',  ( 3.705139346311793869, 15.61213720913094960, -60.59999999999996589 ) ) ;
#41371=CARTESIAN_POINT ( 'NONE',  ( 0.6839900399647733664, 13.18145684914961357, -70.04999999999996874 ) ) ;
#41373=CARTESIAN_POINT ( 'NONE',  ( 3.965139115708213868, 19.34895832295540430, -52.65704692567388179 ) ) ;
#41376=CARTESIAN_POINT ( 'NONE',  ( 2.837723661809363307, 20.54310680552015356, -28.49295307432605995 ) ) ;
#41379=CARTESIAN_POINT ( 'NONE',  ( 4.342430937695320736, 16.96683151040971538, -43.94295307432605568 ) ) ;
#41397=CARTESIAN_POINT ( 'NONE',  ( 0.9307174358028528216, 11.62368137996505801, -58.04999999999996874 ) ) ;
#41417=CARTESIAN_POINT ( 'NONE',  ( -4.314955953707389824, 21.59900333660018390, -45.74295307432605995 ) ) ;
#41426=CARTESIAN_POINT ( 'NONE',  ( -3.826489000663265472, 15.37892550466785480, -54.14295307432606563 ) ) ;
#41440=CARTESIAN_POINT ( 'NONE',  ( -4.107178604518053611, 16.84948681541050775, -43.79999999999996163 ) ) ;
#41466=CARTESIAN_POINT ( 'NONE',  ( 4.318543150850366885, 16.81600996003516713, -33.44999999999996021 ) ) ;
#41472=CARTESIAN_POINT ( 'NONE',  ( -4.294655364005415699, 18.33481159033935626, -69.45704692567387895 ) ) ;
#41482=CARTESIAN_POINT ( 'NONE',  ( -3.705139346311794313, 19.38786279086902198, -56.09999999999996589 ) ) ;
#41485=CARTESIAN_POINT ( 'NONE',  ( 4.099003336600150149, 13.18504404629255689, -50.25704692567386900 ) ) ;
#41486=CARTESIAN_POINT ( 'NONE',  ( -5.041649132594344884, 20.06884854047834921, -26.09999999999996234 ) ) ;
#41487=CARTESIAN_POINT ( 'NONE',  ( 0.5070733663080689846, 21.62989723985679902, -28.19295307432605568 ) ) ;
#41497=CARTESIAN_POINT ( 'NONE',  ( -2.568848540478311904, 22.54164913259435465, -74.39999999999996305 ) ) ;
#41502=CARTESIAN_POINT ( 'NONE',  ( 3.898383833589191383, 21.60376697729997275, -43.49295307432606705 ) ) ;
#41521=CARTESIAN_POINT ( 'NONE',  ( 5.900206406879871857, 16.72010411457162604, -64.94295307432605568 ) ) ;
#41526=CARTESIAN_POINT ( 'NONE',  ( -4.318543150850367773, 18.18399003996480801, -34.94999999999996732 ) ) ;
#41527=CARTESIAN_POINT ( 'NONE',  ( 1.985016409143818272, 21.39581405818570303, -56.84999999999995879 ) ) ;
#41537=CARTESIAN_POINT ( 'NONE',  ( -0.7798958854283041253, 23.40020640687986386, -73.05704692567387326 ) ) ;
#41538=CARTESIAN_POINT ( 'NONE',  ( -2.701047200102606460, 12.19889638921340591, -55.34999999999996589 ) ) ;
#41550=CARTESIAN_POINT ( 'NONE',  ( 5.370428668309080500, 20.06498911391418360, -52.65704692567388179 ) ) ;
#41553=CARTESIAN_POINT ( 'NONE',  ( -3.898383833589191827, 13.39623302270000771, -65.99295307432606705 ) ) ;
#41570=CARTESIAN_POINT ( 'NONE',  ( 2.701047200102605572, 22.80110361078655856, -41.84999999999995879 ) ) ;
#41574=CARTESIAN_POINT ( 'NONE',  ( -2.121074495332175847, 13.67351099933674341, -62.85704692567387042 ) ) ;
#41575=CARTESIAN_POINT ( 'NONE',  ( -4.318543150850366885, 18.18399003996480801, -61.94999999999996732 ) ) ;
#41583=CARTESIAN_POINT ( 'NONE',  ( -1.887862790868997553, 21.20513934631180319, -62.39999999999997016 ) ) ;
#41585=CARTESIAN_POINT ( 'NONE',  ( -3.043106805520194413, 14.66227633819065623, -57.00704692567387610 ) ) ;
#41588=CARTESIAN_POINT ( 'NONE',  ( 1.848958322955461808, 21.46513911570817612, -31.34295307432605782 ) ) ;
#41591=CARTESIAN_POINT ( 'NONE',  ( 4.342430937695320736, 16.96683151040971538, -46.94295307432605568 ) ) ;
#41607=CARTESIAN_POINT ( 'NONE',  ( -5.301103610786608300, 14.79895279989743706, -46.64999999999994884 ) ) ;
#41627=CARTESIAN_POINT ( 'NONE',  ( 1.985016409143818272, 21.39581405818570303, -47.84999999999994458 ) ) ;
#41630=CARTESIAN_POINT ( 'NONE',  ( -5.900206406879871857, 18.27989588542834554, -48.44295307432605568 ) ) ;
#41640=CARTESIAN_POINT ( 'NONE',  ( -0.8348115903393239501, 21.79465536400541126, -52.04295307432606421 ) ) ;
#41653=CARTESIAN_POINT ( 'NONE',  ( -4.318543150850367773, 18.18399003996480801, -40.94999999999996732 ) ) ;
#41678=CARTESIAN_POINT ( 'NONE',  ( 3.895814058185739892, 19.48501640914376054, -33.14999999999996305 ) ) ;
#41681=CARTESIAN_POINT ( 'NONE',  ( -2.564989113914250662, 12.12957133169093282, -38.84295307432606137 ) ) ;
#41682=CARTESIAN_POINT ( 'NONE',  ( 1.985016409143818272, 21.39581405818570303, -29.84999999999996589 ) ) ;
#41690=CARTESIAN_POINT ( 'NONE',  ( 3.705139346311793869, 15.61213720913094960, -45.59999999999996589 ) ) ;
#41693=CARTESIAN_POINT ( 'NONE',  ( 5.611429750749524992, 18.24172506386835479, -40.80704692567388037 ) ) ;
#41694=CARTESIAN_POINT ( 'NONE',  ( 5.876318620034919782, 16.56928256419707068, -27.44999999999996376 ) ) ;
#41696=CARTESIAN_POINT ( 'NONE',  ( -0.6505131845895224529, 13.39282139548194195, -61.19999999999996732 ) ) ;
#41706=CARTESIAN_POINT ( 'NONE',  ( 0.9307174358028528216, 11.62368137996505801, -73.04999999999998295 ) ) ;
#41711=CARTESIAN_POINT ( 'NONE',  ( 1.081538986177402295, 11.64756916681001186, -38.54295307432605000 ) ) ;
#41728=CARTESIAN_POINT ( 'NONE',  ( 5.900206406879871857, 16.72010411457162604, -61.94295307432605568 ) ) ;
#41734=CARTESIAN_POINT ( 'NONE',  ( -0.6505131845895224529, 13.39282139548194195, -28.19999999999996732 ) ) ;
#41735=CARTESIAN_POINT ( 'NONE',  ( -4.107178604518053611, 16.84948681541050775, -55.79999999999996874 ) ) ;
#41747=CARTESIAN_POINT ( 'NONE',  ( 5.370428668309080500, 20.06498911391418360, -70.65704692567386758 ) ) ;
#41748=CARTESIAN_POINT ( 'NONE',  ( -2.568848540478311904, 22.54164913259435465, -53.39999999999997016 ) ) ;
#41761=CARTESIAN_POINT ( 'NONE',  ( -1.028604700431329233, 11.93400751992799513, -56.70704692567387184 ) ) ;
#41764=CARTESIAN_POINT ( 'NONE',  ( -5.231778553264134324, 14.66289471370907727, -75.14295307432605853 ) ) ;
#41783=CARTESIAN_POINT ( 'NONE',  ( 0.8851648821498760977, 23.08871111541074228, -38.69999999999996021 ) ) ;
#41788=CARTESIAN_POINT ( 'NONE',  ( -3.965139115708213868, 15.65104167704456906, -60.15704692567387468 ) ) ;
#41790=CARTESIAN_POINT ( 'NONE',  ( -3.895814058185739892, 15.51498359085620748, -52.64999999999997016 ) ) ;
#41799=CARTESIAN_POINT ( 'NONE',  ( 3.895814058185739448, 19.48501640914375344, -63.14999999999997016 ) ) ;
#41801=CARTESIAN_POINT ( 'NONE',  ( 3.965139115708213868, 19.34895832295540430, -40.65704692567387468 ) ) ;
#41804=CARTESIAN_POINT ( 'NONE',  ( 0.5070733663080689846, 21.62989723985679902, -31.19295307432605568 ) ) ;
#41807=CARTESIAN_POINT ( 'NONE',  ( -3.199711850326840246, 20.48375923321962233, -48.74295307432605284 ) ) ;
#41824=CARTESIAN_POINT ( 'NONE',  ( -5.876318620034919782, 18.43071743580290089, -46.94999999999996021 ) ) ;
#41838=CARTESIAN_POINT ( 'NONE',  ( -2.701047200102606016, 12.19889638921340413, -67.34999999999996589 ) ) ;
#41844=CARTESIAN_POINT ( 'NONE',  ( -3.091735541773221296, 20.59173554177323950, -44.24999999999997868 ) ) ;
#41845=CARTESIAN_POINT ( 'NONE',  ( 3.091735541773220852, 14.40826445822673740, -72.74999999999995737 ) ) ;
#41856=CARTESIAN_POINT ( 'NONE',  ( -0.5070733663080690956, 13.37010276014318144, -53.69295307432606279 ) ) ;
#41871=CARTESIAN_POINT ( 'NONE',  ( -3.091735541773221296, 20.59173554177323950, -38.24999999999996447 ) ) ;
#41896=CARTESIAN_POINT ( 'NONE',  ( 2.121074495332174958, 21.32648900066323350, -37.35704692567387752 ) ) ;
#41897=CARTESIAN_POINT ( 'NONE',  ( 3.895814058185739892, 19.48501640914376054, -27.14999999999996305 ) ) ;
#41901=CARTESIAN_POINT ( 'NONE',  ( -5.565992480072003978, 16.47139529956871229, -30.29295307432605355 ) ) ;
#41902=CARTESIAN_POINT ( 'NONE',  ( 4.107178604518054499, 18.15051318458946383, -30.29999999999996518 ) ) ;
#41909=CARTESIAN_POINT ( 'NONE',  ( 4.318543150850367773, 16.81600996003516357, -45.44999999999996021 ) ) ;
#41912=CARTESIAN_POINT ( 'NONE',  ( -5.852430833189966819, 18.58153898617744915, -39.45704692567387184 ) ) ;
#41913=CARTESIAN_POINT ( 'NONE',  ( 5.876318620034919782, 16.56928256419707068, -30.44999999999996021 ) ) ;
#41914=CARTESIAN_POINT ( 'NONE',  ( 4.107178604518054499, 18.15051318458946383, -66.29999999999996874 ) ) ;
#41927=CARTESIAN_POINT ( 'NONE',  ( -5.231778553264134324, 14.66289471370907727, -42.14295307432605142 ) ) ;
#41941=CARTESIAN_POINT ( 'NONE',  ( -2.698247469942396837, 22.47571708489507358, -63.89295307432605853 ) ) ;
#41946=CARTESIAN_POINT ( 'NONE',  ( -1.985016409143819605, 13.60418594181426855, -28.34999999999995524 ) ) ;
#41947=CARTESIAN_POINT ( 'NONE',  ( -1.887862790868997553, 21.20513934631180319, -59.39999999999997016 ) ) ;
#41958=CARTESIAN_POINT ( 'NONE',  ( -5.370428668309080500, 14.93501088608579153, -69.15704692567386758 ) ) ;
#41959=CARTESIAN_POINT ( 'NONE',  ( 2.568848540478311460, 12.45835086740561692, -54.89999999999996305 ) ) ;
#41973=CARTESIAN_POINT ( 'NONE',  ( -5.370428668309080500, 14.93501088608579153, -57.15704692567387468 ) ) ;
#41976=CARTESIAN_POINT ( 'NONE',  ( 5.231778553264135212, 20.33710528629089254, -67.64295307432605853 ) ) ;
#41994=CARTESIAN_POINT ( 'NONE',  ( 5.588711115410763597, 18.38516488214980882, -42.29999999999996874 ) ) ;
#41998=CARTESIAN_POINT ( 'NONE',  ( 3.639207298612508801, 15.48273827966686866, -59.10704692567387752 ) ) ;
#41999=CARTESIAN_POINT ( 'NONE',  ( -2.940415233664778860, 14.55958476633523802, -49.49999999999996447 ) ) ;
#42008=CARTESIAN_POINT ( 'NONE',  ( -1.887862790868997553, 21.20513934631180319, -65.39999999999997726 ) ) ;
#42010=CARTESIAN_POINT ( 'NONE',  ( -3.639207298612509689, 19.51726172033310647, -42.60704692567387752 ) ) ;
#42015=CARTESIAN_POINT ( 'NONE',  ( -0.8348115903393239501, 21.79465536400541126, -49.04295307432606421 ) ) ;
#42030=CARTESIAN_POINT ( 'NONE',  ( 0.9307174358028528216, 11.62368137996505801, -46.04999999999996163 ) ) ;
#42046=CARTESIAN_POINT ( 'NONE',  ( 2.568848540478311460, 12.45835086740561692, -69.89999999999996305 ) ) ;
#42051=CARTESIAN_POINT ( 'NONE',  ( -0.6839900399647736995, 21.81854315085035623, -44.54999999999994742 ) ) ;
#42059=CARTESIAN_POINT ( 'NONE',  ( 3.771071394011080269, 15.74153613859503764, -53.09295307432605426 ) ) ;
#42075=CARTESIAN_POINT ( 'NONE',  ( 2.940415233664778416, 20.44041523366473712, -32.99999999999996447 ) ) ;
#42102=CARTESIAN_POINT ( 'NONE',  ( 2.121074495332174958, 21.32648900066323350, -34.35704692567387752 ) ) ;
#42103=CARTESIAN_POINT ( 'NONE',  ( -3.895814058185739892, 15.51498359085620748, -28.64999999999995950 ) ) ;
#42106=CARTESIAN_POINT ( 'NONE',  ( -5.900206406879871857, 18.27989588542834554, -33.44295307432605568 ) ) ;
#42107=CARTESIAN_POINT ( 'NONE',  ( 3.895814058185739448, 19.48501640914375344, -27.14999999999995595 ) ) ;
#42114=CARTESIAN_POINT ( 'NONE',  ( -4.318543150850367773, 18.18399003996480801, -43.94999999999995310 ) ) ;
#42146=COLOUR_RGB('Grey',0.48,0.52,0.57);
#42147=FILL_AREA_STYLE_COLOUR('',#42146);
#42148=FILL_AREA_STYLE('',(#42147));
#42149=SURFACE_STYLE_FILL_AREA(#42148);
#42150=SURFACE_SIDE_STYLE('',(#42149));
#42151=SURFACE_STYLE_USAGE(.BOTH.,#42150);
#42152=PRESENTATION_STYLE_ASSIGNMENT((#42151));
ENDSEC;
END-ISO-10303-21;
